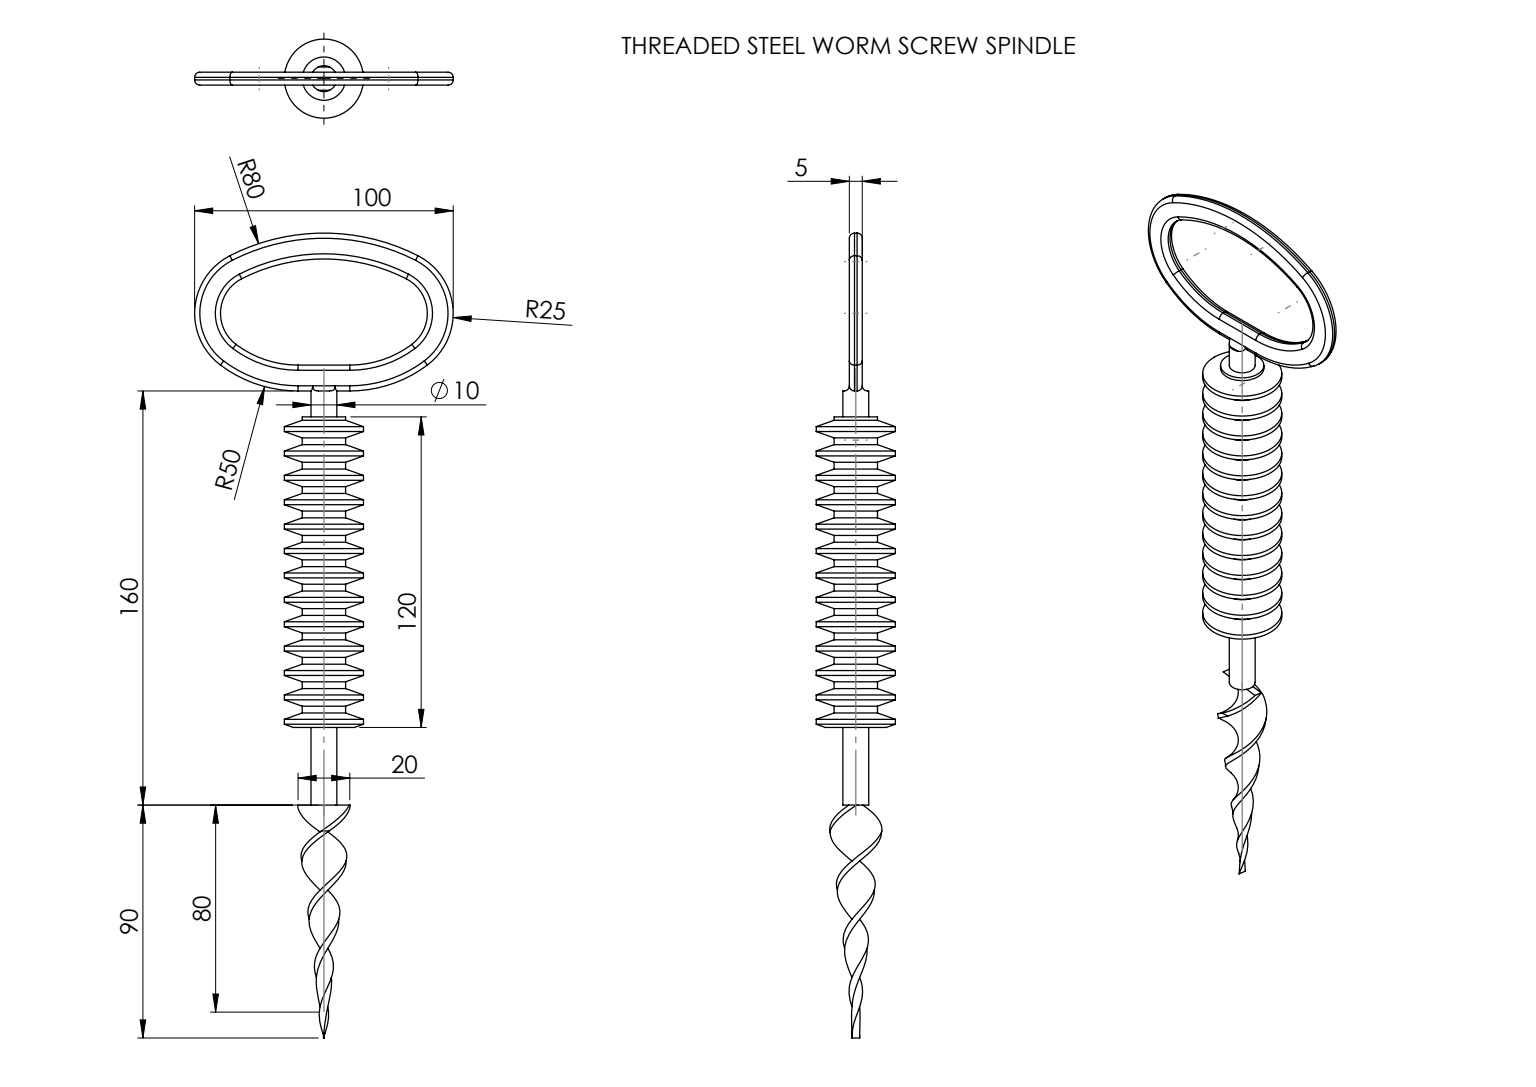
ISO-10303-21;
HEADER;
FILE_DESCRIPTION (('STEP AP214'),
    '1' );
FILE_NAME ('Threaded Steel Worm Screw Spindle.step',
    '2026-10-08T14:03:35',
    ( '' ),
    ( '' ),
    'SwSTEP 2.0',
    'SolidWorks 2026',
    '' );
FILE_SCHEMA (( 'AUTOMOTIVE_DESIGN' ));
ENDSEC;

DATA;
#7=AXIS2_PLACEMENT_3D ( 'NONE', #7492, #359, #1391 ) ;
#9=ORIENTED_EDGE ( 'NONE', *, *, #2863, .F. ) ;
#10=CYLINDRICAL_SURFACE ( 'NONE', #6059, 5.000000000000000000 ) ;
#12=DIRECTION ( 'NONE',  ( -1.000000000000000000, 0.000000000000000000, 0.000000000000000000 ) ) ;
#16=CARTESIAN_POINT ( 'NONE',  ( -12.99553232110413248, 67.62342244460847951, -25.99106464220826851 ) ) ;
#19=CARTESIAN_POINT ( 'NONE',  ( 4.330127018922190985, 92.00000000000000000, -2.500000000000000000 ) ) ;
#20=CARTESIAN_POINT ( 'NONE',  ( 10.69381717166375623, 25.55944687211528077, 0.000000000000000000 ) ) ;
#21=ADVANCED_FACE ( 'NONE', ( #11217 ), #12542, .T. ) ;
#26=EDGE_CURVE ( 'NONE', #11146, #5183, #4908, .T. ) ;
#27=EDGE_CURVE ( 'NONE', #5877, #10681, #5933, .T. ) ;
#30=VERTEX_POINT ( 'NONE', #13473 ) ;
#31=CARTESIAN_POINT ( 'NONE',  ( 25.00000000000000355, 120.0000000000000284, -0.5000000000000000000 ) ) ;
#32=CARTESIAN_POINT ( 'NONE',  ( 8.259026987433399469, -87.08508809531834061, -4.189641850005036083 ) ) ;
#36=CARTESIAN_POINT ( 'NONE',  ( -12.99579180576517246, 64.08350967699263379, -3.310582014804570635E-15 ) ) ;
#37=DIRECTION ( 'NONE',  ( -2.797435172181481150E-17, 1.000000000000000000, -1.765856845898762549E-18 ) ) ;
#38=CARTESIAN_POINT ( 'NONE',  ( -4.250272934615508369, -76.81818181818270830, -9.136824450690360422 ) ) ;
#41=B_SPLINE_CURVE_WITH_KNOTS ( 'NONE', 3,
 ( #7096, #11371, #11645, #793, #10657, #9414, #8218, #1840, #4203, #6320, #13730, #12506, #2044, #8486, #3154, #2892, #3943, #7162, #10396, #1973, #13588, #10461, #11447, #12783, #5330, #6125, #4075, #12585, #8357, #859, #3030, #10593, #5066, #6254, #12653, #997, #11713, #7433, #2104, #9347, #5125, #1907, #13657, #4005, #8288, #6388, #5261, #1067, #2965, #7233, #7301, #11516, #11582, #3091, #9550, #6196, #8427, #10523, #931, #13858, #5196, #9484, #13791, #4141, #12715, #7359, #12055, #6584, #8618, #1398, #12856, #9746, #158, #7499, #6454, #13067, #1133, #3221, #9677, #5393, #292, #12926, #10918, #4547, #2170, #6728, #3289, #81, #6655, #1321, #7637, #10717, #10997, #7564, #11781, #2240, #8759, #3423, #4335, #11846, #8825, #2370, #2303, #8688, #6525, #10783, #4276, #9612 ),
 .UNSPECIFIED., .F., .F.,
 ( 4, 2, 2, 2, 2, 2, 2, 2, 2, 2, 2, 2, 2, 2, 2, 2, 2, 2, 2, 2, 2, 2, 2, 2, 2, 2, 2, 2, 2, 2, 2, 2, 2, 2, 2, 2, 2, 2, 2, 2, 2, 2, 2, 2, 2, 2, 2, 2, 2, 2, 2, 2, 2, 4 ),
 ( 1.115175723065530429E-16, 0.0007940898450324740008, 0.001588179690064836329, 0.003176359380129561202, 0.004764539070194286074, 0.006352718760259011381, 0.007940898450323734953, 0.009529078140388459392, 0.01111725783045318383, 0.01270543752051791001, 0.01588179690064744215, 0.01905815628077697083, 0.02223451566090650297, 0.02382269535097126731, 0.02541087504103603512, 0.02858723442116564359, 0.03017541411123044609, 0.03176359380129525206, 0.03493995318142493339, 0.03652813287148980875, 0.03811631256155468411, 0.04129267194168446953, 0.04288085163174937264, 0.04446903132181426188, 0.04764539070194404730, 0.04923357039200896429, 0.05082175008207386740, 0.05399810946220368751, 0.05717446884233351456, 0.05876264853239842462, 0.06035082822246332079, 0.06352718760259316866, 0.06511536729265808565, 0.06670354698272301652, 0.06829172667278794739, 0.06987990636285287827, 0.07305626574298272613, 0.07464444543304765700, 0.07623262512311257399, 0.07782080481317750487, 0.07940898450324243574, 0.08258534388337231136, 0.08417352357343724223, 0.08576170326350217310, 0.08734988295356710397, 0.08893806264363202096, 0.09211442202376185495, 0.09370260171382675807, 0.09529078140389167506, 0.09687896109395660593, 0.09846714078402152293, 0.1000553204740864260, 0.1008494103191188984, 0.1016435001641513708 ),
 .UNSPECIFIED. ) ;
#43=EDGE_CURVE ( 'NONE', #8596, #8398, #2943, .T. ) ;
#46=FACE_OUTER_BOUND ( 'NONE', #6458, .T. ) ;
#49=CARTESIAN_POINT ( 'NONE',  ( 2.406219558548489190E-16, -8.601520358636511432, 1.518905361043589440E-17 ) ) ;
#52=DIRECTION ( 'NONE',  ( -2.797435172181481150E-17, 1.000000000000000000, -1.765856845898762549E-18 ) ) ;
#53=CARTESIAN_POINT ( 'NONE',  ( 1.800977217354326365, -65.63636364725842043, 1.354836293522729163 ) ) ;
#57=CARTESIAN_POINT ( 'NONE',  ( -8.385254915620292238, 24.75422479069652937, -16.77050983124059158 ) ) ;
#58=CARTESIAN_POINT ( 'NONE',  ( -15.29705854078140348, -29.33764382806072746, 30.59411708156278920 ) ) ;
#59=CARTESIAN_POINT ( 'NONE',  ( -2.079471018873752021E-15, 74.33491362204294717, -1.312648161087776599E-16 ) ) ;
#62=EDGE_LOOP ( 'NONE', ( #12490, #5333, #1562, #12326 ) ) ;
#64=CARTESIAN_POINT ( 'NONE',  ( -10.69381717166375800, 53.83378072214353693, -1.499740397452121781E-15 ) ) ;
#70=ORIENTED_EDGE ( 'NONE', *, *, #7148, .F. ) ;
#73=ORIENTED_EDGE ( 'NONE', *, *, #707, .T. ) ;
#78=CARTESIAN_POINT ( 'NONE',  ( 0.3899450390716444614, -79.59552052770862929, -10.11716208056824762 ) ) ;
#79=DIRECTION ( 'NONE',  ( -1.000000000000000000, 0.000000000000000000, 0.000000000000000000 ) ) ;
#80=CARTESIAN_POINT ( 'NONE',  ( 3.915931169992960648, 90.55292468037850995, -3.111431273932147246 ) ) ;
#81=CARTESIAN_POINT ( 'NONE',  ( -7.912770636739809405, -89.29698991853884138, 4.227864033747772865 ) ) ;
#83=EDGE_LOOP ( 'NONE', ( #9533, #5553, #4896, #10180 ) ) ;
#84=ORIENTED_EDGE ( 'NONE', *, *, #10476, .F. ) ;
#93=AXIS2_PLACEMENT_3D ( 'NONE', #1306, #12036, #9868 ) ;
#96=CARTESIAN_POINT ( 'NONE',  ( -2.905947830705728041, -133.0909090909398458, 2.158723819798283206 ) ) ;
#99=EDGE_CURVE ( 'NONE', #9883, #11270, #7176, .T. ) ;
#100=CARTESIAN_POINT ( 'NONE',  ( 1.824130267506742786, -166.5454545852088017, -2.249022964541941061 ) ) ;
#102=CARTESIAN_POINT ( 'NONE',  ( -1.416598489609734557, -78.09090909090909349, -10.12631592825915838 ) ) ;
#103=B_SPLINE_CURVE_WITH_KNOTS ( 'NONE', 3,
 ( #9323, #12223, #13300, #13225 ),
 .UNSPECIFIED., .F., .F.,
 ( 4, 4 ),
 ( 0.000000000000000000, 1.000000000000000000 ),
 .UNSPECIFIED. ) ;
#106=VECTOR ( 'NONE', #4632, 1000.000000000000000 ) ;
#111=CIRCLE ( 'NONE', #7943, 15.29705854078139460 ) ;
#112=ADVANCED_FACE ( 'NONE', ( #12595 ), #4281, .T. ) ;
#114=EDGE_CURVE ( 'NONE', #2716, #3638, #13476, .T. ) ;
#117=AXIS2_PLACEMENT_3D ( 'NONE', #10882, #1230, #12167 ) ;
#118=CARTESIAN_POINT ( 'NONE',  ( 8.385254915620292238, 90.00000000000000000, 8.679704431140114636E-16 ) ) ;
#119=CARTESIAN_POINT ( 'NONE',  ( -15.29705854078139637, 74.33491362204294717, -1.312648161087776599E-16 ) ) ;
#120=CARTESIAN_POINT ( 'NONE',  ( -8.385254915620295790, 3.280056672672170492, 16.77050983124058448 ) ) ;
#125=CARTESIAN_POINT ( 'NONE',  ( -12.99579180576517246, -20.73949187309215247, -1.518279536322449159E-15 ) ) ;
#126=CARTESIAN_POINT ( 'NONE',  ( -8.385254915620294014, 12.70483462268159869, -2.089658196149648066E-15 ) ) ;
#135=ORIENTED_EDGE ( 'NONE', *, *, #9456, .T. ) ;
#143=DIRECTION ( 'NONE',  ( -2.797435172181481150E-17, 1.000000000000000000, -1.765856845898762549E-18 ) ) ;
#145=EDGE_LOOP ( 'NONE', ( #4394, #1634, #10776, #9029 ) ) ;
#146=AXIS2_PLACEMENT_3D ( 'NONE', #3923, #12417, #8205 ) ;
#147=CIRCLE ( 'NONE', #5069, 5.000000000000000000 ) ;
#149=VERTEX_POINT ( 'NONE', #5637 ) ;
#150=CARTESIAN_POINT ( 'NONE',  ( 15.29705854078138927, 55.48535772202409078, 1.773704474924340737E-15 ) ) ;
#151=ORIENTED_EDGE ( 'NONE', *, *, #13444, .T. ) ;
#154=AXIS2_PLACEMENT_3D ( 'NONE', #13891, #2740, #9326 ) ;
#156=DIRECTION ( 'NONE',  ( -2.797435172181481150E-17, 1.000000000000000000, -1.765856845898762549E-18 ) ) ;
#158=CARTESIAN_POINT ( 'NONE',  ( -5.529376117763302290, -98.63915323273988633, -5.578400940830572807 ) ) ;
#159=B_SPLINE_CURVE_WITH_KNOTS ( 'NONE', 3,
 ( #12320, #4952, #9234, #13548 ),
 .UNSPECIFIED., .F., .F.,
 ( 4, 4 ),
 ( 0.000000000000000000, 1.000000000000000000 ),
 .UNSPECIFIED. ) ;
#164=CIRCLE ( 'NONE', #12478, 50.00000000000001421 ) ;
#166=CARTESIAN_POINT ( 'NONE',  ( 31.81818181818183433, 133.3608531424536920, 2.500000000000000000 ) ) ;
#169=CARTESIAN_POINT ( 'NONE',  ( -15.29705854078138927, 19.67281349139174296, -3.473937238186366113E-17 ) ) ;
#173=CARTESIAN_POINT ( 'NONE',  ( -9.456627357064087747, -73.18181818181821541, -3.908318357316046487 ) ) ;
#176=ADVANCED_FACE ( 'NONE', ( #6620 ), #9921, .T. ) ;
#179=ORIENTED_EDGE ( 'NONE', *, *, #7625, .T. ) ;
#180=CARTESIAN_POINT ( 'NONE',  ( -2.517691654963332357E-15, 90.00000000000000000, -1.589271161308885878E-16 ) ) ;
#183=CARTESIAN_POINT ( 'NONE',  ( -12.99579180576516535, 7.534841976936128560, -1.618136388307047266E-15 ) ) ;
#185=CARTESIAN_POINT ( 'NONE',  ( 12.99579180576516713, 73.50828762700209040, 0.000000000000000000 ) ) ;
#188=FACE_OUTER_BOUND ( 'NONE', #11939, .T. ) ;
#190=EDGE_CURVE ( 'NONE', #2348, #11393, #10077, .T. ) ;
#191=DIRECTION ( 'NONE',  ( -2.797435172181481150E-17, 1.000000000000000000, -1.765856845898762549E-18 ) ) ;
#192=ADVANCED_FACE ( 'NONE', ( #6688 ), #1879, .T. ) ;
#193=ADVANCED_FACE ( 'NONE', ( #9782 ), #3762, .T. ) ;
#195=EDGE_LOOP ( 'NONE', ( #3953, #4577 ) ) ;
#198=ADVANCED_FACE ( 'NONE', ( #8588 ), #2424, .T. ) ;
#200=ORIENTED_EDGE ( 'NONE', *, *, #12255, .T. ) ;
#204=FACE_OUTER_BOUND ( 'NONE', #4519, .T. ) ;
#207=EDGE_CURVE ( 'NONE', #13779, #9777, #1115, .T. ) ;
#211=EDGE_CURVE ( 'NONE', #2222, #2825, #5653, .T. ) ;
#213=EDGE_LOOP ( 'NONE', ( #12461, #12603, #11855, #6788 ) ) ;
#215=DIRECTION ( 'NONE',  ( -2.797435172181481150E-17, 1.000000000000000000, -1.765856845898762549E-18 ) ) ;
#217=CARTESIAN_POINT ( 'NONE',  ( -1.868594470333698657E-15, 66.79670324143890525, -1.179534157023628988E-16 ) ) ;
#218=DIRECTION ( 'NONE',  ( -0.000000000000000000, -0.000000000000000000, -1.000000000000000000 ) ) ;
#219=CYLINDRICAL_SURFACE ( 'NONE', #7081, 8.385254915620292238 ) ;
#221=CARTESIAN_POINT ( 'NONE',  ( -15.29705854078139282, -29.33764382806072746, -30.59411708156279630 ) ) ;
#223=EDGE_LOOP ( 'NONE', ( #1388, #322, #1636, #10853 ) ) ;
#226=ORIENTED_EDGE ( 'NONE', *, *, #7270, .T. ) ;
#228=FACE_OUTER_BOUND ( 'NONE', #3050, .T. ) ;
#229=CARTESIAN_POINT ( 'NONE',  ( -0.9875499244693202172, -80.00464164737402939, 10.06307371418729701 ) ) ;
#232=CARTESIAN_POINT ( 'NONE',  ( -25.00000000000000355, 120.0000000000000284, 0.5000000000000000000 ) ) ;
#233=CARTESIAN_POINT ( 'NONE',  ( -15.29705854078139637, 0.8232575913728885642, -1.453755053663958216E-18 ) ) ;
#235=CARTESIAN_POINT ( 'NONE',  ( -2.866821506922881722E-16, 10.24803554138234496, -1.809656371776380929E-17 ) ) ;
#236=CARTESIAN_POINT ( 'NONE',  ( 1.713057075396043238, -163.8787878899150030, 2.641018403436653728 ) ) ;
#237=VECTOR ( 'NONE', #1930, 1000.000000000000000 ) ;
#238=CARTESIAN_POINT ( 'NONE',  ( 15.29705854078138927, 46.06057977201469100, 1.790347283588440388E-15 ) ) ;
#241=FILL_AREA_STYLE ('',( #9833 ) ) ;
#243=CYLINDRICAL_SURFACE ( 'NONE', #12092, 8.385254915620295790 ) ;
#244=CARTESIAN_POINT ( 'NONE',  ( 0.4999999999999966693, 79.99058638175036151, -2.499999999999982236 ) ) ;
#246=ORIENTED_EDGE ( 'NONE', *, *, #1045, .F. ) ;
#247=CIRCLE ( 'NONE', #2028, 15.29705854078138572 ) ;
#248=AXIS2_PLACEMENT_3D ( 'NONE', #3744, #8028, #12308 ) ;
#250=CARTESIAN_POINT ( 'NONE',  ( 36.36363636363638108, 142.2680885707561629, 2.500000000000000000 ) ) ;
#251=ORIENTED_EDGE ( 'NONE', *, *, #10047, .F. ) ;
#252=DIRECTION ( 'NONE',  ( -2.797435172181481150E-17, 1.000000000000000000, -1.765856845898762549E-18 ) ) ;
#255=EDGE_CURVE ( 'NONE', #10763, #2744, #8961, .T. ) ;
#258=AXIS2_PLACEMENT_3D ( 'NONE', #3303, #12076, #6668 ) ;
#259=CARTESIAN_POINT ( 'NONE',  ( -12.99579180576516713, -1.889935973073298525, -1.584850770978847568E-15 ) ) ;
#262=DIRECTION ( 'NONE',  ( -1.000000000000000000, -5.171946152600902986E-17, 0.000000000000000000 ) ) ;
#263=AXIS2_PLACEMENT_3D ( 'NONE', #6259, #865, #11653 ) ;
#264=B_SPLINE_CURVE_WITH_KNOTS ( 'NONE', 3,
 ( #3142, #782, #3995, #11363 ),
 .UNSPECIFIED., .F., .F.,
 ( 4, 4 ),
 ( 0.000000000000000000, 1.000000000000000000 ),
 .UNSPECIFIED. ) ;
#267=LINE ( 'NONE', #5318, #5455 ) ;
#268=CIRCLE ( 'NONE', #8110, 14.99999999999998934 ) ;
#271=EDGE_CURVE ( 'NONE', #8931, #12042, #8495, .T. ) ;
#274=CARTESIAN_POINT ( 'NONE',  ( -12.99553232110413781, 39.34908859458022334, -1.730463420974848368E-15 ) ) ;
#275=EDGE_CURVE ( 'NONE', #4145, #2418, #159, .T. ) ;
#278=CARTESIAN_POINT ( 'NONE',  ( 10.69346802281034492, 11.89973432371241380, 2.619144277183853160E-15 ) ) ;
#282=CARTESIAN_POINT ( 'NONE',  ( -25.00000000000000355, 120.0000000000000284, -0.5000000000000000000 ) ) ;
#283=VERTEX_POINT ( 'NONE', #6077 ) ;
#284=CARTESIAN_POINT ( 'NONE',  ( -15.29705854078138394, 76.22148119144830503, -30.59411708156277854 ) ) ;
#285=ORIENTED_EDGE ( 'NONE', *, *, #8017, .F. ) ;
#286=DIRECTION ( 'NONE',  ( 0.1234677578012386701, 0.000000000000000000, -0.9923485843107424653 ) ) ;
#287=CARTESIAN_POINT ( 'NONE',  ( 5.570495138619319060E-16, -19.91286587805129926, 3.516327053222078456E-17 ) ) ;
#291=CARTESIAN_POINT ( 'NONE',  ( 4.317896099768522511, 91.66241202089436513, -2.521541801375117853 ) ) ;
#292=CARTESIAN_POINT ( 'NONE',  ( -8.281054986618348934, -94.04345070189340561, -1.330912282001587954 ) ) ;
#293=CARTESIAN_POINT ( 'NONE',  ( -15.29705854078139282, 90.00000000000000000, -1.589271161308885878E-16 ) ) ;
#295=CIRCLE ( 'NONE', #9689, 77.99999999999997158 ) ;
#296=EDGE_LOOP ( 'NONE', ( #12676, #4447, #755, #3036 ) ) ;
#297=VERTEX_POINT ( 'NONE', #11394 ) ;
#299=CARTESIAN_POINT ( 'NONE',  ( -7.887411832334696449, -93.14649341443603703, -3.265743713357469602 ) ) ;
#300=CARTESIAN_POINT ( 'NONE',  ( -3.915931169992964200, 90.55292468037848153, 3.111431273932144581 ) ) ;
#302=LINE ( 'NONE', #4555, #8293 ) ;
#304=CARTESIAN_POINT ( 'NONE',  ( -12.99579180576516713, -1.889935973073298525, -1.584850770978847568E-15 ) ) ;
#305=CARTESIAN_POINT ( 'NONE',  ( -12.99579180576516713, 35.80917582696438473, -1.717993240291646161E-15 ) ) ;
#306=CARTESIAN_POINT ( 'NONE',  ( 15.29705854078139460, -8.601520358636511432, 1.890204135573040269E-15 ) ) ;
#307=CARTESIAN_POINT ( 'NONE',  ( 25.00000000000000355, 120.0000000000000284, 0.5000000000000000000 ) ) ;
#308=CARTESIAN_POINT ( 'NONE',  ( -10.11144051725924520, -69.99977036137985920, 0.2534939247371171822 ) ) ;
#310=CARTESIAN_POINT ( 'NONE',  ( -2.517691654963332357E-15, 90.00000000000000000, -1.589271161308885878E-16 ) ) ;
#311=CARTESIAN_POINT ( 'NONE',  ( -15.29705854078139460, -18.02629830864593785, -1.809685653284690613E-15 ) ) ;
#312=DIRECTION ( 'NONE',  ( -2.797435172181481150E-17, 1.000000000000000000, -1.765856845898762549E-18 ) ) ;
#313=VECTOR ( 'NONE', #2315, 1000.000000000000000 ) ;
#318=CARTESIAN_POINT ( 'NONE',  ( -15.29705854078138927, 74.33491362204296138, -30.59411708156278564 ) ) ;
#320=CARTESIAN_POINT ( 'NONE',  ( -4.288313376222440694E-16, 15.32944684068712782, -2.706960864746847057E-17 ) ) ;
#322=ORIENTED_EDGE ( 'NONE', *, *, #4730, .F. ) ;
#323=CARTESIAN_POINT ( 'NONE',  ( 35.45454545454547457, 140.4866414850956744, -0.5000000000000000000 ) ) ;
#326=CARTESIAN_POINT ( 'NONE',  ( -15.29705854078139460, 27.21102387199583461, 30.59411708156277854 ) ) ;
#329=CARTESIAN_POINT ( 'NONE',  ( -25.00000000000000355, 120.0000000000000284, -0.5000000000000000000 ) ) ;
#334=DIRECTION ( 'NONE',  ( -0.000000000000000000, -0.000000000000000000, -1.000000000000000000 ) ) ;
#336=ORIENTED_EDGE ( 'NONE', *, *, #5229, .T. ) ;
#337=FACE_OUTER_BOUND ( 'NONE', #1428, .T. ) ;
#338=ORIENTED_EDGE ( 'NONE', *, *, #5869, .F. ) ;
#341=DIRECTION ( 'NONE',  ( 1.000000000000000000, 0.000000000000000000, 0.000000000000000000 ) ) ;
#346=CARTESIAN_POINT ( 'NONE',  ( 1.119237408740483668E-15, -40.00941361824963849, 7.065089693818137167E-17 ) ) ;
#349=DIRECTION ( 'NONE',  ( -0.1234677578008764876, 2.460994371251751031E-11, 0.9923485843107875404 ) ) ;
#350=AXIS2_PLACEMENT_3D ( 'NONE', #10266, #11321, #5862 ) ;
#354=EDGE_CURVE ( 'NONE', #717, #1714, #10955, .T. ) ;
#356=CARTESIAN_POINT ( 'NONE',  ( 8.385254915620295790, -24.99427717735608212, 1.068716529980328740E-15 ) ) ;
#357=VERTEX_POINT ( 'NONE', #882 ) ;
#359=DIRECTION ( 'NONE',  ( -2.797435172181481150E-17, 1.000000000000000000, -1.765856845898762549E-18 ) ) ;
#366=CARTESIAN_POINT ( 'NONE',  ( 15.29705854078138749, 57.37192529142945574, 3.746698755667522411E-15 ) ) ;
#367=ORIENTED_EDGE ( 'NONE', *, *, #12940, .T. ) ;
#368=EDGE_CURVE ( 'NONE', #4551, #8182, #6045, .T. ) ;
#371=CARTESIAN_POINT ( 'NONE',  ( -7.177581306179082077, -94.18858243930635865, -4.303391048795623064 ) ) ;
#372=DIRECTION ( 'NONE',  ( -1.000000000000000000, 0.000000000000000000, 0.000000000000000000 ) ) ;
#374=( BOUNDED_SURFACE ( )  B_SPLINE_SURFACE ( 3, 3, ( 
 ( #3071, #10573, #976, #9525 ),
 ( #7481, #12037, #5514, #9661 ),
 ( #6639, #11762, #5441, #8537 ),
 ( #7615, #5310, #2217, #8808 ) ),
 .UNSPECIFIED., .F., .F., .F. ) 
 B_SPLINE_SURFACE_WITH_KNOTS ( ( 4, 4 ),
 ( 4, 4 ),
 ( 0.000000000000000000, 1.000000000000000000 ),
 ( 0.000000000000000000, 1.000000000000000000 ),
 .UNSPECIFIED. ) 
 GEOMETRIC_REPRESENTATION_ITEM ( )  RATIONAL_B_SPLINE_SURFACE ( (
 ( 1.000000000000000000, 0.3333333333333334259, 0.3333333333333334259, 1.000000000000000000),
 ( 1.000000000000000000, 0.3333333333333334259, 0.3333333333333334259, 1.000000000000000000),
 ( 1.000000000000000000, 0.3333333333333334259, 0.3333333333333334259, 1.000000000000000000),
 ( 1.000000000000000000, 0.3333333333333334259, 0.3333333333333334259, 1.000000000000000000) ) ) 
 REPRESENTATION_ITEM ( '' )  SURFACE ( )  );
#375=EDGE_CURVE ( 'NONE', #7425, #1069, #7596, .T. ) ;
#380=DIRECTION ( 'NONE',  ( -2.797435172181481150E-17, 1.000000000000000000, -1.765856845898762549E-18 ) ) ;
#382=DIRECTION ( 'NONE',  ( 1.000000000000000000, 0.000000000000000000, 0.000000000000000000 ) ) ;
#383=CARTESIAN_POINT ( 'NONE',  ( 8.385254915620292238, 59.82872437272870769, -16.77050983124058092 ) ) ;
#384=LINE ( 'NONE', #7781, #5223 ) ;
#385=CARTESIAN_POINT ( 'NONE',  ( -2.134167523385911647, -102.5454545454534099, -7.554873526040499776 ) ) ;
#386=CARTESIAN_POINT ( 'NONE',  ( -15.29705854078139282, 46.06057977201469100, -8.133639011647813827E-17 ) ) ;
#387=CARTESIAN_POINT ( 'NONE',  ( 15.29705854078139815, -18.02629830864593785, -30.59411708156277854 ) ) ;
#388=CARTESIAN_POINT ( 'NONE',  ( 7.181435285653160250, -97.41991341991979425, 5.065585088379008560 ) ) ;
#392=EDGE_LOOP ( 'NONE', ( #9098, #8342, #7823, #504 ) ) ;
#394=AXIS2_PLACEMENT_3D ( 'NONE', #10889, #13103, #12895 ) ;
#395=ORIENTED_EDGE ( 'NONE', *, *, #12190, .T. ) ;
#398=CARTESIAN_POINT ( 'NONE',  ( 15.29705854078139815, 0.8232575913728894523, 1.873561326908940224E-15 ) ) ;
#401=DIRECTION ( 'NONE',  ( 1.000000000000000000, 0.000000000000000000, 0.000000000000000000 ) ) ;
#402=CARTESIAN_POINT ( 'NONE',  ( 1.947606478028208261E-13, -70.00000000000000000, 2.411204079342396664E-14 ) ) ;
#405=DIRECTION ( 'NONE',  ( -1.000000000000000000, 0.000000000000000000, 0.000000000000000000 ) ) ;
#407=B_SPLINE_CURVE_WITH_KNOTS ( 'NONE', 3,
 ( #6684, #183, #7665, #5554 ),
 .UNSPECIFIED., .F., .F.,
 ( 4, 4 ),
 ( 0.000000000000000000, 1.000000000000000000 ),
 .UNSPECIFIED. ) ;
#408=FACE_OUTER_BOUND ( 'NONE', #9520, .T. ) ;
#409=LINE ( 'NONE', #6624, #13262 ) ;
#413=CYLINDRICAL_SURFACE ( 'NONE', #5659, 8.385254915620292238 ) ;
#415=EDGE_LOOP ( 'NONE', ( #5034, #4687, #8692, #5104 ) ) ;
#416=CARTESIAN_POINT ( 'NONE',  ( -25.00000000000000355, 120.0000000000000284, -2.500000000000000000 ) ) ;
#417=EDGE_LOOP ( 'NONE', ( #8624, #1326, #7821, #12079 ) ) ;
#423=CARTESIAN_POINT ( 'NONE',  ( -8.385254915620299343, -34.41905512736551032, 16.77050983124059513 ) ) ;
#424=CARTESIAN_POINT ( 'NONE',  ( -11.81226048336476708, -40.00941361824963849, -1.520867253700650540E-15 ) ) ;
#428=CIRCLE ( 'NONE', #8039, 2.000000000000003997 ) ;
#430=VERTEX_POINT ( 'NONE', #6149 ) ;
#431=ORIENTED_EDGE ( 'NONE', *, *, #8075, .F. ) ;
#437=CARTESIAN_POINT ( 'NONE',  ( 2.498436201158980463, -101.8697035856479260, 6.998341292597221930 ) ) ;
#438=CARTESIAN_POINT ( 'NONE',  ( 15.29705854078138927, 17.78624592198638155, -30.59411708156276788 ) ) ;
#440=ORIENTED_EDGE ( 'NONE', *, *, #1952, .T. ) ;
#441=ORIENTED_EDGE ( 'NONE', *, *, #13836, .T. ) ;
#443=CARTESIAN_POINT ( 'NONE',  ( 12.99553232110414669, -26.62435705548577047, 3.182987412051232956E-15 ) ) ;
#444=CARTESIAN_POINT ( 'NONE',  ( 2.563982627555995819, -78.09090909091013089, 9.749794964675599473 ) ) ;
#446=CARTESIAN_POINT ( 'NONE',  ( -0.9875499244693202172, -80.00464164737402939, 10.06307371418729701 ) ) ;
#449=DIRECTION ( 'NONE',  ( -2.797435172181481150E-17, 1.000000000000000000, -1.765856845898762549E-18 ) ) ;
#451=CARTESIAN_POINT ( 'NONE',  ( -2.054569550994074234, -122.9090909090864159, -4.917417506340981959 ) ) ;
#455=DIRECTION ( 'NONE',  ( -0.8907235428302473501, -0.4545454545454531425, -0.000000000000000000 ) ) ;
#459=ORIENTED_EDGE ( 'NONE', *, *, #3702, .T. ) ;
#461=AXIS2_PLACEMENT_3D ( 'NONE', #7793, #1638, #3808 ) ;
#462=CARTESIAN_POINT ( 'NONE',  ( -4.974937185533102380, 90.00000000000000000, 0.5000000000000000000 ) ) ;
#464=CARTESIAN_POINT ( 'NONE',  ( -2.127113563276592512, -126.4347724850053396, 3.943208343314429154 ) ) ;
#471=CARTESIAN_POINT ( 'NONE',  ( -1.823748309627396313, -150.1894710958037251, 0.6860160126068575170 ) ) ;
#474=CARTESIAN_POINT ( 'NONE',  ( 15.29705854078139282, 46.06057977201469100, -30.59411708156277854 ) ) ;
#475=CARTESIAN_POINT ( 'NONE',  ( -2.517691654963332357E-15, 90.00000000000000000, -1.589271161308885878E-16 ) ) ;
#476=CARTESIAN_POINT ( 'NONE',  ( -15.29705854078139105, 8.361467971976981772, -1.476515546007874940E-17 ) ) ;
#477=CARTESIAN_POINT ( 'NONE',  ( 34.00000000000001421, 108.0000000000000142, 0.5000000000000000000 ) ) ;
#481=CARTESIAN_POINT ( 'NONE',  ( -10.69346802281034670, -35.22415542633469698, -1.185170506590736236E-15 ) ) ;
#482=CIRCLE ( 'NONE', #702, 8.385254915620295790 ) ;
#483=CARTESIAN_POINT ( 'NONE',  ( 8.385254915620288685, 15.32944684068712782, 16.77050983124058448 ) ) ;
#484=AXIS2_PLACEMENT_3D ( 'NONE', #235, #2386, #11795 ) ;
#486=CARTESIAN_POINT ( 'NONE',  ( 4.268720428656451737, 91.34229515271626099, 2.603909174561179540 ) ) ;
#487=ORIENTED_EDGE ( 'NONE', *, *, #12528, .F. ) ;
#488=CARTESIAN_POINT ( 'NONE',  ( -4.607646589138113313, -134.6363636363689977, -0.3820433400546732750 ) ) ;
#489=EDGE_LOOP ( 'NONE', ( #11904, #251, #1201, #2372 ) ) ;
#491=AXIS2_PLACEMENT_3D ( 'NONE', #12908, #6506, #11038 ) ;
#494=( BOUNDED_SURFACE ( )  B_SPLINE_SURFACE ( 3, 3, ( 
 ( #12028, #7814, #12101, #1510 ),
 ( #10005, #4668, #11125, #3609 ),
 ( #6845, #5793, #8499, #5617 ),
 ( #306, #10669, #3167, #13002 ) ),
 .UNSPECIFIED., .F., .F., .T. ) 
 B_SPLINE_SURFACE_WITH_KNOTS ( ( 4, 4 ),
 ( 4, 4 ),
 ( 0.000000000000000000, 1.000000000000000000 ),
 ( 0.000000000000000000, 1.000000000000000000 ),
 .UNSPECIFIED. ) 
 GEOMETRIC_REPRESENTATION_ITEM ( )  RATIONAL_B_SPLINE_SURFACE ( (
 ( 1.000000000000000000, 0.3333333333333334259, 0.3333333333333334259, 1.000000000000000000),
 ( 1.000000000000000000, 0.3333333333333334259, 0.3333333333333334259, 1.000000000000000000),
 ( 1.000000000000000000, 0.3333333333333334259, 0.3333333333333334259, 1.000000000000000000),
 ( 1.000000000000000000, 0.3333333333333334259, 0.3333333333333334259, 1.000000000000000000) ) ) 
 REPRESENTATION_ITEM ( '' )  SURFACE ( )  );
#495=CARTESIAN_POINT ( 'NONE',  ( 6.356408395747725315, -164.3636363623434704, 0.5463072363203682613 ) ) ;
#498=CARTESIAN_POINT ( 'NONE',  ( -15.29705854078139105, 8.361467971976955127, -1.902879688753918396E-15 ) ) ;
#500=ADVANCED_FACE ( 'NONE', ( #7521 ), #3866, .T. ) ;
#501=CARTESIAN_POINT ( 'NONE',  ( 15.29705854078138927, 19.67281349139177138, 3.746698755667522411E-15 ) ) ;
#502=CARTESIAN_POINT ( 'NONE',  ( 9.943536536256114999, -71.42980831100965133, 1.832023074086042591 ) ) ;
#503=ADVANCED_FACE ( 'NONE', ( #5628, #46 ), #2266, .T. ) ;
#504=ORIENTED_EDGE ( 'NONE', *, *, #7116, .F. ) ;
#506=DIRECTION ( 'NONE',  ( -0.000000000000000000, -0.000000000000000000, -1.000000000000000000 ) ) ;
#511=AXIS2_PLACEMENT_3D ( 'NONE', #4639, #8923, #13227 ) ;
#513=CARTESIAN_POINT ( 'NONE',  ( 6.374040420648922733, -86.95534703849641289, -6.729367440589365756 ) ) ;
#514=CARTESIAN_POINT ( 'NONE',  ( -12.99553232110414136, 58.19864449459907974, -1.797034655631248355E-15 ) ) ;
#515=ORIENTED_EDGE ( 'NONE', *, *, #7707, .T. ) ;
#518=CARTESIAN_POINT ( 'NONE',  ( 6.257768754720297677E-16, -22.36966495935058319, 3.950162600893091522E-17 ) ) ;
#519=B_SPLINE_SURFACE_WITH_KNOTS ( 'NONE', 3, 3, ( 
 ( #5541, #1213, #3438, #3236 ),
 ( #3372, #6601, #1154, #100 ),
 ( #236, #4497, #2388, #13153 ),
 ( #4353, #8636, #3301, #6541 ),
 ( #1337, #5620, #7580, #11861 ),
 ( #10799, #5478, #13452, #3655 ),
 ( #6953, #655, #9134, #5764 ),
 ( #7867, #2753, #3733, #4922 ),
 ( #12226, #3577, #13527, #5692 ),
 ( #3799, #7024, #12429, #3867 ),
 ( #10045, #12368, #1699, #12149 ),
 ( #11301, #9205, #451, #11167 ),
 ( #4790, #10184, #8150, #4713 ),
 ( #8016, #5841, #5987, #2820 ),
 ( #8086, #12293, #10119, #8924 ),
 ( #9066, #1553, #10252, #11015 ),
 ( #1415, #11241, #9978, #388 ),
 ( #1627, #528, #2683, #4640 ),
 ( #13228, #2541, #6817, #11092 ),
 ( #1486, #8999, #13303, #7941 ),
 ( #2615, #6888, #13384, #5911 ),
 ( #594, #4858, #11641, #5193 ),
 ( #8216, #4199, #2962, #1762 ),
 ( #2039, #12712, #6317, #1970 ) ),
 .UNSPECIFIED., .F., .F., .F.,
 ( 4, 1, 1, 1, 1, 1, 1, 1, 1, 1, 1, 1, 1, 1, 1, 1, 1, 1, 1, 1, 1, 4 ),
 ( 4, 4 ),
 ( -0.1668267180224854429, -0.1624291228870498593, -0.1587644602741868916, -0.1580315277516142758, -0.1536339326161787200, -0.1471422445591071271, -0.1404411472098719693, -0.1360435520744364135, -0.1316459569390008300, -0.1272483618035652464, -0.1228507666681296628, -0.1140555763972585096, -0.1096579812618229399, -0.1052603861263873564, -0.1008627909909517867, -0.09646519585551620313, -0.08976409850628105924, -0.08327241044920946633, -0.07887481531377389665, -0.07814188279120132252, -0.07447722017833831309, -0.07007962504290274341 ),
 ( 0.003200000000000001888, 0.006800000000000002223 ),
 .UNSPECIFIED. ) ;
#522=CARTESIAN_POINT ( 'NONE',  ( -0.2899689842973289244, -81.00000000000004263, 10.01379011345948378 ) ) ;
#523=ORIENTED_EDGE ( 'NONE', *, *, #13758, .T. ) ;
#525=LINE ( 'NONE', #10042, #3224 ) ;
#527=CARTESIAN_POINT ( 'NONE',  ( -4.918402716924988205, -70.00000000000000000, 0.8996192050778424321 ) ) ;
#528=CARTESIAN_POINT ( 'NONE',  ( 9.844122869699651446, -91.60173160172368512, 1.011447867174433579 ) ) ;
#529=DIRECTION ( 'NONE',  ( -2.797435172181481150E-17, 1.000000000000000000, -1.765856845898762549E-18 ) ) ;
#531=FACE_OUTER_BOUND ( 'NONE', #4485, .T. ) ;
#532=ORIENTED_EDGE ( 'NONE', *, *, #6100, .T. ) ;
#538=CARTESIAN_POINT ( 'NONE',  ( 6.100791518294768956, -112.6832912522008030, 0.2938029233185053268 ) ) ;
#539=FACE_OUTER_BOUND ( 'NONE', #7622, .T. ) ;
#541=CARTESIAN_POINT ( 'NONE',  ( -10.69346802281034847, 30.74929022373126841, -1.418169827888134119E-15 ) ) ;
#542=DIRECTION ( 'NONE',  ( -1.000000000000000000, 0.000000000000000000, 0.000000000000000000 ) ) ;
#546=CARTESIAN_POINT ( 'NONE',  ( -0.1618148777053960430, -158.9590251630839646, -1.491571185530413901 ) ) ;
#547=CARTESIAN_POINT ( 'NONE',  ( 4.804060984082277663, 90.20500167315060480, -1.391503737930617213 ) ) ;
#549=CARTESIAN_POINT ( 'NONE',  ( 8.385254915620294014, 22.12961257269105531, -16.77050983124058092 ) ) ;
#553=CARTESIAN_POINT ( 'NONE',  ( -12.99579180576517601, 64.08350967699263379, 25.99158361153033070 ) ) ;
#554=DIRECTION ( 'NONE',  ( -2.797435172181481150E-17, 1.000000000000000000, -1.765856845898762549E-18 ) ) ;
#555=CARTESIAN_POINT ( 'NONE',  ( -13.62402331790689836, -89.44155844156966850, 2.236035847434436619 ) ) ;
#558=AXIS2_PLACEMENT_3D ( 'NONE', #878, #13613, #12600 ) ;
#559=CARTESIAN_POINT ( 'NONE',  ( -9.701113296676140862, -68.99999999999997158, -3.021359762293432283 ) ) ;
#561=DIRECTION ( 'NONE',  ( -1.000000000000000000, 0.000000000000000000, 0.000000000000000000 ) ) ;
#562=B_SPLINE_CURVE_WITH_KNOTS ( 'NONE', 3,
 ( #7847, #8980, #2601, #8064, #5745, #4693, #3713, #8001, #12352, #6877, #8206, #9051, #6036, #1537, #2741, #513, #4846, #3785, #7009, #3636, #1686, #13571, #3924, #11152, #11223, #11290, #2873, #5822, #12276, #12488, #5899, #7927, #7147, #11425, #10101, #1614, #5971, #10026, #4774, #2664, #437, #10172, #13509, #13287, #3851, #12210, #13365, #10239, #643, #9121, #6933, #583, #13437, #4907, #9185, #8134, #12418, #2807, #7079, #10311, #11357, #1749, #712, #4976, #9255, #4123, #10374, #4184, #8340, #2088, #8538, #1820, #10575, #9592, #10504, #12564, #7418, #8405, #1932, #9327, #3007, #13642, #2947, #5244, #7214, #5046, #1886, #11496, #6369, #977, #11564, #4255, #6237, #1051, #6175, #11695, #12840, #10443, #1955, #3988, #9466, #13713, #8270, #12634, #9531, #13841, #843, #4059 ),
 .UNSPECIFIED., .F., .F.,
 ( 4, 2, 2, 2, 2, 2, 2, 2, 2, 2, 2, 2, 2, 2, 2, 2, 2, 2, 2, 2, 2, 2, 2, 2, 2, 2, 2, 2, 2, 2, 2, 2, 2, 2, 2, 2, 2, 2, 2, 2, 2, 2, 2, 2, 2, 2, 2, 2, 2, 2, 2, 2, 2, 4 ),
 ( 8.420559318810145779E-18, 0.0007945603842730117761, 0.001589120768546015095, 0.003178241537091996798, 0.004767362305637979150, 0.006356483074183960635, 0.009534724611275923606, 0.01112384537982191897, 0.01271296614836791260, 0.01430208691691390623, 0.01589120768545989465, 0.01906944922255190966, 0.02065856999109790329, 0.02224769075964389692, 0.02383681152818988708, 0.02542593229673587724, 0.02860417383382784021, 0.03019329460237380608, 0.03178241537091977542, 0.03337153613946574476, 0.03496065690801170717, 0.03813889844510363891, 0.03972801921364962213, 0.04131713998219560535, 0.04449538151928759955, 0.04767362305637958680, 0.04926274382492558390, 0.05085186459347158100, 0.05403010613056356826, 0.05561922689910957923, 0.05720834766765561102, 0.05879746843620162200, 0.06038658920474763991, 0.06356483074183967574, 0.06515395151038569366, 0.06674307227893173933, 0.06992131381602378903, 0.07309955535311585262, 0.07468867612166184278, 0.07627779689020783294, 0.07945603842729982713, 0.08104515919584577566, 0.08263427996439172418, 0.08581252150148363511, 0.08899076303857555992, 0.09057988380712146681, 0.09216900457566738758, 0.09375812534421329447, 0.09534724611275921524, 0.09693636688130513601, 0.09852548764985105678, 0.1001146084183969637, 0.1009091688026699241, 0.1017037291869428844 ),
 .UNSPECIFIED. ) ;
#563=CARTESIAN_POINT ( 'NONE',  ( 13.62402331790597287, -89.44155844157094748, -2.236035847433821555 ) ) ;
#564=CARTESIAN_POINT ( 'NONE',  ( 10.69381717166375090, 6.709890972096426154, 21.38763434332751245 ) ) ;
#565=CARTESIAN_POINT ( 'NONE',  ( -12.99579180576517246, -20.73949187309215247, -1.518279536322449159E-15 ) ) ;
#570=ORIENTED_EDGE ( 'NONE', *, *, #12778, .T. ) ;
#571=EDGE_CURVE ( 'NONE', #1705, #2048, #9846, .T. ) ;
#572=CARTESIAN_POINT ( 'NONE',  ( 10.69346802281034670, 30.74929022373126841, 0.000000000000000000 ) ) ;
#575=VERTEX_POINT ( 'NONE', #2474 ) ;
#580=AXIS2_PLACEMENT_3D ( 'NONE', #9356, #5931, #7955 ) ;
#582=DIRECTION ( 'NONE',  ( -1.000000000000000000, -0.000000000000000000, -0.000000000000000000 ) ) ;
#583=CARTESIAN_POINT ( 'NONE',  ( -5.285683233297803874, -111.9165838417090271, 3.246843445714708398 ) ) ;
#584=CARTESIAN_POINT ( 'NONE',  ( 10.69346802281034670, 49.59884612375012125, 1.251549203118916541E-15 ) ) ;
#585=AXIS2_PLACEMENT_3D ( 'NONE', #8584, #7391, #10614 ) ;
#588=CARTESIAN_POINT ( 'NONE',  ( 0.9402774206043281735, -80.12121212121192571, 9.996606859377758170 ) ) ;
#589=ORIENTED_EDGE ( 'NONE', *, *, #13115, .F. ) ;
#590=CARTESIAN_POINT ( 'NONE',  ( 0.2039588443089787317, -79.18543989864099331, 10.12004280280962831 ) ) ;
#594=CARTESIAN_POINT ( 'NONE',  ( -7.328281204033265439, -76.12121212249812174, -4.753922619039316011 ) ) ;
#601=ORIENTED_EDGE ( 'NONE', *, *, #5658, .F. ) ;
#603=CARTESIAN_POINT ( 'NONE',  ( -1.619020611652117081, -125.5321122364420603, 4.300443607797105550 ) ) ;
#606=CARTESIAN_POINT ( 'NONE',  ( -1.604942417060130136E-15, 57.37192529142945574, -1.013106070382630377E-16 ) ) ;
#610=FACE_OUTER_BOUND ( 'NONE', #6249, .T. ) ;
#611=CARTESIAN_POINT ( 'NONE',  ( 4.942648287111185645, 90.01344868170882307, -0.7664870281642336414 ) ) ;
#612=DIRECTION ( 'NONE',  ( -2.797435172181481150E-17, 1.000000000000000000, -1.765856845898762549E-18 ) ) ;
#616=LINE ( 'NONE', #8236, #7848 ) ;
#619=CARTESIAN_POINT ( 'NONE',  ( 4.231485814931493117, 91.18833760977217651, 2.665113332093635101 ) ) ;
#620=ORIENTED_EDGE ( 'NONE', *, *, #5753, .T. ) ;
#621=CARTESIAN_POINT ( 'NONE',  ( -3.373786045844842096, -82.89610389617892849, 3.887588323745183150 ) ) ;
#622=ORIENTED_EDGE ( 'NONE', *, *, #7115, .F. ) ;
#627=CARTESIAN_POINT ( 'NONE',  ( -5.581994045268341864, -105.1818181818167091, 11.80851735648757739 ) ) ;
#631=ADVANCED_FACE ( 'NONE', ( #539 ), #4652, .T. ) ;
#632=EDGE_CURVE ( 'NONE', #3638, #2716, #12550, .T. ) ;
#633=CARTESIAN_POINT ( 'NONE',  ( 8.385254915620294014, 90.00000000000000000, 8.679704431140118580E-16 ) ) ;
#634=CYLINDRICAL_SURFACE ( 'NONE', #4434, 15.29705854078138749 ) ;
#636=EDGE_CURVE ( 'NONE', #4358, #10177, #6755, .T. ) ;
#641=CARTESIAN_POINT ( 'NONE',  ( -8.862685976966703905, -71.63821982307230485, -4.927609701037551027 ) ) ;
#643=CARTESIAN_POINT ( 'NONE',  ( -3.419709198711867071, -108.3206314215273665, 5.719072246552273420 ) ) ;
#644=CARTESIAN_POINT ( 'NONE',  ( -15.29705854078138927, 17.78624592198638155, -3.776441015662857042E-15 ) ) ;
#645=CIRCLE ( 'NONE', #8252, 15.29705854078139993 ) ;
#647=ORIENTED_EDGE ( 'NONE', *, *, #9006, .T. ) ;
#649=DIRECTION ( 'NONE',  ( -1.000000000000000000, -0.000000000000000000, -0.000000000000000000 ) ) ;
#651=CARTESIAN_POINT ( 'NONE',  ( 9.991007172155546456, -71.90909090909001122, 2.111483349789144981 ) ) ;
#653=DIRECTION ( 'NONE',  ( -1.000000000000000000, 0.000000000000000000, 0.000000000000000000 ) ) ;
#654=DIRECTION ( 'NONE',  ( 0.000000000000000000, 0.000000000000000000, 1.000000000000000000 ) ) ;
#655=CARTESIAN_POINT ( 'NONE',  ( -1.109824446838103551, -148.3982683980276533, 1.619194360872903804 ) ) ;
#657=CARTESIAN_POINT ( 'NONE',  ( -8.385254915620292238, 22.12961257269105531, -3.907772785857374249E-17 ) ) ;
#660=EDGE_CURVE ( 'NONE', #1806, #12845, #2964, .T. ) ;
#663=ORIENTED_EDGE ( 'NONE', *, *, #3817, .F. ) ;
#664=CARTESIAN_POINT ( 'NONE',  ( 1.843109844542686560, -151.2149270183035128, -0.2962055024153073535 ) ) ;
#666=CARTESIAN_POINT ( 'NONE',  ( 6.132836266241635137, -110.2447350134475101, -1.893865185603917922 ) ) ;
#667=DIRECTION ( 'NONE',  ( -0.000000000000000000, -0.000000000000000000, -1.000000000000000000 ) ) ;
#670=CARTESIAN_POINT ( 'NONE',  ( 1.369039070337584096, -125.1255798145694200, -4.439507930958486170 ) ) ;
#672=CARTESIAN_POINT ( 'NONE',  ( 10.00000000000000000, 98.00000000000000000, -0.5000000000000000000 ) ) ;
#673=CARTESIAN_POINT ( 'NONE',  ( -2.517691654963332357E-15, 90.00000000000000000, -1.589271161308885878E-16 ) ) ;
#675=AXIS2_PLACEMENT_3D ( 'NONE', #13174, #7668, #12891 ) ;
#678=CARTESIAN_POINT ( 'NONE',  ( 8.385254915620290461, 62.45333659073423860, 2.053795118489800004E-15 ) ) ;
#679=ORIENTED_EDGE ( 'NONE', *, *, #10110, .F. ) ;
#680=CARTESIAN_POINT ( 'NONE',  ( -1.651792843486753513E-16, 5.904668890677672088, -1.042679998336861873E-17 ) ) ;
#683=CARTESIAN_POINT ( 'NONE',  ( -2.937342332082010898, -95.36363636365091168, -3.570487953801811276 ) ) ;
#684=AXIS2_PLACEMENT_3D ( 'NONE', #416, #1511, #3396 ) ;
#688=ORIENTED_EDGE ( 'NONE', *, *, #2950, .T. ) ;
#689=FACE_BOUND ( 'NONE', #195, .T. ) ;
#691=CARTESIAN_POINT ( 'NONE',  ( 1.315456961488612908, -124.8181818181797098, -4.422452657364230433 ) ) ;
#692=AXIS2_PLACEMENT_3D ( 'NONE', #9743, #2236, #1063 ) ;
#693=FACE_OUTER_BOUND ( 'NONE', #13636, .T. ) ;
#694=CARTESIAN_POINT ( 'NONE',  ( 25.00000000000000355, 120.0000000000000284, -0.5000000000000000000 ) ) ;
#695=AXIS2_PLACEMENT_3D ( 'NONE', #13824, #5226, #4237 ) ;
#696=FACE_OUTER_BOUND ( 'NONE', #7553, .T. ) ;
#699=CARTESIAN_POINT ( 'NONE',  ( -4.471182088707197799, 90.98125128669738615, 2.240943909473569917 ) ) ;
#700=EDGE_LOOP ( 'NONE', ( #13623, #151, #5803, #4865 ) ) ;
#701=EDGE_CURVE ( 'NONE', #1478, #9187, #6462, .T. ) ;
#702=AXIS2_PLACEMENT_3D ( 'NONE', #7338, #908, #8404 ) ;
#703=CARTESIAN_POINT ( 'NONE',  ( -7.331936968928880916, -85.59420029784318729, 5.937794338404503769 ) ) ;
#705=AXIS2_PLACEMENT_3D ( 'NONE', #8682, #11776, #4329 ) ;
#707=EDGE_CURVE ( 'NONE', #2716, #6241, #8627, .T. ) ;
#710=DIRECTION ( 'NONE',  ( -0.000000000000000000, -0.000000000000000000, -1.000000000000000000 ) ) ;
#712=CARTESIAN_POINT ( 'NONE',  ( -4.569026568008291989, -119.8678717589752836, -2.546033243568991633 ) ) ;
#713=CARTESIAN_POINT ( 'NONE',  ( -4.330127018922195425, 92.00000000000000000, 2.500000000000000000 ) ) ;
#714=VECTOR ( 'NONE', #10865, 1000.000000000000000 ) ;
#715=AXIS2_PLACEMENT_3D ( 'NONE', #7101, #4647, #7031 ) ;
#717=VERTEX_POINT ( 'NONE', #1204 ) ;
#721=CARTESIAN_POINT ( 'NONE',  ( 0.1760972876109651863, -80.66666666666658614, 10.02690338805414072 ) ) ;
#722=EDGE_LOOP ( 'NONE', ( #11943, #9603, #12720, #1677 ) ) ;
#724=LINE ( 'NONE', #2959, #8363 ) ;
#726=AXIS2_PLACEMENT_3D ( 'NONE', #1717, #10409, #13405 ) ;
#729=DIRECTION ( 'NONE',  ( -2.797435172181481150E-17, 1.000000000000000000, -1.765856845898762549E-18 ) ) ;
#732=EDGE_LOOP ( 'NONE', ( #6280, #5930, #13577, #2245 ) ) ;
#738=CARTESIAN_POINT ( 'NONE',  ( -6.341686887230054914, -95.24900142918743029, -5.248039533272778279 ) ) ;
#739=CARTESIAN_POINT ( 'NONE',  ( -33.99999999999999289, 108.0000000000000142, 2.500000000000000000 ) ) ;
#741=ORIENTED_EDGE ( 'NONE', *, *, #7517, .T. ) ;
#743=CARTESIAN_POINT ( 'NONE',  ( -1.570139719938473233, -148.1629368621884169, 1.428393430366113881 ) ) ;
#745=CARTESIAN_POINT ( 'NONE',  ( -0.6059849261898251349, -166.5454546808362863, 5.665245053931520225 ) ) ;
#746=DIRECTION ( 'NONE',  ( -2.797435172181481150E-17, 1.000000000000000000, -1.765856845898762549E-18 ) ) ;
#748=DIRECTION ( 'NONE',  ( -1.000000000000000000, 0.000000000000000000, 0.000000000000000000 ) ) ;
#751=DIRECTION ( 'NONE',  ( -0.000000000000000000, -0.000000000000000000, -1.000000000000000000 ) ) ;
#753=CARTESIAN_POINT ( 'NONE',  ( 3.784192700541107346, -60.99999999999997158, 1.982393907671070599 ) ) ;
#754=VECTOR ( 'NONE', #380, 1000.000000000000000 ) ;
#755=ORIENTED_EDGE ( 'NONE', *, *, #6867, .F. ) ;
#757=DIRECTION ( 'NONE',  ( -2.797435172181481150E-17, 1.000000000000000000, -1.765856845898762549E-18 ) ) ;
#761=CARTESIAN_POINT ( 'NONE',  ( -8.385254915620286909, 34.17900274070598243, -16.77050983124057737 ) ) ;
#762=CARTESIAN_POINT ( 'NONE',  ( -25.00000000000000355, 120.0000000000000284, -0.5000000000000000000 ) ) ;
#763=DIRECTION ( 'NONE',  ( 1.000000000000000000, 0.000000000000000000, 0.000000000000000000 ) ) ;
#765=CARTESIAN_POINT ( 'NONE',  ( -4.974937185533102380, 90.00000000000000000, 0.5000000000000000000 ) ) ;
#770=DIRECTION ( 'NONE',  ( -2.797435172181481150E-17, 1.000000000000000000, -1.765856845898762549E-18 ) ) ;
#773=CARTESIAN_POINT ( 'NONE',  ( 10.69381717166375623, -2.714886977913000266, 1.320497585966558038E-15 ) ) ;
#776=EDGE_CURVE ( 'NONE', #12557, #8762, #302, .T. ) ;
#782=CARTESIAN_POINT ( 'NONE',  ( -12.99579180576516890, -11.31471392308272605, -1.551565153650648068E-15 ) ) ;
#783=ORIENTED_EDGE ( 'NONE', *, *, #6529, .T. ) ;
#784=CARTESIAN_POINT ( 'NONE',  ( 7.500230552170977560, -73.18181818181670906, 6.960552780978377818 ) ) ;
#790=DIRECTION ( 'NONE',  ( 1.000000000000000000, 0.000000000000000000, 0.000000000000000000 ) ) ;
#793=CARTESIAN_POINT ( 'NONE',  ( 0.09329349605429697323, -158.9451967104999142, -1.495111656224116015 ) ) ;
#798=ORIENTED_EDGE ( 'NONE', *, *, #1974, .F. ) ;
#802=EDGE_CURVE ( 'NONE', #149, #11499, #5829, .T. ) ;
#803=CARTESIAN_POINT ( 'NONE',  ( -2.332330206345282431, -138.2006080288368253, -2.072564583226628621 ) ) ;
#805=VECTOR ( 'NONE', #1497, 1000.000000000000000 ) ;
#807=CARTESIAN_POINT ( 'NONE',  ( 1.982309627628414228, -99.59031080125953395, 7.452550939933153984 ) ) ;
#808=CARTESIAN_POINT ( 'NONE',  ( 0.04956920569949166411, -160.9696969715462274, -0.4964001826764073422 ) ) ;
#810=CIRCLE ( 'NONE', #8403, 14.99999999999998934 ) ;
#816=EDGE_CURVE ( 'NONE', #2083, #7574, #4917, .T. ) ;
#828=CARTESIAN_POINT ( 'NONE',  ( -2.733214919987291491, -81.93939393967723106, 9.473759075773607208 ) ) ;
#830=CARTESIAN_POINT ( 'NONE',  ( 3.915768125671617028, -76.35064935075745041, 2.796074470131364453 ) ) ;
#831=DIRECTION ( 'NONE',  ( -1.000000000000000000, 0.000000000000000000, 0.000000000000000000 ) ) ;
#833=FACE_OUTER_BOUND ( 'NONE', #4970, .T. ) ;
#834=CARTESIAN_POINT ( 'NONE',  ( 12.99553232110413781, 77.04820039461787928, 0.000000000000000000 ) ) ;
#837=CARTESIAN_POINT ( 'NONE',  ( -8.277783874104137851, -87.06151417676248627, 4.224168635135138850 ) ) ;
#839=CYLINDRICAL_SURFACE ( 'NONE', #9881, 2.000000000000000000 ) ;
#842=CARTESIAN_POINT ( 'NONE',  ( -12.99579180576516002, -1.889935973073298747, -25.99158361153033070 ) ) ;
#843=CARTESIAN_POINT ( 'NONE',  ( -0.1741440327402171140, -159.7354236601310618, 1.510075946869572139 ) ) ;
#845=( BOUNDED_SURFACE ( )  B_SPLINE_SURFACE ( 3, 3, ( 
 ( #6944, #9195, #8914, #2607 ),
 ( #3860, #13219, #11084, #12361 ),
 ( #2814, #8141, #1476, #443 ),
 ( #5979, #5756, #12423, #4701 ) ),
 .UNSPECIFIED., .F., .F., .T. ) 
 B_SPLINE_SURFACE_WITH_KNOTS ( ( 4, 4 ),
 ( 4, 4 ),
 ( 0.000000000000000000, 1.000000000000000000 ),
 ( 0.000000000000000000, 1.000000000000000000 ),
 .UNSPECIFIED. ) 
 GEOMETRIC_REPRESENTATION_ITEM ( )  RATIONAL_B_SPLINE_SURFACE ( (
 ( 1.000000000000000000, 0.3333333333333334259, 0.3333333333333334259, 1.000000000000000000),
 ( 1.000000000000000000, 0.3333333333333334259, 0.3333333333333334259, 1.000000000000000000),
 ( 1.000000000000000000, 0.3333333333333334259, 0.3333333333333334259, 1.000000000000000000),
 ( 1.000000000000000000, 0.3333333333333334259, 0.3333333333333334259, 1.000000000000000000) ) ) 
 REPRESENTATION_ITEM ( '' )  SURFACE ( )  );
#849=VERTEX_POINT ( 'NONE', #10319 ) ;
#850=ADVANCED_FACE ( 'NONE', ( #13445 ), #9785, .F. ) ;
#853=CARTESIAN_POINT ( 'NONE',  ( -8.385254915620299343, 78.67828027274755698, -2.258796916435532892E-15 ) ) ;
#854=ORIENTED_EDGE ( 'NONE', *, *, #10805, .F. ) ;
#859=CARTESIAN_POINT ( 'NONE',  ( -2.642019774883006988, -134.5079500460111319, 2.362135513950679666 ) ) ;
#860=DIRECTION ( 'NONE',  ( -0.1234677578012386562, -1.701584941912606716E-18, 0.9923485843107423543 ) ) ;
#861=ORIENTED_EDGE ( 'NONE', *, *, #13453, .F. ) ;
#862=EDGE_LOOP ( 'NONE', ( #10905, #5451, #901, #8011 ) ) ;
#865=DIRECTION ( 'NONE',  ( -2.797435172181481150E-17, 1.000000000000000000, -1.765856845898762549E-18 ) ) ;
#869=CARTESIAN_POINT ( 'NONE',  ( 10.00000000000000000, 92.00000000000000000, 2.500000000000000000 ) ) ;
#870=CARTESIAN_POINT ( 'NONE',  ( 5.038813069536555389, -96.69644570957702001, 6.323701593888624295 ) ) ;
#873=CARTESIAN_POINT ( 'NONE',  ( 41.99999999999999289, 120.0000000000000284, -2.500000000000000000 ) ) ;
#876=CIRCLE ( 'NONE', #4681, 5.000000000000000000 ) ;
#878=CARTESIAN_POINT ( 'NONE',  ( 25.00000000000000355, 120.0000000000000284, 0.5000000000000000000 ) ) ;
#879=CARTESIAN_POINT ( 'NONE',  ( -15.29705854078139993, 90.00000000000000000, -1.589271161308885878E-16 ) ) ;
#880=ORIENTED_EDGE ( 'NONE', *, *, #11978, .F. ) ;
#882=CARTESIAN_POINT ( 'NONE',  ( 9.736331930512850619, -69.99978782402618549, 2.722951059031191612 ) ) ;
#883=CARTESIAN_POINT ( 'NONE',  ( -12.88103206736694695, -118.2727272727293979, -6.757986543075753083 ) ) ;
#884=ORIENTED_EDGE ( 'NONE', *, *, #7402, .F. ) ;
#885=DIRECTION ( 'NONE',  ( -1.000000000000000000, 0.000000000000000000, 0.000000000000000000 ) ) ;
#886=AXIS2_PLACEMENT_3D ( 'NONE', #6133, #5201, #13598 ) ;
#887=VERTEX_POINT ( 'NONE', #11637 ) ;
#889=CYLINDRICAL_SURFACE ( 'NONE', #8820, 15.29705854078139105 ) ;
#890=CARTESIAN_POINT ( 'NONE',  ( 2.401759516345856493, -79.03030303050532268, 10.21173794894131248 ) ) ;
#891=CARTESIAN_POINT ( 'NONE',  ( 2.224981447619138297, -153.6493506492904544, -4.266231359692138625 ) ) ;
#894=CARTESIAN_POINT ( 'NONE',  ( 15.29705854078138394, 47.94714734142005597, 30.59411708156277854 ) ) ;
#897=CARTESIAN_POINT ( 'NONE',  ( 15.29705854078138749, 76.22148119144830503, 1.740418857596140842E-15 ) ) ;
#901=ORIENTED_EDGE ( 'NONE', *, *, #12822, .T. ) ;
#902=CARTESIAN_POINT ( 'NONE',  ( -10.00000000000000711, 92.00000000000000000, 0.5000000000000000000 ) ) ;
#908=DIRECTION ( 'NONE',  ( -2.797435172181481150E-17, 1.000000000000000000, -1.765856845898762549E-18 ) ) ;
#911=AXIS2_PLACEMENT_3D ( 'NONE', #11264, #11326, #1722 ) ;
#912=ORIENTED_EDGE ( 'NONE', *, *, #660, .F. ) ;
#920=ORIENTED_EDGE ( 'NONE', *, *, #9124, .T. ) ;
#921=CARTESIAN_POINT ( 'NONE',  ( 12.99553232110413958, 77.04820039461787928, -25.99106464220826851 ) ) ;
#923=DIRECTION ( 'NONE',  ( -2.797435172181481150E-17, 1.000000000000000000, -1.765856845898762549E-18 ) ) ;
#931=CARTESIAN_POINT ( 'NONE',  ( 3.452401867291364557, -108.4018358419776007, -5.656396446225017804 ) ) ;
#933=ORIENTED_EDGE ( 'NONE', *, *, #12978, .T. ) ;
#935=ADVANCED_FACE ( 'NONE', ( #4068 ), #5189, .T. ) ;
#936=B_SPLINE_CURVE_WITH_KNOTS ( 'NONE', 3,
 ( #8249, #1793, #6082, #4827 ),
 .UNSPECIFIED., .F., .F.,
 ( 4, 4 ),
 ( 0.000000000000000000, 1.000000000000000000 ),
 .UNSPECIFIED. ) ;
#937=ORIENTED_EDGE ( 'NONE', *, *, #12975, .F. ) ;
#938=EDGE_LOOP ( 'NONE', ( #5796, #12498, #1323, #6671 ) ) ;
#940=ORIENTED_EDGE ( 'NONE', *, *, #7461, .F. ) ;
#941=DIRECTION ( 'NONE',  ( -0.000000000000000000, -0.000000000000000000, -1.000000000000000000 ) ) ;
#942=CARTESIAN_POINT ( 'NONE',  ( 0.3822922200478666155, -101.0602069644519361, 7.519122157920856253 ) ) ;
#944=CARTESIAN_POINT ( 'NONE',  ( 12.99579180576516890, 64.08350967699263379, 1.492731922528324790E-15 ) ) ;
#947=DIRECTION ( 'NONE',  ( 1.000000000000000000, 0.000000000000000000, 0.000000000000000000 ) ) ;
#949=ADVANCED_FACE ( 'NONE', ( #7224 ), #12480, .T. ) ;
#950=EDGE_CURVE ( 'NONE', #6854, #11418, #8882, .T. ) ;
#951=DIRECTION ( 'NONE',  ( -2.797435172181481150E-17, 1.000000000000000000, -1.765856845898762549E-18 ) ) ;
#952=DIRECTION ( 'NONE',  ( 0.000000000000000000, 0.000000000000000000, 1.000000000000000000 ) ) ;
#954=CARTESIAN_POINT ( 'NONE',  ( -12.85867081388705202, -161.0909090911694932, -2.071848600304991628 ) ) ;
#955=ADVANCED_FACE ( 'NONE', ( #6648 ), #3283, .T. ) ;
#957=LINE ( 'NONE', #5218, #13120 ) ;
#959=DIRECTION ( 'NONE',  ( 0.000000000000000000, 0.000000000000000000, 1.000000000000000000 ) ) ;
#960=FACE_OUTER_BOUND ( 'NONE', #5437, .T. ) ;
#962=CARTESIAN_POINT ( 'NONE',  ( -3.894934744997970100, -89.44155844158483148, 2.935215040339494763 ) ) ;
#964=CARTESIAN_POINT ( 'NONE',  ( 10.69346802281034670, 49.59884612375012125, 2.619144277183853949E-15 ) ) ;
#967=CARTESIAN_POINT ( 'NONE',  ( -4.804060984082282104, 90.20500167315060480, 1.391503737930616991 ) ) ;
#968=CIRCLE ( 'NONE', #8787, 8.385254915620292238 ) ;
#969=EDGE_CURVE ( 'NONE', #3210, #1805, #10968, .T. ) ;
#974=CARTESIAN_POINT ( 'NONE',  ( -12.99579180576516180, -11.31471392308272428, -25.99158361153033425 ) ) ;
#976=CARTESIAN_POINT ( 'NONE',  ( 15.29705854078138394, 55.48535772202409788, 30.59411708156277854 ) ) ;
#977=CARTESIAN_POINT ( 'NONE',  ( 1.489377283214609049, -147.9547819581979979, 1.534577776538655680 ) ) ;
#978=AXIS2_PLACEMENT_3D ( 'NONE', #10454, #11440, #9408 ) ;
#980=CARTESIAN_POINT ( 'NONE',  ( 15.29705854078138927, 47.94714734142005597, 1.790347283588440782E-15 ) ) ;
#982=ORIENTED_EDGE ( 'NONE', *, *, #1139, .T. ) ;
#983=EDGE_LOOP ( 'NONE', ( #6992, #11956, #8964, #6518 ) ) ;
#984=EDGE_CURVE ( 'NONE', #10478, #10108, #1576, .T. ) ;
#987=CARTESIAN_POINT ( 'NONE',  ( 10.69346802281034670, 77.87317997377837742, 1.216646543541944040E-15 ) ) ;
#989=CARTESIAN_POINT ( 'NONE',  ( 15.29705854078139282, 8.361467971976981772, 1.856918518244840178E-15 ) ) ;
#990=CIRCLE ( 'NONE', #4811, 8.385254915620297567 ) ;
#991=CARTESIAN_POINT ( 'NONE',  ( -0.3728392436186487857, -81.93939393937360194, 10.00978956348542326 ) ) ;
#993=CARTESIAN_POINT ( 'NONE',  ( 10.69381717166375267, 63.25855867215299355, 0.000000000000000000 ) ) ;
#996=CARTESIAN_POINT ( 'NONE',  ( 10.69346802281034847, 68.44840202376897764, -21.38693604562068984 ) ) ;
#997=CARTESIAN_POINT ( 'NONE',  ( -0.5124393331798130502, -128.8492006177044118, 4.163771180444989284 ) ) ;
#1005=CYLINDRICAL_SURFACE ( 'NONE', #9526, 15.29705854078139993 ) ;
#1006=CARTESIAN_POINT ( 'NONE',  ( -0.8060388441294140671, -102.1876712484548335, 7.345991765615691449 ) ) ;
#1008=DIRECTION ( 'NONE',  ( -1.000000000000000000, 0.000000000000000000, 0.000000000000000000 ) ) ;
#1010=AXIS2_PLACEMENT_3D ( 'NONE', #3254, #3057, #10751 ) ;
#1014=AXIS2_PLACEMENT_3D ( 'NONE', #10951, #11113, #1354 ) ;
#1015=CARTESIAN_POINT ( 'NONE',  ( 12.99553232110413781, 67.62342244460847951, 0.000000000000000000 ) ) ;
#1020=CARTESIAN_POINT ( 'NONE',  ( -20.16774360697312218, -62.63636366012922707, 2.887214123323314841 ) ) ;
#1027=AXIS2_PLACEMENT_3D ( 'NONE', #3290, #11714, #10718 ) ;
#1028=CYLINDRICAL_SURFACE ( 'NONE', #11070, 8.385254915620292238 ) ;
#1029=B_SPLINE_CURVE_WITH_KNOTS ( 'NONE', 3,
 ( #12936, #2255, #8632, #233 ),
 .UNSPECIFIED., .F., .F.,
 ( 4, 4 ),
 ( 0.000000000000000000, 1.000000000000000000 ),
 .UNSPECIFIED. ) ;
#1031=CARTESIAN_POINT ( 'NONE',  ( -12.66071438417701778, -140.5584415584565079, -5.506376209458912818 ) ) ;
#1035=CARTESIAN_POINT ( 'NONE',  ( -15.29705854078138927, -36.87585420866476227, -1.743114418628290232E-15 ) ) ;
#1038=AXIS2_PLACEMENT_3D ( 'NONE', #10347, #9293, #11462 ) ;
#1039=EDGE_LOOP ( 'NONE', ( #4656, #2047, #6993, #8729 ) ) ;
#1040=CIRCLE ( 'NONE', #12469, 24.99999999999998934 ) ;
#1041=EDGE_CURVE ( 'NONE', #11894, #11396, #10088, .T. ) ;
#1044=FACE_OUTER_BOUND ( 'NONE', #8362, .T. ) ;
#1045=EDGE_CURVE ( 'NONE', #1633, #1929, #12847, .T. ) ;
#1046=CARTESIAN_POINT ( 'NONE',  ( 12.99553232110412893, 67.62342244460847951, 25.99106464220826851 ) ) ;
#1047=CARTESIAN_POINT ( 'NONE',  ( -10.69346802281034847, 30.74929022373126841, -2.692987470725032262E-15 ) ) ;
#1048=ADVANCED_FACE ( 'NONE', ( #10908 ), #10, .T. ) ;
#1051=CARTESIAN_POINT ( 'NONE',  ( 0.8615837080506374424, -151.0610343063302139, 1.652123164482231843 ) ) ;
#1052=CIRCLE ( 'NONE', #5516, 24.99999999999998934 ) ;
#1054=ORIENTED_EDGE ( 'NONE', *, *, #10887, .F. ) ;
#1063=DIRECTION ( 'NONE',  ( -1.000000000000000000, -5.171946152600901754E-17, 0.000000000000000000 ) ) ;
#1064=EDGE_CURVE ( 'NONE', #7475, #1472, #12093, .T. ) ;
#1067=CARTESIAN_POINT ( 'NONE',  ( 5.223624298350400430, -118.2088257147582340, 1.581264552922174049 ) ) ;
#1069=VERTEX_POINT ( 'NONE', #9950 ) ;
#1070=B_SPLINE_CURVE_WITH_KNOTS ( 'NONE', 3,
 ( #4019, #11528, #11726, #1079 ),
 .UNSPECIFIED., .F., .F.,
 ( 4, 4 ),
 ( 0.000000000000000000, 0.002999984648040830010 ),
 .UNSPECIFIED. ) ;
#1071=EDGE_LOOP ( 'NONE', ( #5655, #1958, #7489, #10006 ) ) ;
#1076=CARTESIAN_POINT ( 'NONE',  ( 4.325223352540145783, -97.40615224493882351, 6.735768676233161223 ) ) ;
#1078=CARTESIAN_POINT ( 'NONE',  ( -1.024176664971890860, -142.5800865798597670, -2.358741788134935735 ) ) ;
#1079=CARTESIAN_POINT ( 'NONE',  ( 9.736331930512850619, -69.99978782402618549, 2.722951059031191612 ) ) ;
#1080=CARTESIAN_POINT ( 'NONE',  ( -0.08455446438426061917, -80.00111630769902149, -10.00862910738027622 ) ) ;
#1083=CARTESIAN_POINT ( 'NONE',  ( -9.888538082662732265, -70.78787878787531440, -1.806551902650875840 ) ) ;
#1086=VECTOR ( 'NONE', #12985, 1000.000000000000000 ) ;
#1088=CARTESIAN_POINT ( 'NONE',  ( 12.99579180576516713, 73.50828762700209040, 1.478592833246211056E-15 ) ) ;
#1089=ORIENTED_EDGE ( 'NONE', *, *, #632, .F. ) ;
#1091=CARTESIAN_POINT ( 'NONE',  ( -10.69381717166375800, -12.13966492792242846, -1.266741076154724095E-15 ) ) ;
#1094=DIRECTION ( 'NONE',  ( -2.797435172181481150E-17, 1.000000000000000000, -1.765856845898762549E-18 ) ) ;
#1095=CARTESIAN_POINT ( 'NONE',  ( 8.385254915620290461, 3.280056672672171381, 16.77050983124058803 ) ) ;
#1099=CARTESIAN_POINT ( 'NONE',  ( 8.385254915620294014, 24.75422479069652582, 9.996449125125100638E-16 ) ) ;
#1101=CARTESIAN_POINT ( 'NONE',  ( -12.99553232110414136, 77.04820039461787928, -1.863605890287647356E-15 ) ) ;
#1105=ORIENTED_EDGE ( 'NONE', *, *, #9011, .T. ) ;
#1114=B_SPLINE_CURVE_WITH_KNOTS ( 'NONE', 3,
 ( #9543, #8352, #1834, #4988 ),
 .UNSPECIFIED., .F., .F.,
 ( 4, 4 ),
 ( 0.000000000000000000, 1.000000000000000000 ),
 .UNSPECIFIED. ) ;
#1115=CIRCLE ( 'NONE', #6929, 8.385254915620292238 ) ;
#1116=CARTESIAN_POINT ( 'NONE',  ( -15.29705854078138749, 10.24803554138234496, -1.909542505269288522E-15 ) ) ;
#1120=EDGE_CURVE ( 'NONE', #9797, #887, #7165, .T. ) ;
#1122=EDGE_CURVE ( 'NONE', #7574, #1929, #10739, .T. ) ;
#1124=CIRCLE ( 'NONE', #8726, 15.29705854078139637 ) ;
#1125=AXIS2_PLACEMENT_3D ( 'NONE', #11875, #4574, #6551 ) ;
#1126=CARTESIAN_POINT ( 'NONE',  ( 10.00000000000000000, 92.00000000000000000, -0.5000000000000000000 ) ) ;
#1127=ORIENTED_EDGE ( 'NONE', *, *, #11633, .T. ) ;
#1128=CARTESIAN_POINT ( 'NONE',  ( 10.00000000000000000, 92.00000000000000000, -0.5000000000000000000 ) ) ;
#1129=CARTESIAN_POINT ( 'NONE',  ( -10.00000000000000711, 99.99999999999994316, 0.5000000000000000000 ) ) ;
#1133=CARTESIAN_POINT ( 'NONE',  ( -7.323500324365400438, -96.14321736266329310, -3.508298222391299959 ) ) ;
#1135=EDGE_LOOP ( 'NONE', ( #10525, #11632, #5422, #13706 ) ) ;
#1136=ADVANCED_FACE ( 'NONE', ( #7729 ), #4429, .F. ) ;
#1139=EDGE_CURVE ( 'NONE', #8182, #10177, #6498, .T. ) ;
#1141=EDGE_CURVE ( 'NONE', #2083, #1633, #9870, .T. ) ;
#1143=CYLINDRICAL_SURFACE ( 'NONE', #11409, 15.29705854078139815 ) ;
#1146=VERTEX_POINT ( 'NONE', #12161 ) ;
#1148=CARTESIAN_POINT ( 'NONE',  ( 15.29705854078138927, 38.52236939141059935, -30.59411708156276788 ) ) ;
#1149=CARTESIAN_POINT ( 'NONE',  ( 1.436028440950094742, -80.32363832966076700, -10.00441251861082748 ) ) ;
#1152=CIRCLE ( 'NONE', #8747, 8.385254915620290461 ) ;
#1154=CARTESIAN_POINT ( 'NONE',  ( 0.6059849270565064172, -166.5454544424325718, -5.665245052758470123 ) ) ;
#1155=CARTESIAN_POINT ( 'NONE',  ( -9.991007172155491389, -71.90909090909036649, -2.111483349789142760 ) ) ;
#1159=CIRCLE ( 'NONE', #3378, 15.29705854078139282 ) ;
#1160=CARTESIAN_POINT ( 'NONE',  ( -15.29705854078139637, 74.33491362204294717, -3.876297867647458896E-15 ) ) ;
#1161=EDGE_CURVE ( 'NONE', #3518, #4148, #7840, .T. ) ;
#1166=ORIENTED_EDGE ( 'NONE', *, *, #9006, .F. ) ;
#1170=CIRCLE ( 'NONE', #2960, 50.00000000000001421 ) ;
#1171=CARTESIAN_POINT ( 'NONE',  ( -10.69381717166375623, -2.714886977913000710, -1.300026693482923793E-15 ) ) ;
#1172=CARTESIAN_POINT ( 'NONE',  ( 12.99579180576517246, 26.38439787695498495, -25.99158361153033070 ) ) ;
#1176=VERTEX_POINT ( 'NONE', #1427 ) ;
#1179=CARTESIAN_POINT ( 'NONE',  ( -10.00000000000000711, 139.9999999999999716, -0.5000000000000000000 ) ) ;
#1181=DIRECTION ( 'NONE',  ( 0.000000000000000000, 1.000000000000000000, 0.000000000000000000 ) ) ;
#1183=DIRECTION ( 'NONE',  ( -1.000000000000000000, 0.000000000000000000, 0.000000000000000000 ) ) ;
#1185=ORIENTED_EDGE ( 'NONE', *, *, #4539, .F. ) ;
#1186=CIRCLE ( 'NONE', #2980, 5.000000000000000000 ) ;
#1189=ORIENTED_EDGE ( 'NONE', *, *, #6708, .T. ) ;
#1190=DIRECTION ( 'NONE',  ( -1.000000000000000000, 0.000000000000000000, 0.000000000000000000 ) ) ;
#1191=EDGE_CURVE ( 'NONE', #4658, #10763, #8941, .T. ) ;
#1194=CARTESIAN_POINT ( 'NONE',  ( -7.273479275674047173, -73.48250329347293075, -7.060675431679237057 ) ) ;
#1197=CARTESIAN_POINT ( 'NONE',  ( -15.29705854078139637, 64.91013567203349055, -1.146220074446778111E-16 ) ) ;
#1199=ORIENTED_EDGE ( 'NONE', *, *, #3503, .F. ) ;
#1201=ORIENTED_EDGE ( 'NONE', *, *, #6512, .T. ) ;
#1202=AXIS2_PLACEMENT_3D ( 'NONE', #6544, #2391, #9908 ) ;
#1204=CARTESIAN_POINT ( 'NONE',  ( -33.99999999999999289, 108.0000000000000142, 0.5000000000000000000 ) ) ;
#1205=ORIENTED_EDGE ( 'NONE', *, *, #8589, .T. ) ;
#1208=CIRCLE ( 'NONE', #93, 42.00000000000001421 ) ;
#1209=CARTESIAN_POINT ( 'NONE',  ( -12.99553232110414136, 58.19864449459907974, -3.303875580016498200E-15 ) ) ;
#1210=ADVANCED_FACE ( 'NONE', ( #8649 ), #5552, .T. ) ;
#1212=CARTESIAN_POINT ( 'NONE',  ( -12.99579180576516713, 45.23395377697384134, -1.751278857619846450E-15 ) ) ;
#1213=CARTESIAN_POINT ( 'NONE',  ( 1.066429238991517314, -168.0000000000001421, -0.4719413927851733859 ) ) ;
#1215=CARTESIAN_POINT ( 'NONE',  ( -9.601587402597671073, -70.78787878788241983, -2.975959431766524776 ) ) ;
#1217=EDGE_CURVE ( 'NONE', #1501, #10825, #13244, .T. ) ;
#1220=ORIENTED_EDGE ( 'NONE', *, *, #4700, .F. ) ;
#1225=DIRECTION ( 'NONE',  ( -1.000000000000000000, 0.000000000000000000, 0.000000000000000000 ) ) ;
#1227=AXIS2_PLACEMENT_3D ( 'NONE', #6619, #9995, #5635 ) ;
#1229=VERTEX_POINT ( 'NONE', #11110 ) ;
#1230=DIRECTION ( 'NONE',  ( -0.8907235428302473501, 0.4545454545454531425, 0.000000000000000000 ) ) ;
#1231=CARTESIAN_POINT ( 'NONE',  ( 8.385254915620294014, 3.280056672672171381, 2.053795118489800793E-15 ) ) ;
#1232=EDGE_CURVE ( 'NONE', #4529, #4849, #6504, .T. ) ;
#1233=VECTOR ( 'NONE', #7883, 1000.000000000000114 ) ;
#1234=B_SPLINE_CURVE_WITH_KNOTS ( 'NONE', 3,
 ( #10165, #572, #4533, #8815 ),
 .UNSPECIFIED., .F., .F.,
 ( 4, 4 ),
 ( 0.000000000000000000, 1.000000000000000000 ),
 .UNSPECIFIED. ) ;
#1237=CYLINDRICAL_SURFACE ( 'NONE', #11778, 8.385254915620292238 ) ;
#1240=CARTESIAN_POINT ( 'NONE',  ( 12.99579180576515647, 16.95961992694555676, 25.99158361153032359 ) ) ;
#1242=DIRECTION ( 'NONE',  ( -2.797435172181481150E-17, 1.000000000000000000, -1.765856845898762549E-18 ) ) ;
#1245=ORIENTED_EDGE ( 'NONE', *, *, #1141, .F. ) ;
#1249=PRODUCT_DEFINITION_FORMATION_WITH_SPECIFIED_SOURCE ( 'ANY', '', #10016, .NOT_KNOWN. ) ;
#1251=DIRECTION ( 'NONE',  ( -2.797435172181481150E-17, 1.000000000000000000, -1.765856845898762549E-18 ) ) ;
#1253=CARTESIAN_POINT ( 'NONE',  ( 12.99553232110413958, 11.07475474455194053, 3.182987412051231773E-15 ) ) ;
#1255=ORIENTED_EDGE ( 'NONE', *, *, #7784, .F. ) ;
#1256=ORIENTED_EDGE ( 'NONE', *, *, #354, .F. ) ;
#1260=CARTESIAN_POINT ( 'NONE',  ( -1.964926745380544348, -77.94210580202374672, -9.914063068206223406 ) ) ;
#1261=CARTESIAN_POINT ( 'NONE',  ( 2.974540731479519701E-17, -1.063309978032472847, 1.877653204021102445E-18 ) ) ;
#1262=CARTESIAN_POINT ( 'NONE',  ( 4.130090007162176668, 90.90347248489021581, -2.819710018450384048 ) ) ;
#1265=ORIENTED_EDGE ( 'NONE', *, *, #114, .T. ) ;
#1267=CARTESIAN_POINT ( 'NONE',  ( -4.317896099768527840, 91.66241202089433671, 2.521541801375117853 ) ) ;
#1270=DIRECTION ( 'NONE',  ( 0.000000000000000000, 0.000000000000000000, 1.000000000000000000 ) ) ;
#1274=LINE ( 'NONE', #7718, #3945 ) ;
#1277=( BOUNDED_SURFACE ( )  B_SPLINE_SURFACE ( 3, 3, ( 
 ( #10028, #438, #8065, #644 ),
 ( #3786, #8982, #13288, #1539 ),
 ( #3637, #4909, #7011, #5823 ),
 ( #11291, #9186, #7928, #12211 ) ),
 .UNSPECIFIED., .F., .F., .F. ) 
 B_SPLINE_SURFACE_WITH_KNOTS ( ( 4, 4 ),
 ( 4, 4 ),
 ( 0.000000000000000000, 1.000000000000000000 ),
 ( 0.000000000000000000, 1.000000000000000000 ),
 .UNSPECIFIED. ) 
 GEOMETRIC_REPRESENTATION_ITEM ( )  RATIONAL_B_SPLINE_SURFACE ( (
 ( 1.000000000000000000, 0.3333333333333334259, 0.3333333333333334259, 1.000000000000000000),
 ( 1.000000000000000000, 0.3333333333333334259, 0.3333333333333334259, 1.000000000000000000),
 ( 1.000000000000000000, 0.3333333333333334259, 0.3333333333333334259, 1.000000000000000000),
 ( 1.000000000000000000, 0.3333333333333334259, 0.3333333333333334259, 1.000000000000000000) ) ) 
 REPRESENTATION_ITEM ( '' )  SURFACE ( )  );
#1281=CARTESIAN_POINT ( 'NONE',  ( -12.99579180576517068, 73.50828762700209040, -3.329728542850656599E-15 ) ) ;
#1284=EDGE_CURVE ( 'NONE', #4658, #12645, #13017, .T. ) ;
#1286=CARTESIAN_POINT ( 'NONE',  ( 10.00000000000000000, 98.00000000000000000, 0.5000000000000000000 ) ) ;
#1293=CARTESIAN_POINT ( 'NONE',  ( -10.69381717166375978, 25.55944687211528787, 21.38763434332751245 ) ) ;
#1295=CARTESIAN_POINT ( 'NONE',  ( -8.385254915620292238, -22.36966495935058319, 3.950162600893091522E-17 ) ) ;
#1296=CARTESIAN_POINT ( 'NONE',  ( 35.20000000000002416, 106.4000000000000199, 2.500000000000000000 ) ) ;
#1297=CARTESIAN_POINT ( 'NONE',  ( 12.99579180576517601, -30.16426982310158067, 3.183050967463144563E-15 ) ) ;
#1299=DIRECTION ( 'NONE',  ( -1.000000000000000000, -5.171946152600901754E-17, 0.000000000000000000 ) ) ;
#1302=AXIS2_PLACEMENT_3D ( 'NONE', #287, #3633, #1682 ) ;
#1303=ADVANCED_FACE ( 'NONE', ( #3952 ), #8974, .T. ) ;
#1306=CARTESIAN_POINT ( 'NONE',  ( -10.00000000000000711, 139.9999999999999716, 2.500000000000000000 ) ) ;
#1307=CARTESIAN_POINT ( 'NONE',  ( 15.29705854078138927, 90.00000000000000000, 1.714422261702872766E-15 ) ) ;
#1308=CARTESIAN_POINT ( 'NONE',  ( 8.385254915620294014, -15.56949922734665570, 1.052073721316228694E-15 ) ) ;
#1309=CARTESIAN_POINT ( 'NONE',  ( 7.679260624019852705E-16, -27.45107625865536605, 4.847467093863555185E-17 ) ) ;
#1312=ADVANCED_FACE ( 'NONE', ( #11256 ), #4731, .T. ) ;
#1315=VERTEX_POINT ( 'NONE', #8228 ) ;
#1316=DIRECTION ( 'NONE',  ( -2.797435172181481150E-17, 1.000000000000000000, -1.765856845898762549E-18 ) ) ;
#1317=CARTESIAN_POINT ( 'NONE',  ( 48.00000000000000000, 120.0000000000000284, -0.5000000000000000000 ) ) ;
#1320=CARTESIAN_POINT ( 'NONE',  ( 3.629742700906665842, 90.29727615934677942, -3.441963681523289686 ) ) ;
#1321=CARTESIAN_POINT ( 'NONE',  ( -7.363455934862510155, -88.30281729203618113, 5.335658674741773133 ) ) ;
#1323=ORIENTED_EDGE ( 'NONE', *, *, #10531, .T. ) ;
#1324=CIRCLE ( 'NONE', #6265, 2.000000000000003997 ) ;
#1326=ORIENTED_EDGE ( 'NONE', *, *, #12213, .F. ) ;
#1331=DIRECTION ( 'NONE',  ( 2.797435172181480534E-17, -1.000000000000000000, 1.765856845898762164E-18 ) ) ;
#1333=CARTESIAN_POINT ( 'NONE',  ( 10.69381717166374912, 34.98422482212468054, 21.38763434332751245 ) ) ;
#1334=CARTESIAN_POINT ( 'NONE',  ( 12.99579180576517068, 7.534841976936129448, -25.99158361153032359 ) ) ;
#1337=CARTESIAN_POINT ( 'NONE',  ( -0.5048931899935213963, -158.0606060608750170, -1.721373026808497686 ) ) ;
#1339=DIRECTION ( 'NONE',  ( -1.000000000000000000, 0.000000000000000000, 0.000000000000000000 ) ) ;
#1346=CARTESIAN_POINT ( 'NONE',  ( -10.69381717166375090, 72.68333662216240043, -21.38763434332750890 ) ) ;
#1350=DIRECTION ( 'NONE',  ( 1.000000000000000000, 2.797435172181480534E-17, -0.000000000000000000 ) ) ;
#1354=DIRECTION ( 'NONE',  ( -1.000000000000000000, 0.000000000000000000, 0.000000000000000000 ) ) ;
#1356=LINE ( 'NONE', #4508, #9291 ) ;
#1358=CARTESIAN_POINT ( 'NONE',  ( 12.99579180576516535, 45.23395377697384134, 1.521010101092551666E-15 ) ) ;
#1360=ADVANCED_FACE ( 'NONE', ( #4804 ), #4937, .T. ) ;
#1362=CARTESIAN_POINT ( 'NONE',  ( -1.077638310512993291E-15, 38.52236939141059935, -6.802498971006334016E-17 ) ) ;
#1363=CARTESIAN_POINT ( 'NONE',  ( -12.99553232110413958, 67.62342244460847951, -1.830320272959447658E-15 ) ) ;
#1365=SHAPE_REPRESENTATION ( 'Threaded Steel Worm Screw Spindle', ( #8193 ), #11552 ) ;
#1369=CARTESIAN_POINT ( 'NONE',  ( 8.385254915620292238, 15.32944684068712782, 2.053795118489800004E-15 ) ) ;
#1371=DIRECTION ( 'NONE',  ( -0.000000000000000000, -0.000000000000000000, -1.000000000000000000 ) ) ;
#1373=EDGE_LOOP ( 'NONE', ( #9014, #4066, #10422, #13661 ) ) ;
#1379=ADVANCED_FACE ( 'NONE', ( #6065 ), #9145, .T. ) ;
#1382=DIRECTION ( 'NONE',  ( -2.797435172181481150E-17, 1.000000000000000000, -1.765856845898762549E-18 ) ) ;
#1383=CARTESIAN_POINT ( 'NONE',  ( 4.789632241632986620, -77.94522257074953586, 8.921723374081109270 ) ) ;
#1386=EDGE_CURVE ( 'NONE', #12240, #1176, #4981, .T. ) ;
#1388=ORIENTED_EDGE ( 'NONE', *, *, #4419, .F. ) ;
#1391=DIRECTION ( 'NONE',  ( -1.000000000000000000, 0.000000000000000000, 0.000000000000000000 ) ) ;
#1394=ADVANCED_FACE ( 'NONE', ( #6182 ), #3012, .T. ) ;
#1398=CARTESIAN_POINT ( 'NONE',  ( -3.521118371085406373, -100.8219657368393030, -6.686088967780647430 ) ) ;
#1403=ORIENTED_EDGE ( 'NONE', *, *, #9175, .T. ) ;
#1404=AXIS2_PLACEMENT_3D ( 'NONE', #13762, #9455, #1944 ) ;
#1408=DIRECTION ( 'NONE',  ( -0.8000000000000008216, 0.5999999999999988676, 0.000000000000000000 ) ) ;
#1409=CARTESIAN_POINT ( 'NONE',  ( 0.000000000000000000, 0.000000000000000000, 0.000000000000000000 ) ) ;
#1410=CARTESIAN_POINT ( 'NONE',  ( 12.99553232110413781, 58.19864449459907974, 1.506840924385250240E-15 ) ) ;
#1411=DIRECTION ( 'NONE',  ( -1.000000000000000000, 0.000000000000000000, 0.000000000000000000 ) ) ;
#1412=AXIS2_PLACEMENT_3D ( 'NONE', #9958, #4403, #11982 ) ;
#1414=CARTESIAN_POINT ( 'NONE',  ( 8.385254915620297567, -15.56949922734665748, -16.77050983124058803 ) ) ;
#1415=CARTESIAN_POINT ( 'NONE',  ( 4.278103086407295308, -97.41991341990937769, 7.774081346648461732 ) ) ;
#1416=CARTESIAN_POINT ( 'NONE',  ( -10.00000000000000711, 139.9999999999999716, 2.500000000000000000 ) ) ;
#1417=CARTESIAN_POINT ( 'NONE',  ( 15.29705854078138927, -18.02629830864593785, 30.59411708156278564 ) ) ;
#1418=DIRECTION ( 'NONE',  ( -0.000000000000000000, -0.000000000000000000, -1.000000000000000000 ) ) ;
#1419=VERTEX_POINT ( 'NONE', #12031 ) ;
#1421=VERTEX_POINT ( 'NONE', #6775 ) ;
#1424=CARTESIAN_POINT ( 'NONE',  ( 10.00000000000000000, 90.00000000000000000, 0.5000000000000000000 ) ) ;
#1425=DIRECTION ( 'NONE',  ( -0.000000000000000000, -0.000000000000000000, -1.000000000000000000 ) ) ;
#1426=DIRECTION ( 'NONE',  ( -0.000000000000000000, -0.000000000000000000, -1.000000000000000000 ) ) ;
#1427=CARTESIAN_POINT ( 'NONE',  ( 15.29705854078138749, 47.94714734142005597, 1.790347283588440388E-15 ) ) ;
#1428=EDGE_LOOP ( 'NONE', ( #10008, #3383, #8004, #1403 ) ) ;
#1431=ORIENTED_EDGE ( 'NONE', *, *, #3497, .F. ) ;
#1432=DIRECTION ( 'NONE',  ( -1.000000000000000000, 0.000000000000000000, 0.000000000000000000 ) ) ;
#1433=CARTESIAN_POINT ( 'NONE',  ( 12.99579180576516357, 16.95961992694555676, 0.000000000000000000 ) ) ;
#1437=CARTESIAN_POINT ( 'NONE',  ( -4.259889090956146873, -78.36053271697988976, -9.185913463276904167 ) ) ;
#1438=CARTESIAN_POINT ( 'NONE',  ( 15.29705854078139460, -29.33764382806072746, 30.59411708156279985 ) ) ;
#1439=CARTESIAN_POINT ( 'NONE',  ( -8.385254915620295790, -34.41905512736551032, 6.077912412602530076E-17 ) ) ;
#1440=DIRECTION ( 'NONE',  ( -1.000000000000000000, 0.000000000000000000, 0.000000000000000000 ) ) ;
#1442=ORIENTED_EDGE ( 'NONE', *, *, #8928, .F. ) ;
#1444=EDGE_CURVE ( 'NONE', #2799, #3806, #8730, .T. ) ;
#1445=AXIS2_PLACEMENT_3D ( 'NONE', #4826, #13624, #10423 ) ;
#1447=CARTESIAN_POINT ( 'NONE',  ( -2.237684797877293663E-15, 79.99058638175036151, -1.412519245696701158E-16 ) ) ;
#1448=EDGE_LOOP ( 'NONE', ( #11783, #1558, #7098, #2655 ) ) ;
#1449=( BOUNDED_SURFACE ( )  B_SPLINE_SURFACE ( 3, 3, ( 
 ( #10572, #12754, #9589, #5369 ),
 ( #13838, #9463, #8464, #7414 ),
 ( #7543, #6503, #1046, #6234 ),
 ( #8337, #8402, #9660, #11691 ) ),
 .UNSPECIFIED., .F., .F., .T. ) 
 B_SPLINE_SURFACE_WITH_KNOTS ( ( 4, 4 ),
 ( 4, 4 ),
 ( 0.000000000000000000, 1.000000000000000000 ),
 ( 0.000000000000000000, 1.000000000000000000 ),
 .UNSPECIFIED. ) 
 GEOMETRIC_REPRESENTATION_ITEM ( )  RATIONAL_B_SPLINE_SURFACE ( (
 ( 1.000000000000000000, 0.3333333333333334259, 0.3333333333333334259, 1.000000000000000000),
 ( 1.000000000000000000, 0.3333333333333334259, 0.3333333333333334259, 1.000000000000000000),
 ( 1.000000000000000000, 0.3333333333333334259, 0.3333333333333334259, 1.000000000000000000),
 ( 1.000000000000000000, 0.3333333333333334259, 0.3333333333333334259, 1.000000000000000000) ) ) 
 REPRESENTATION_ITEM ( '' )  SURFACE ( )  );
#1452=CARTESIAN_POINT ( 'NONE',  ( 10.11144057928414242, -69.99977036137985920, -0.2534939170199681513 ) ) ;
#1454=ORIENTED_EDGE ( 'NONE', *, *, #5490, .F. ) ;
#1456=ORIENTED_EDGE ( 'NONE', *, *, #4730, .T. ) ;
#1457=EDGE_CURVE ( 'NONE', #2229, #11958, #5249, .T. ) ;
#1459=EDGE_LOOP ( 'NONE', ( #3631, #4186, #3330, #12674 ) ) ;
#1460=VERTEX_POINT ( 'NONE', #11700 ) ;
#1466=DIRECTION ( 'NONE',  ( -0.000000000000000000, -0.000000000000000000, -1.000000000000000000 ) ) ;
#1472=VERTEX_POINT ( 'NONE', #9159 ) ;
#1476=CARTESIAN_POINT ( 'NONE',  ( 12.99553232110413958, -26.62435705548576692, 25.99106464220828983 ) ) ;
#1477=CARTESIAN_POINT ( 'NONE',  ( 8.152362820469006621, -73.18181818182262077, 5.943141306424061021 ) ) ;
#1478=VERTEX_POINT ( 'NONE', #1591 ) ;
#1479=CARTESIAN_POINT ( 'NONE',  ( 8.385254915620292238, 90.00000000000000000, 8.679704431140114636E-16 ) ) ;
#1484=CARTESIAN_POINT ( 'NONE',  ( -15.29705854078139282, 46.06057977201469100, -2.036022158066717581E-15 ) ) ;
#1485=FACE_OUTER_BOUND ( 'NONE', #145, .T. ) ;
#1486=CARTESIAN_POINT ( 'NONE',  ( 3.913402758210908772, -81.93939393942487470, -9.205743832022209361 ) ) ;
#1487=DIRECTION ( 'NONE',  ( -1.000000000000000000, 0.000000000000000000, 0.000000000000000000 ) ) ;
#1489=CARTESIAN_POINT ( 'NONE',  ( 8.385254915620294014, 78.67828027274755698, 8.868043070384791430E-16 ) ) ;
#1490=ORIENTED_EDGE ( 'NONE', *, *, #11940, .F. ) ;
#1491=ORIENTED_EDGE ( 'NONE', *, *, #11278, .F. ) ;
#1493=CARTESIAN_POINT ( 'NONE',  ( 1.661059338047568001, -148.6780715075996966, -1.248219484669665924 ) ) ;
#1495=CARTESIAN_POINT ( 'NONE',  ( -6.036583442707799563, -95.60204248688987150, -5.530378780570661235 ) ) ;
#1496=CARTESIAN_POINT ( 'NONE',  ( 2.008006476061143353, -80.00378950643523979, 9.910921260988354575 ) ) ;
#1497=DIRECTION ( 'NONE',  ( -1.000000000000000000, -2.797435172181480534E-17, 0.000000000000000000 ) ) ;
#1501=VERTEX_POINT ( 'NONE', #1787 ) ;
#1509=CARTESIAN_POINT ( 'NONE',  ( -39.99999999999999289, 100.0000000000000000, 2.500000000000000000 ) ) ;
#1510=CARTESIAN_POINT ( 'NONE',  ( -8.385254915620297567, -6.144721277337256815, -2.041332847496538735E-15 ) ) ;
#1511=DIRECTION ( 'NONE',  ( 0.000000000000000000, 0.000000000000000000, 1.000000000000000000 ) ) ;
#1512=CARTESIAN_POINT ( 'NONE',  ( 8.385254915620290461, 53.02855864072483882, 9.722760835075755586E-16 ) ) ;
#1514=ORIENTED_EDGE ( 'NONE', *, *, #11143, .F. ) ;
#1515=CARTESIAN_POINT ( 'NONE',  ( 4.208314830452973609, -157.8181818182845007, 0.6624707635749896850 ) ) ;
#1517=CARTESIAN_POINT ( 'NONE',  ( -2.517691654963332357E-15, 90.00000000000000000, -1.589271161308885878E-16 ) ) ;
#1520=FACE_OUTER_BOUND ( 'NONE', #11031, .T. ) ;
#1522=CARTESIAN_POINT ( 'NONE',  ( -8.385254915620297567, -34.41905512736551032, -9.053393109928500416E-16 ) ) ;
#1523=ADVANCED_FACE ( 'NONE', ( #7899 ), #11140, .F. ) ;
#1526=B_SPLINE_CURVE_WITH_KNOTS ( 'NONE', 3,
 ( #1439, #481, #5716, #8954 ),
 .UNSPECIFIED., .F., .F.,
 ( 4, 4 ),
 ( 0.000000000000000000, 1.000000000000000000 ),
 .UNSPECIFIED. ) ;
#1527=AXIS2_PLACEMENT_3D ( 'NONE', #13455, #4995, #3801 ) ;
#1529=AXIS2_PLACEMENT_3D ( 'NONE', #5524, #10912, #4542 ) ;
#1531=LINE ( 'NONE', #5671, #12811 ) ;
#1533=CARTESIAN_POINT ( 'NONE',  ( 12.99553232110413781, 77.04820039461787928, 3.182987412051231773E-15 ) ) ;
#1537=CARTESIAN_POINT ( 'NONE',  ( 5.492103586168583185, -85.98458891577695340, -7.620002978679659478 ) ) ;
#1539=CARTESIAN_POINT ( 'NONE',  ( -12.99579180576516535, 16.95961992694555676, -3.214849374574138845E-15 ) ) ;
#1542=EDGE_LOOP ( 'NONE', ( #8607, #8080, #6527, #11183 ) ) ;
#1543=EDGE_CURVE ( 'NONE', #2454, #8513, #7588, .T. ) ;
#1546=CARTESIAN_POINT ( 'NONE',  ( 8.385254915620294014, -24.99427717735608212, 1.068716529980328543E-15 ) ) ;
#1549=CARTESIAN_POINT ( 'NONE',  ( 7.273479296210343392, -73.48250327241889579, 7.060675410516041417 ) ) ;
#1550=DIRECTION ( 'NONE',  ( -2.797435172181481150E-17, 1.000000000000000000, -1.765856845898762549E-18 ) ) ;
#1553=CARTESIAN_POINT ( 'NONE',  ( -0.4173931308523584627, -102.5454545454544615, 7.668730708677045982 ) ) ;
#1555=AXIS2_PLACEMENT_3D ( 'NONE', #329, #13101, #3459 ) ;
#1558=ORIENTED_EDGE ( 'NONE', *, *, #9619, .F. ) ;
#1559=AXIS2_PLACEMENT_3D ( 'NONE', #3456, #10956, #8717 ) ;
#1562=ORIENTED_EDGE ( 'NONE', *, *, #3110, .T. ) ;
#1565=CARTESIAN_POINT ( 'NONE',  ( 6.060518735590991746, -109.8459309627911864, -2.257746733285272089 ) ) ;
#1566=DIRECTION ( 'NONE',  ( 1.000000000000000000, 0.000000000000000000, 0.000000000000000000 ) ) ;
#1567=CARTESIAN_POINT ( 'NONE',  ( -15.29705854078138927, 29.09759144140119957, -5.138218104596347907E-17 ) ) ;
#1570=EDGE_LOOP ( 'NONE', ( #12242, #620, #13076, #12492 ) ) ;
#1571=ORIENTED_EDGE ( 'NONE', *, *, #3141, .T. ) ;
#1572=FACE_OUTER_BOUND ( 'NONE', #13487, .T. ) ;
#1575=AXIS2_PLACEMENT_3D ( 'NONE', #9277, #13660, #13796 ) ;
#1576=CIRCLE ( 'NONE', #9419, 8.385254915620294014 ) ;
#1577=DIRECTION ( 'NONE',  ( 0.000000000000000000, 0.000000000000000000, 1.000000000000000000 ) ) ;
#1583=VECTOR ( 'NONE', #8845, 1000.000000000000000 ) ;
#1586=AXIS2_PLACEMENT_3D ( 'NONE', #13102, #4376, #9715 ) ;
#1588=AXIS2_PLACEMENT_3D ( 'NONE', #13019, #2479, #12948 ) ;
#1589=CARTESIAN_POINT ( 'NONE',  ( 3.288118420601234604, 90.13403546913524167, 3.770150660886109950 ) ) ;
#1590=ORIENTED_EDGE ( 'NONE', *, *, #1191, .T. ) ;
#1591=CARTESIAN_POINT ( 'NONE',  ( 31.81818181818183433, 133.3608531424536920, 0.5000000000000000000 ) ) ;
#1597=CARTESIAN_POINT ( 'NONE',  ( 0.7140975576127237545, -124.8181818181821825, -13.04184819563892539 ) ) ;
#1599=AXIS2_PLACEMENT_3D ( 'NONE', #518, #12281, #372 ) ;
#1600=CARTESIAN_POINT ( 'NONE',  ( -1.552166912326615374E-15, 55.48535772202409078, -9.797919878057798703E-17 ) ) ;
#1601=CARTESIAN_POINT ( 'NONE',  ( -25.00000000000000355, 120.0000000000000284, 0.5000000000000000000 ) ) ;
#1603=CARTESIAN_POINT ( 'NONE',  ( -12.97449437267217931, -39.59556244224027211, 25.94898874534434796 ) ) ;
#1609=CARTESIAN_POINT ( 'NONE',  ( 15.29705854078139105, -36.87585420866476227, 1.980000072520086583E-15 ) ) ;
#1613=CARTESIAN_POINT ( 'NONE',  ( -2.517691654963332357E-15, 90.00000000000000000, -1.589271161308885878E-16 ) ) ;
#1614=CARTESIAN_POINT ( 'NONE',  ( 4.934221198804287667, -99.30322515911785786, 5.966777793213275061 ) ) ;
#1615=CARTESIAN_POINT ( 'NONE',  ( 8.385254915620295790, 50.40394642271930081, -16.77050983124058803 ) ) ;
#1618=CARTESIAN_POINT ( 'NONE',  ( -10.69346802281034847, -6.949821576306442594, -1.285027358575335329E-15 ) ) ;
#1620=CARTESIAN_POINT ( 'NONE',  ( 0.9052951019204806826, -80.99999999999998579, 10.12030223674823581 ) ) ;
#1622=FACE_OUTER_BOUND ( 'NONE', #13090, .T. ) ;
#1626=CARTESIAN_POINT ( 'NONE',  ( -10.69346802281034670, -16.37459952631584059, -2.593420296013165014E-15 ) ) ;
#1627=CARTESIAN_POINT ( 'NONE',  ( 9.841394828004627726, -91.60173160174092288, 2.396245945945958411 ) ) ;
#1629=CARTESIAN_POINT ( 'NONE',  ( -15.29705854078138927, 19.67281349139174296, -3.473937238186366113E-17 ) ) ;
#1630=AXIS2_PLACEMENT_3D ( 'NONE', #59, #7473, #10758 ) ;
#1631=DIRECTION ( 'NONE',  ( -1.000000000000000000, 0.000000000000000000, 0.000000000000000000 ) ) ;
#1633=VERTEX_POINT ( 'NONE', #2696 ) ;
#1634=ORIENTED_EDGE ( 'NONE', *, *, #12978, .F. ) ;
#1635=DIRECTION ( 'NONE',  ( -2.797435172181481150E-17, 1.000000000000000000, -1.765856845898762549E-18 ) ) ;
#1636=ORIENTED_EDGE ( 'NONE', *, *, #13462, .T. ) ;
#1637=CARTESIAN_POINT ( 'NONE',  ( 4.216390066750006937, -117.2395442519084128, 3.627621796832325884 ) ) ;
#1638=DIRECTION ( 'NONE',  ( -2.797435172181481150E-17, 1.000000000000000000, -1.765856845898762549E-18 ) ) ;
#1644=ORIENTED_EDGE ( 'NONE', *, *, #6867, .T. ) ;
#1646=ORIENTED_EDGE ( 'NONE', *, *, #2049, .T. ) ;
#1648=ADVANCED_FACE ( 'NONE', ( #9217 ), #8226, .T. ) ;
#1649=CARTESIAN_POINT ( 'NONE',  ( 3.709034887389476509, -132.4786972693144662, -0.6210620215803320798 ) ) ;
#1650=CARTESIAN_POINT ( 'NONE',  ( 4.330127018922190985, 91.86461561432780343, -2.500000000000000000 ) ) ;
#1654=EDGE_CURVE ( 'NONE', #2621, #3550, #8315, .T. ) ;
#1655=CARTESIAN_POINT ( 'NONE',  ( 15.29705854078139105, 19.67281349139174296, 1.840275709580740132E-15 ) ) ;
#1668=CARTESIAN_POINT ( 'NONE',  ( -10.82118823930625418, -118.2727272727264420, -9.720764081409949853 ) ) ;
#1671=CARTESIAN_POINT ( 'NONE',  ( -10.69381717166375623, -21.56444287793185666, -1.233455458826524398E-15 ) ) ;
#1674=CARTESIAN_POINT ( 'NONE',  ( 9.115242562766566081, -73.26725376456661820, 4.373789808026823600 ) ) ;
#1675=CIRCLE ( 'NONE', #2788, 8.385254915620292238 ) ;
#1676=ORIENTED_EDGE ( 'NONE', *, *, #1120, .F. ) ;
#1677=ORIENTED_EDGE ( 'NONE', *, *, #2791, .T. ) ;
#1678=CARTESIAN_POINT ( 'NONE',  ( -1.210348956774063511, -80.16702553641545137, 10.05366391452042230 ) ) ;
#1679=EDGE_LOOP ( 'NONE', ( #10985, #3054, #7344, #7916 ) ) ;
#1681=CIRCLE ( 'NONE', #1227, 8.385254915620290461 ) ;
#1682=DIRECTION ( 'NONE',  ( -1.000000000000000000, 0.000000000000000000, 0.000000000000000000 ) ) ;
#1686=CARTESIAN_POINT ( 'NONE',  ( 7.892147093659925616, -89.25378073177839156, -4.277061995178171649 ) ) ;
#1687=FACE_OUTER_BOUND ( 'NONE', #8643, .T. ) ;
#1692=CARTESIAN_POINT ( 'NONE',  ( 25.00000000000000355, 120.0000000000000284, -0.5000000000000000000 ) ) ;
#1693=CARTESIAN_POINT ( 'NONE',  ( 6.726204760714201925, -75.54545454545360883, 7.481082188384250209 ) ) ;
#1695=CARTESIAN_POINT ( 'NONE',  ( 2.255225228351934952, -77.73185732064989395, 9.851628683897507344 ) ) ;
#1696=( NAMED_UNIT ( * ) PLANE_ANGLE_UNIT ( ) SI_UNIT ( $, .RADIAN. ) );
#1699=CARTESIAN_POINT ( 'NONE',  ( 1.423465862495751466, -128.7272727272806492, -3.918423281948167691 ) ) ;
#1701=CARTESIAN_POINT ( 'NONE',  ( 15.29705854078138749, 76.22148119144830503, 1.740418857596140842E-15 ) ) ;
#1703=CARTESIAN_POINT ( 'NONE',  ( 1.958204620527036497E-15, -70.00000000000000000, 1.236099792129133461E-16 ) ) ;
#1705=VERTEX_POINT ( 'NONE', #7772 ) ;
#1706=EDGE_CURVE ( 'NONE', #3550, #2621, #11671, .T. ) ;
#1709=ORIENTED_EDGE ( 'NONE', *, *, #11756, .F. ) ;
#1710=CARTESIAN_POINT ( 'NONE',  ( -5.391851710260636921, -96.31036116225249089, -6.045474291746966600 ) ) ;
#1712=DIRECTION ( 'NONE',  ( -2.797435172181481150E-17, 1.000000000000000000, -1.765856845898762549E-18 ) ) ;
#1714=VERTEX_POINT ( 'NONE', #8912 ) ;
#1716=CARTESIAN_POINT ( 'NONE',  ( 0.1852016367012860043, -160.0000000000003126, -1.488522876466233713 ) ) ;
#1717=CARTESIAN_POINT ( 'NONE',  ( 4.355466475183198247E-16, -15.56949922734665570, 2.749350679782564022E-17 ) ) ;
#1718=DIRECTION ( 'NONE',  ( -2.797435172181481150E-17, 1.000000000000000000, -1.765856845898762549E-18 ) ) ;
#1722=DIRECTION ( 'NONE',  ( 0.000000000000000000, 0.000000000000000000, 1.000000000000000000 ) ) ;
#1725=ADVANCED_FACE ( 'NONE', ( #12062 ), #3294, .T. ) ;
#1727=VERTEX_POINT ( 'NONE', #13780 ) ;
#1733=PLANE ( 'NONE',  #1445 ) ;
#1734=CARTESIAN_POINT ( 'NONE',  ( 35.20000000000001705, 106.4000000000000199, -2.500000000000000000 ) ) ;
#1738=CARTESIAN_POINT ( 'NONE',  ( 12.99553232110413425, 20.49953269456136695, 25.99106464220827917 ) ) ;
#1739=CARTESIAN_POINT ( 'NONE',  ( -4.330127018922195425, 92.00000000000000000, 2.500000000000000000 ) ) ;
#1741=EDGE_CURVE ( 'NONE', #283, #13516, #1152, .T. ) ;
#1743=CARTESIAN_POINT ( 'NONE',  ( -6.938012361950032236, -85.09891028704761595, 6.468549380687601769 ) ) ;
#1745=VERTEX_POINT ( 'NONE', #13053 ) ;
#1748=CARTESIAN_POINT ( 'NONE',  ( -1.815818965600183303E-15, 64.91013567203349055, -1.146220074446778111E-16 ) ) ;
#1749=CARTESIAN_POINT ( 'NONE',  ( -4.752793807721118924, -119.4346283814399499, -2.305654517533438419 ) ) ;
#1757=CARTESIAN_POINT ( 'NONE',  ( 10.03938689678732032, -69.87878787879145648, 0.2267434780641480463 ) ) ;
#1759=CARTESIAN_POINT ( 'NONE',  ( 4.961404791891397714, 89.99999999999998579, 0.6346456166747422856 ) ) ;
#1762=CARTESIAN_POINT ( 'NONE',  ( -8.355983821213438745, -73.45454545935436386, -17.50953411596619702 ) ) ;
#1764=DIRECTION ( 'NONE',  ( -2.797435172181481150E-17, 1.000000000000000000, -1.765856845898762549E-18 ) ) ;
#1768=CIRCLE ( 'NONE', #12538, 8.385254915620294014 ) ;
#1779=DIRECTION ( 'NONE',  ( -2.797435172181481150E-17, 1.000000000000000000, -1.765856845898762549E-18 ) ) ;
#1780=CARTESIAN_POINT ( 'NONE',  ( 12.99553232110414491, 1.649976794542512559, 1.591673766201862918E-15 ) ) ;
#1787=CARTESIAN_POINT ( 'NONE',  ( 36.36363636363638108, 142.2680885707561629, 0.5000000000000000000 ) ) ;
#1788=AXIS2_PLACEMENT_3D ( 'NONE', #11891, #1242, #9791 ) ;
#1789=ORIENTED_EDGE ( 'NONE', *, *, #1139, .F. ) ;
#1792=DIRECTION ( 'NONE',  ( -2.797435172181481150E-17, 1.000000000000000000, -1.765856845898762549E-18 ) ) ;
#1793=CARTESIAN_POINT ( 'NONE',  ( 10.69346802281034314, 59.02362407375952102, 0.000000000000000000 ) ) ;
#1795=CARTESIAN_POINT ( 'NONE',  ( 3.469499284126810856, -73.45454542565497036, 20.14723442872987746 ) ) ;
#1796=ADVANCED_FACE ( 'NONE', ( #6924 ), #8146, .T. ) ;
#1797=CARTESIAN_POINT ( 'NONE',  ( -15.29705854078139282, 36.63580182200523438, -3.809726632991057923E-15 ) ) ;
#1798=VECTOR ( 'NONE', #9395, 1000.000000000000000 ) ;
#1799=CARTESIAN_POINT ( 'NONE',  ( 8.385254915620288685, 5.904668890677672088, 16.77050983124058448 ) ) ;
#1800=DIRECTION ( 'NONE',  ( 0.000000000000000000, 0.000000000000000000, 1.000000000000000000 ) ) ;
#1801=CIRCLE ( 'NONE', #484, 15.29705854078138749 ) ;
#1805=VERTEX_POINT ( 'NONE', #2434 ) ;
#1806=VERTEX_POINT ( 'NONE', #11144 ) ;
#1807=AXIS2_PLACEMENT_3D ( 'NONE', #12317, #10067, #2910 ) ;
#1813=PLANE ( 'NONE',  #2040 ) ;
#1814=EDGE_CURVE ( 'NONE', #2160, #10681, #6742, .T. ) ;
#1815=CARTESIAN_POINT ( 'NONE',  ( 12.99553232110414491, 29.92431064457076673, -25.99106464220827561 ) ) ;
#1817=CARTESIAN_POINT ( 'NONE',  ( -10.69346802281034670, 59.02362407375952102, -1.518026679872732817E-15 ) ) ;
#1818=EDGE_CURVE ( 'NONE', #6908, #9709, #1234, .T. ) ;
#1820=CARTESIAN_POINT ( 'NONE',  ( -0.009804802457270511001, -127.8804227454992457, -4.311392792372593874 ) ) ;
#1821=DIRECTION ( 'NONE',  ( 0.1234677578012386701, 0.000000000000000000, -0.9923485843107424653 ) ) ;
#1822=( BOUNDED_SURFACE ( )  B_SPLINE_SURFACE ( 3, 3, ( 
 ( #4284, #9559, #11790, #11524 ),
 ( #11593, #8435, #13868, #4215 ),
 ( #5137, #6465, #12793, #10667 ),
 ( #10729, #1148, #1982, #13669 ) ),
 .UNSPECIFIED., .F., .F., .T. ) 
 B_SPLINE_SURFACE_WITH_KNOTS ( ( 4, 4 ),
 ( 4, 4 ),
 ( 0.000000000000000000, 1.000000000000000000 ),
 ( 0.000000000000000000, 1.000000000000000000 ),
 .UNSPECIFIED. ) 
 GEOMETRIC_REPRESENTATION_ITEM ( )  RATIONAL_B_SPLINE_SURFACE ( (
 ( 1.000000000000000000, 0.3333333333333334259, 0.3333333333333334259, 1.000000000000000000),
 ( 1.000000000000000000, 0.3333333333333334259, 0.3333333333333334259, 1.000000000000000000),
 ( 1.000000000000000000, 0.3333333333333334259, 0.3333333333333334259, 1.000000000000000000),
 ( 1.000000000000000000, 0.3333333333333334259, 0.3333333333333334259, 1.000000000000000000) ) ) 
 REPRESENTATION_ITEM ( '' )  SURFACE ( )  );
#1825=ORIENTED_EDGE ( 'NONE', *, *, #6988, .T. ) ;
#1826=ORIENTED_EDGE ( 'NONE', *, *, #375, .F. ) ;
#1828=ORIENTED_EDGE ( 'NONE', *, *, #5654, .T. ) ;
#1830=EDGE_CURVE ( 'NONE', #2958, #4633, #7853, .T. ) ;
#1832=CARTESIAN_POINT ( 'NONE',  ( -14.13596196814456718, -39.17949320881311337, -28.27192393628914502 ) ) ;
#1834=CARTESIAN_POINT ( 'NONE',  ( 12.99553232110413958, 11.07475474455194053, 0.000000000000000000 ) ) ;
#1838=ADVANCED_FACE ( 'NONE', ( #11285 ), #9653, .T. ) ;
#1840=CARTESIAN_POINT ( 'NONE',  ( -0.1372443476013192609, -156.3093790477994958, -1.553728524142399037 ) ) ;
#1841=FACE_OUTER_BOUND ( 'NONE', #213, .T. ) ;
#1846=CARTESIAN_POINT ( 'NONE',  ( -15.29705854078138927, 38.52236939141059935, 30.59411708156276433 ) ) ;
#1847=ORIENTED_EDGE ( 'NONE', *, *, #4187, .T. ) ;
#1849=CARTESIAN_POINT ( 'NONE',  ( -4.684139815134829021, -116.4556953340202909, -3.176431292803267414 ) ) ;
#1854=CARTESIAN_POINT ( 'NONE',  ( 15.29705854078138394, 29.09759144140119957, 30.59411708156277854 ) ) ;
#1856=DIRECTION ( 'NONE',  ( -0.000000000000000000, -0.000000000000000000, -1.000000000000000000 ) ) ;
#1863=ORIENTED_EDGE ( 'NONE', *, *, #8017, .T. ) ;
#1864=CARTESIAN_POINT ( 'NONE',  ( -8.385254915620295790, -12.94488700934118341, 16.77050983124058448 ) ) ;
#1871=CARTESIAN_POINT ( 'NONE',  ( 3.606245374316391583, -157.8181818183015821, -2.267989313183790934 ) ) ;
#1872=VECTOR ( 'NONE', #5601, 1000.000000000000000 ) ;
#1874=CARTESIAN_POINT ( 'NONE',  ( 10.00000000000000000, 92.00000000000000000, 2.500000000000000000 ) ) ;
#1875=CARTESIAN_POINT ( 'NONE',  ( -10.00000000000000711, 139.9999999999999716, 2.500000000000000000 ) ) ;
#1876=CARTESIAN_POINT ( 'NONE',  ( -4.942648287111191863, 90.01344868170882307, 0.7664870281642331973 ) ) ;
#1879=( BOUNDED_SURFACE ( )  B_SPLINE_SURFACE ( 3, 3, ( 
 ( #5558, #326, #9711, #4582 ),
 ( #10883, #3255, #10684, #7529 ),
 ( #12019, #1293, #4509, #7466 ),
 ( #7735, #11810, #13100, #8867 ) ),
 .UNSPECIFIED., .F., .F., .T. ) 
 B_SPLINE_SURFACE_WITH_KNOTS ( ( 4, 4 ),
 ( 4, 4 ),
 ( 0.000000000000000000, 1.000000000000000000 ),
 ( 0.000000000000000000, 1.000000000000000000 ),
 .UNSPECIFIED. ) 
 GEOMETRIC_REPRESENTATION_ITEM ( )  RATIONAL_B_SPLINE_SURFACE ( (
 ( 1.000000000000000000, 0.3333333333333334259, 0.3333333333333334259, 1.000000000000000000),
 ( 1.000000000000000000, 0.3333333333333334259, 0.3333333333333334259, 1.000000000000000000),
 ( 1.000000000000000000, 0.3333333333333334259, 0.3333333333333334259, 1.000000000000000000),
 ( 1.000000000000000000, 0.3333333333333334259, 0.3333333333333334259, 1.000000000000000000) ) ) 
 REPRESENTATION_ITEM ( '' )  SURFACE ( )  );
#1880=CARTESIAN_POINT ( 'NONE',  ( -6.798205150802573371, -84.93498744380758581, 6.637038377984636917 ) ) ;
#1885=FACE_OUTER_BOUND ( 'NONE', #3585, .T. ) ;
#1886=CARTESIAN_POINT ( 'NONE',  ( 2.435310979999304237, -143.3834574191564002, 0.8240421561592208288 ) ) ;
#1887=DIRECTION ( 'NONE',  ( -0.8000000000000008216, 0.5999999999999988676, 0.000000000000000000 ) ) ;
#1889=EDGE_CURVE ( 'NONE', #12845, #7874, #12943, .T. ) ;
#1890=VERTEX_POINT ( 'NONE', #462 ) ;
#1894=CIRCLE ( 'NONE', #9727, 8.385254915620295790 ) ;
#1901=ORIENTED_EDGE ( 'NONE', *, *, #2761, .F. ) ;
#1903=CARTESIAN_POINT ( 'NONE',  ( -9.846850911399156914, -91.60173160168641004, 0.3733502116265231541 ) ) ;
#1904=CARTESIAN_POINT ( 'NONE',  ( -8.385254915620292238, 43.60378069071538221, 16.77050983124057382 ) ) ;
#1905=( BOUNDED_SURFACE ( )  B_SPLINE_SURFACE ( 3, 3, ( 
 ( #3089, #10521, #5195, #13790 ),
 ( #6319, #996, #9549, #12781 ),
 ( #10656, #9611, #16, #12854 ),
 ( #3220, #6802, #10781, #2301 ) ),
 .UNSPECIFIED., .F., .F., .T. ) 
 B_SPLINE_SURFACE_WITH_KNOTS ( ( 4, 4 ),
 ( 4, 4 ),
 ( 0.000000000000000000, 1.000000000000000000 ),
 ( 0.000000000000000000, 1.000000000000000000 ),
 .UNSPECIFIED. ) 
 GEOMETRIC_REPRESENTATION_ITEM ( )  RATIONAL_B_SPLINE_SURFACE ( (
 ( 1.000000000000000000, 0.3333333333333334259, 0.3333333333333334259, 1.000000000000000000),
 ( 1.000000000000000000, 0.3333333333333334259, 0.3333333333333334259, 1.000000000000000000),
 ( 1.000000000000000000, 0.3333333333333334259, 0.3333333333333334259, 1.000000000000000000),
 ( 1.000000000000000000, 0.3333333333333334259, 0.3333333333333334259, 1.000000000000000000) ) ) 
 REPRESENTATION_ITEM ( '' )  SURFACE ( )  );
#1907=CARTESIAN_POINT ( 'NONE',  ( 2.678949786664373445, -123.4179834144425740, 4.050618884325445812 ) ) ;
#1909=CIRCLE ( 'NONE', #11972, 48.00000000000001421 ) ;
#1910=ORIENTED_EDGE ( 'NONE', *, *, #9040, .T. ) ;
#1911=ORIENTED_EDGE ( 'NONE', *, *, #6137, .T. ) ;
#1914=EDGE_CURVE ( 'NONE', #8462, #8344, #10106, .T. ) ;
#1918=CARTESIAN_POINT ( 'NONE',  ( 3.127593042865025375, -81.56118865055866252, -9.358713454693210920 ) ) ;
#1919=CARTESIAN_POINT ( 'NONE',  ( 0.3237100442286745539, -158.0606060622567668, 0.5247744424694577026 ) ) ;
#1923=CYLINDRICAL_SURFACE ( 'NONE', #1038, 8.385254915620292238 ) ;
#1924=CYLINDRICAL_SURFACE ( 'NONE', #7839, 15.29705854078139105 ) ;
#1927=CIRCLE ( 'NONE', #6627, 5.000000000000000000 ) ;
#1929=VERTEX_POINT ( 'NONE', #9140 ) ;
#1930=DIRECTION ( 'NONE',  ( -2.797435172181481150E-17, 1.000000000000000000, -1.765856845898762549E-18 ) ) ;
#1932=CARTESIAN_POINT ( 'NONE',  ( 2.710744138662893210, -134.9675367765264582, -2.173820228074841321 ) ) ;
#1933=CARTESIAN_POINT ( 'NONE',  ( -3.867425345466811493, -111.7272727272759454, 3.383301718857328666 ) ) ;
#1934=AXIS2_PLACEMENT_3D ( 'NONE', #9679, #7434, #6389 ) ;
#1936=ORIENTED_EDGE ( 'NONE', *, *, #5084, .F. ) ;
#1938=ORIENTED_EDGE ( 'NONE', *, *, #6260, .F. ) ;
#1941=CARTESIAN_POINT ( 'NONE',  ( 8.012933684613601670, -76.12121211522740793, 3.597289648239124116 ) ) ;
#1942=CARTESIAN_POINT ( 'NONE',  ( 2.503528417663046124, -105.1818181818193096, -12.81920766435407089 ) ) ;
#1943=CARTESIAN_POINT ( 'NONE',  ( -8.385254915620299343, 50.40394642271930081, 16.77050983124058803 ) ) ;
#1944=DIRECTION ( 'NONE',  ( -0.5999999999999966471, 0.8000000000000024869, 0.000000000000000000 ) ) ;
#1948=EDGE_CURVE ( 'NONE', #2799, #11270, #12812, .T. ) ;
#1949=ORIENTED_EDGE ( 'NONE', *, *, #816, .F. ) ;
#1950=CARTESIAN_POINT ( 'NONE',  ( 12.99579180576517778, -20.73949187309215247, -25.99158361153034136 ) ) ;
#1952=EDGE_CURVE ( 'NONE', #849, #717, #5857, .T. ) ;
#1955=CARTESIAN_POINT ( 'NONE',  ( 0.3217016761801410052, -154.7285720644513844, 1.606987287732108527 ) ) ;
#1956=CARTESIAN_POINT ( 'NONE',  ( 12.99553232110413958, 48.77386654458962312, 1.520979731354686344E-15 ) ) ;
#1957=ORIENTED_EDGE ( 'NONE', *, *, #5433, .T. ) ;
#1958=ORIENTED_EDGE ( 'NONE', *, *, #3431, .T. ) ;
#1959=EDGE_LOOP ( 'NONE', ( #2546, #8274, #1644, #8029 ) ) ;
#1963=CARTESIAN_POINT ( 'NONE',  ( 8.385254915620294014, 78.67828027274755698, 9.540301975042864801E-16 ) ) ;
#1964=EDGE_LOOP ( 'NONE', ( #10298, #4928, #5699, #8290 ) ) ;
#1967=CARTESIAN_POINT ( 'NONE',  ( 32.72727272727274084, 135.1423002281142089, 0.5000000000000000000 ) ) ;
#1970=CARTESIAN_POINT ( 'NONE',  ( -10.82460162405759263, -71.99999999999995737, -2.658570984655005631 ) ) ;
#1972=FACE_OUTER_BOUND ( 'NONE', #6824, .T. ) ;
#1973=CARTESIAN_POINT ( 'NONE',  ( -1.819570364555604502, -146.4201944892890879, -1.378504945579682062 ) ) ;
#1974=EDGE_CURVE ( 'NONE', #887, #3550, #3586, .T. ) ;
#1975=FACE_OUTER_BOUND ( 'NONE', #9275, .T. ) ;
#1980=CIRCLE ( 'NONE', #6906, 8.385254915620294014 ) ;
#1982=CARTESIAN_POINT ( 'NONE',  ( -15.29705854078138216, 38.52236939141059935, -30.59411708156276788 ) ) ;
#1983=CARTESIAN_POINT ( 'NONE',  ( -5.313449998973543309, -115.2025049533512799, -2.323891416253867082 ) ) ;
#1985=CARTESIAN_POINT ( 'NONE',  ( -0.7701066202684672124, -168.0000000000000568, -1.909695209560596796 ) ) ;
#1987=EDGE_CURVE ( 'NONE', #10906, #7855, #6496, .T. ) ;
#1988=DIRECTION ( 'NONE',  ( -0.000000000000000000, -0.000000000000000000, -1.000000000000000000 ) ) ;
#1989=CARTESIAN_POINT ( 'NONE',  ( -12.99553232110413781, 1.649976794542511671, -25.99106464220828627 ) ) ;
#1993=CARTESIAN_POINT ( 'NONE',  ( -8.385254915620294014, 59.82872437272870769, -1.056489625149731375E-16 ) ) ;
#1994=EDGE_CURVE ( 'NONE', #13048, #8282, #10954, .T. ) ;
#1995=CARTESIAN_POINT ( 'NONE',  ( 11.81226048336477064, -40.00941361824963849, 0.000000000000000000 ) ) ;
#1996=CARTESIAN_POINT ( 'NONE',  ( -15.29705854078139282, 90.00000000000000000, -1.589271161308885878E-16 ) ) ;
#1998=CARTESIAN_POINT ( 'NONE',  ( -0.01432886326384079194, -82.89610389603521412, -5.147384767215601009 ) ) ;
#2000=FACE_OUTER_BOUND ( 'NONE', #12656, .T. ) ;
#2003=LINE ( 'NONE', #6284, #3458 ) ;
#2007=ADVANCED_FACE ( 'NONE', ( #10967 ), #8662, .F. ) ;
#2008=CARTESIAN_POINT ( 'NONE',  ( -4.560784247219692666, -95.36363636362557372, -0.7586904865638435247 ) ) ;
#2009=EDGE_CURVE ( 'NONE', #9777, #13779, #6942, .T. ) ;
#2010=CARTESIAN_POINT ( 'NONE',  ( -2.517691654963332357E-15, 90.00000000000000000, -1.589271161308885878E-16 ) ) ;
#2011=CARTESIAN_POINT ( 'NONE',  ( -4.769534092270762748, 90.26591089801031842, 1.504791211541889329 ) ) ;
#2013=ORIENTED_EDGE ( 'NONE', *, *, #7115, .T. ) ;
#2016=CARTESIAN_POINT ( 'NONE',  ( -15.29705854078139282, -10.48808792804187284, -3.755586217998579266E-15 ) ) ;
#2020=CARTESIAN_POINT ( 'NONE',  ( 15.29705854078138927, 29.09759144140119957, 1.823632900916640480E-15 ) ) ;
#2021=CARTESIAN_POINT ( 'NONE',  ( -8.385254915620292238, -3.520109059331755663, -2.049896454535566708E-15 ) ) ;
#2022=DIRECTION ( 'NONE',  ( -1.000000000000000000, 0.000000000000000000, 0.000000000000000000 ) ) ;
#2027=DIRECTION ( 'NONE',  ( -0.000000000000000000, -0.000000000000000000, -1.000000000000000000 ) ) ;
#2028=AXIS2_PLACEMENT_3D ( 'NONE', #1362, #5641, #7963 ) ;
#2030=ORIENTED_EDGE ( 'NONE', *, *, #10110, .T. ) ;
#2031=CARTESIAN_POINT ( 'NONE',  ( -2.771542151761396955, 90.01585036846415733, -4.174539845741943367 ) ) ;
#2039=CARTESIAN_POINT ( 'NONE',  ( -9.412634226148453465, -72.00000000000004263, -5.970118669234189213 ) ) ;
#2040=AXIS2_PLACEMENT_3D ( 'NONE', #8201, #4116, #12482 ) ;
#2044=CARTESIAN_POINT ( 'NONE',  ( -0.6071592415733604309, -152.6372033014571343, -1.642897721265916822 ) ) ;
#2047=ORIENTED_EDGE ( 'NONE', *, *, #9173, .T. ) ;
#2048=VERTEX_POINT ( 'NONE', #4517 ) ;
#2049=EDGE_CURVE ( 'NONE', #11046, #11768, #7829, .T. ) ;
#2050=CARTESIAN_POINT ( 'NONE',  ( -0.5594493140154206401, -142.1330619314459796, -2.638491898088323850 ) ) ;
#2051=VECTOR ( 'NONE', #7783, 1000.000000000000000 ) ;
#2053=DIRECTION ( 'NONE',  ( -2.797435172181481150E-17, 1.000000000000000000, -1.765856845898762549E-18 ) ) ;
#2054=CARTESIAN_POINT ( 'NONE',  ( -3.914066993105319359, -117.7082033709801578, -3.866271586310865871 ) ) ;
#2056=DIRECTION ( 'NONE',  ( 1.000000000000000000, 0.000000000000000000, 0.000000000000000000 ) ) ;
#2058=DIRECTION ( 'NONE',  ( -2.797435172181481150E-17, 1.000000000000000000, -1.765856845898762549E-18 ) ) ;
#2068=ADVANCED_FACE ( 'NONE', ( #337 ), #4594, .T. ) ;
#2073=DIRECTION ( 'NONE',  ( -2.797435172181481150E-17, 1.000000000000000000, -1.765856845898762549E-18 ) ) ;
#2074=CARTESIAN_POINT ( 'NONE',  ( 2.518175769240307726, -124.8181818181797240, 12.81633841918553607 ) ) ;
#2077=DIRECTION ( 'NONE',  ( -1.000000000000000000, 0.000000000000000000, 0.000000000000000000 ) ) ;
#2078=DIRECTION ( 'NONE',  ( -2.797435172181481150E-17, 1.000000000000000000, -1.765856845898762549E-18 ) ) ;
#2079=DIRECTION ( 'NONE',  ( -2.797435172181479917E-17, 1.000000000000000000, -1.765856845898779112E-18 ) ) ;
#2082=EDGE_CURVE ( 'NONE', #6129, #4849, #10611, .T. ) ;
#2083=VERTEX_POINT ( 'NONE', #6275 ) ;
#2084=CARTESIAN_POINT ( 'NONE',  ( -8.385254915620292238, 43.60378069071538221, -2.162292655033656152E-15 ) ) ;
#2086=CARTESIAN_POINT ( 'NONE',  ( -12.99553232110413425, 29.92431064457076673, -25.99106464220827917 ) ) ;
#2087=CARTESIAN_POINT ( 'NONE',  ( -3.164093685572913817, -79.18419798644474383, -9.628149054438361887 ) ) ;
#2088=CARTESIAN_POINT ( 'NONE',  ( -1.070382723972096883, -126.0551519452116622, -4.385908996712817753 ) ) ;
#2098=CARTESIAN_POINT ( 'NONE',  ( 15.29705854078139282, 90.00000000000000000, 1.714422261702873160E-15 ) ) ;
#2099=CIRCLE ( 'NONE', #9723, 14.99999999999998934 ) ;
#2100=DIRECTION ( 'NONE',  ( -2.797435172181481150E-17, 1.000000000000000000, -1.765856845898762549E-18 ) ) ;
#2101=CARTESIAN_POINT ( 'NONE',  ( 8.385254915620290461, 62.45333659073423860, 9.189312520034297072E-16 ) ) ;
#2104=CARTESIAN_POINT ( 'NONE',  ( 1.032204844967210100, -126.1190415558569526, 4.386694312918715255 ) ) ;
#2105=CARTESIAN_POINT ( 'NONE',  ( -25.00000000000000355, 120.0000000000000284, 0.5000000000000000000 ) ) ;
#2106=ORIENTED_EDGE ( 'NONE', *, *, #13434, .F. ) ;
#2108=VERTEX_POINT ( 'NONE', #12877 ) ;
#2110=CARTESIAN_POINT ( 'NONE',  ( 10.69346802281034492, 40.17406817374066463, 2.619144277183853160E-15 ) ) ;
#2113=CARTESIAN_POINT ( 'NONE',  ( -3.926155785508803397, -105.6048756127474633, 5.752462641596377324 ) ) ;
#2114=CARTESIAN_POINT ( 'NONE',  ( -2.889799813501109593, -137.4545454546409360, -1.105612428328569763 ) ) ;
#2118=CARTESIAN_POINT ( 'NONE',  ( -3.711366765501976861, -78.09090909091068511, -9.373274001092186225 ) ) ;
#2120=DIRECTION ( 'NONE',  ( -5.551115123125776539E-17, 1.000000000000000000, 3.944304526105059027E-31 ) ) ;
#2125=CARTESIAN_POINT ( 'NONE',  ( -3.915768125667399957, -76.35064935077906512, -2.796074470126640676 ) ) ;
#2126=AXIS2_PLACEMENT_3D ( 'NONE', #12074, #3656, #1339 ) ;
#2128=DIRECTION ( 'NONE',  ( -2.797435172181481150E-17, 1.000000000000000000, -1.765856845898762549E-18 ) ) ;
#2133=CARTESIAN_POINT ( 'NONE',  ( 15.29705854078138927, 0.8232575913729167638, 30.59411708156278564 ) ) ;
#2134=CARTESIAN_POINT ( 'NONE',  ( 57.42880470118691250, -62.63636363331826118, 5.311255545704360870 ) ) ;
#2137=CARTESIAN_POINT ( 'NONE',  ( 15.29705854078139105, 27.21102387199583816, 1.823632900916640874E-15 ) ) ;
#2139=AXIS2_PLACEMENT_3D ( 'NONE', #4273, #7562, #7497 ) ;
#2141=DIRECTION ( 'NONE',  ( 1.000000000000000000, 0.000000000000000000, 0.000000000000000000 ) ) ;
#2148=ORIENTED_EDGE ( 'NONE', *, *, #5469, .F. ) ;
#2149=CARTESIAN_POINT ( 'NONE',  ( -2.517691654963332357E-15, 90.00000000000000000, -1.589271161308885878E-16 ) ) ;
#2150=EDGE_CURVE ( 'NONE', #7666, #1714, #11208, .T. ) ;
#2152=CARTESIAN_POINT ( 'NONE',  ( -9.723082549030324984, -72.03366437468082495, -2.708544034036612924 ) ) ;
#2154=CIRCLE ( 'NONE', #8881, 16.99999999999998934 ) ;
#2159=B_SPLINE_SURFACE_WITH_KNOTS ( 'NONE', 3, 3, ( 
 ( #10359, #10082, #495, #4758, #3692, #3836, #9033, #6916, #7128, #12544, #1597, #1668, #13346, #627, #6017, #7981, #563, #12259, #8121, #5953, #11403, #2646, #11203, #8186 ),
 ( #8047, #12404, #10224, #4888, #2792, #6085, #12330, #2720, #7058, #11340, #691, #4960, #12742, #3119, #3059, #8454, #8520, #7469, #5356, #11478, #6422, #53, #5162, #6158 ),
 ( #10427, #13696, #5224, #2923, #1871, #891, #9451, #9511, #4040, #9646, #6226, #3190, #12615, #13823, #11546, #2008, #962, #4170, #830, #7397, #11747, #10560, #8323, #7197 ),
 ( #8590, #5096, #9379, #11678, #7328, #10620, #2991, #1031, #4309, #7262, #2074, #6351, #6287, #1942, #13757, #10489, #11611, #4106, #5295, #12680, #9576, #13887, #2134, #4236 ) ),
 .UNSPECIFIED., .F., .F., .F.,
 ( 4, 4 ),
 ( 4, 1, 1, 1, 1, 1, 1, 1, 1, 1, 1, 1, 1, 1, 1, 1, 1, 1, 1, 1, 1, 4 ),
 ( -0.002000000000000000475, 0.02200000000000000566 ),
 ( -0.009000000000000030545, -0.004090909090909119854, -2.775557561562891043E-17, 0.0008181818181817908375, 0.005727272727272700661, 0.01250649350649347610, 0.02045454545454543360, 0.02536363636363634516, 0.03027272727272725672, 0.03518181818181816828, 0.04009090909090907984, 0.04990909090909089602, 0.05481818181818180757, 0.05972727272727271913, 0.06463636363636363069, 0.06954545454545453531, 0.07749350649350648934, 0.08427272727272726305, 0.08918181818181818155, 0.08999999999999998279, 0.09409090909090908617, 0.09900000000000000466 ),
 .UNSPECIFIED. ) ;
#2160=VERTEX_POINT ( 'NONE', #2265 ) ;
#2168=DIRECTION ( 'NONE',  ( 2.797435172181479917E-17, -1.000000000000000000, 1.765856845898779112E-18 ) ) ;
#2170=CARTESIAN_POINT ( 'NONE',  ( -8.481997772293230042, -90.97423660740879825, 2.267516047978543448 ) ) ;
#2179=CARTESIAN_POINT ( 'NONE',  ( 10.69381717166375623, -2.714886977913000266, 2.619229793989003951E-15 ) ) ;
#2180=CARTESIAN_POINT ( 'NONE',  ( 8.385254915620292238, 5.904668890677672088, 1.018788103988028800E-15 ) ) ;
#2183=CARTESIAN_POINT ( 'NONE',  ( -1.652786589945713258, -148.3982683983876711, -1.815848636689608053 ) ) ;
#2184=DIRECTION ( 'NONE',  ( 0.4545454545454531425, -0.8907235428302472391, 0.000000000000000000 ) ) ;
#2185=DIRECTION ( 'NONE',  ( -2.797435172181481150E-17, 1.000000000000000000, -1.765856845898762549E-18 ) ) ;
#2186=CARTESIAN_POINT ( 'NONE',  ( -9.849330193486526497, -69.00000000000014211, -1.830547125266440034 ) ) ;
#2189=AXIS2_PLACEMENT_3D ( 'NONE', #12295, #455, #9208 ) ;
#2195=CARTESIAN_POINT ( 'NONE',  ( 10.00000000000000711, 139.9999999999999716, -2.500000000000000000 ) ) ;
#2196=EDGE_LOOP ( 'NONE', ( #5799, #7876, #226, #10586 ) ) ;
#2198=DIRECTION ( 'NONE',  ( -1.000000000000000000, 0.000000000000000000, 0.000000000000000000 ) ) ;
#2199=CIRCLE ( 'NONE', #11610, 16.99999999999998934 ) ;
#2200=CARTESIAN_POINT ( 'NONE',  ( 10.69346802281034847, 2.474956373702985601, 2.619144277183853949E-15 ) ) ;
#2201=DIRECTION ( 'NONE',  ( -2.797435172181481150E-17, 1.000000000000000000, -1.765856845898762549E-18 ) ) ;
#2202=CIRCLE ( 'NONE', #2886, 15.29705854078139460 ) ;
#2204=CARTESIAN_POINT ( 'NONE',  ( 8.385254915620294014, 12.70483462268159869, 1.017890798515799537E-15 ) ) ;
#2207=LINE ( 'NONE', #2282, #8267 ) ;
#2211=EDGE_CURVE ( 'NONE', #5518, #3968, #1124, .T. ) ;
#2214=PRODUCT_DEFINITION ( 'UNKNOWN', '', #1249, #3623 ) ;
#2217=CARTESIAN_POINT ( 'NONE',  ( 8.385254915620285132, 53.02855864072483882, 16.77050983124058092 ) ) ;
#2218=CARTESIAN_POINT ( 'NONE',  ( -10.00000000000000533, 92.00000000000000000, 4.500000000000000888 ) ) ;
#2221=CARTESIAN_POINT ( 'NONE',  ( -12.99553232110413958, 11.07475474455194053, -1.630606568990249473E-15 ) ) ;
#2222=VERTEX_POINT ( 'NONE', #10806 ) ;
#2223=EDGE_CURVE ( 'NONE', #10278, #7425, #10526, .T. ) ;
#2224=AXIS2_PLACEMENT_3D ( 'NONE', #4585, #12096, #7737 ) ;
#2226=EDGE_CURVE ( 'NONE', #297, #5518, #12965, .T. ) ;
#2229=VERTEX_POINT ( 'NONE', #1424 ) ;
#2236=DIRECTION ( 'NONE',  ( -2.797435172181481150E-17, 1.000000000000000000, -1.765856845898762549E-18 ) ) ;
#2238=DIRECTION ( 'NONE',  ( -1.000000000000000000, -0.000000000000000000, 0.000000000000000000 ) ) ;
#2239=AXIS2_PLACEMENT_3D ( 'NONE', #8754, #7697, #11909 ) ;
#2240=CARTESIAN_POINT ( 'NONE',  ( -3.789659181785903552, -84.41043748841794070, 8.773495529534001136 ) ) ;
#2243=VECTOR ( 'NONE', #6352, 1000.000000000000000 ) ;
#2245=ORIENTED_EDGE ( 'NONE', *, *, #12955, .F. ) ;
#2251=DIRECTION ( 'NONE',  ( -2.797435172181481150E-17, 1.000000000000000000, -1.765856845898762549E-18 ) ) ;
#2252=CARTESIAN_POINT ( 'NONE',  ( 12.99553232110413958, 58.19864449459908684, -25.99106464220826851 ) ) ;
#2254=CIRCLE ( 'NONE', #8525, 8.385254915620294014 ) ;
#2255=CARTESIAN_POINT ( 'NONE',  ( -10.69346802281034847, 2.474956373702985157, -1.318312975903535027E-15 ) ) ;
#2258=CARTESIAN_POINT ( 'NONE',  ( -9.736331930512843513, -69.99978782402621391, -2.722951059031194276 ) ) ;
#2259=CARTESIAN_POINT ( 'NONE',  ( -8.152362820468885829, -73.18181818181821541, -5.943141306424241321 ) ) ;
#2261=DIRECTION ( 'NONE',  ( -1.000000000000000000, 0.000000000000000000, 0.000000000000000000 ) ) ;
#2263=( BOUNDED_SURFACE ( )  B_SPLINE_SURFACE ( 3, 3, ( 
 ( #11952, #58, #1438, #2343 ),
 ( #6626, #12099, #10890, #1297 ),
 ( #5563, #9853, #4513, #2413 ),
 ( #5643, #13183, #9925, #3528 ) ),
 .UNSPECIFIED., .F., .F., .F. ) 
 B_SPLINE_SURFACE_WITH_KNOTS ( ( 4, 4 ),
 ( 4, 4 ),
 ( 0.000000000000000000, 1.000000000000000000 ),
 ( 0.000000000000000000, 1.000000000000000000 ),
 .UNSPECIFIED. ) 
 GEOMETRIC_REPRESENTATION_ITEM ( )  RATIONAL_B_SPLINE_SURFACE ( (
 ( 1.000000000000000000, 0.3333333333333334259, 0.3333333333333334259, 1.000000000000000000),
 ( 1.000000000000000000, 0.3333333333333334259, 0.3333333333333334259, 1.000000000000000000),
 ( 1.000000000000000000, 0.3333333333333334259, 0.3333333333333334259, 1.000000000000000000),
 ( 1.000000000000000000, 0.3333333333333334259, 0.3333333333333334259, 1.000000000000000000) ) ) 
 REPRESENTATION_ITEM ( '' )  SURFACE ( )  );
#2265=CARTESIAN_POINT ( 'NONE',  ( -39.99999999999999289, 120.0000000000000284, -0.5000000000000000000 ) ) ;
#2266=PLANE ( 'NONE',  #6271 ) ;
#2274=CARTESIAN_POINT ( 'NONE',  ( 15.29705854078139105, 55.48535772202409078, 1.773704474924341131E-15 ) ) ;
#2282=CARTESIAN_POINT ( 'NONE',  ( 34.00000000000001421, 108.0000000000000142, 2.500000000000000000 ) ) ;
#2287=CARTESIAN_POINT ( 'NONE',  ( -8.385254915620292238, 62.45333659073423860, -1.102836519679677113E-16 ) ) ;
#2288=CARTESIAN_POINT ( 'NONE',  ( -15.29705854078138749, 17.78624592198638155, -3.140796412417860432E-17 ) ) ;
#2289=AXIS2_PLACEMENT_3D ( 'NONE', #8458, #2078, #12747 ) ;
#2292=ORIENTED_EDGE ( 'NONE', *, *, #5390, .T. ) ;
#2293=ORIENTED_EDGE ( 'NONE', *, *, #368, .F. ) ;
#2296=ORIENTED_EDGE ( 'NONE', *, *, #7999, .T. ) ;
#2297=CARTESIAN_POINT ( 'NONE',  ( 15.29705854078138572, 66.79670324143890525, 1.757061666260240493E-15 ) ) ;
#2301=CARTESIAN_POINT ( 'NONE',  ( -15.29705854078138927, 66.79670324143890525, -3.866317875498727004E-15 ) ) ;
#2302=ADVANCED_FACE ( 'NONE', ( #4424 ), #243, .T. ) ;
#2303=CARTESIAN_POINT ( 'NONE',  ( 0.2804847452500967009, -81.23845599192084421, 9.920157271374822727 ) ) ;
#2315=DIRECTION ( 'NONE',  ( -1.000000000000000000, -0.000000000000000000, -0.000000000000000000 ) ) ;
#2323=CARTESIAN_POINT ( 'NONE',  ( 10.69346802281034847, -16.37459952631584059, 2.619144277183853555E-15 ) ) ;
#2326=ORIENTED_EDGE ( 'NONE', *, *, #99, .T. ) ;
#2327=EDGE_CURVE ( 'NONE', #10377, #430, #12102, .T. ) ;
#2328=CARTESIAN_POINT ( 'NONE',  ( 15.29705854078139282, 74.33491362204294717, 1.740418857596141631E-15 ) ) ;
#2330=TOROIDAL_SURFACE ( 'NONE', #3683, 48.00000000000001421, 2.000000000000000000 ) ;
#2332=CARTESIAN_POINT ( 'NONE',  ( -3.554095123023855901E-16, 12.70483462268159869, -2.243491919447391838E-17 ) ) ;
#2334=AXIS2_PLACEMENT_3D ( 'NONE', #3455, #2405, #1432 ) ;
#2340=CARTESIAN_POINT ( 'NONE',  ( 10.69381717166375445, 34.98422482212468054, 0.000000000000000000 ) ) ;
#2341=CARTESIAN_POINT ( 'NONE',  ( 12.99579180576516890, 26.38439787695498495, 1.549288279656779528E-15 ) ) ;
#2343=CARTESIAN_POINT ( 'NONE',  ( 15.29705854078140348, -29.33764382806072746, 3.746698755667525567E-15 ) ) ;
#2344=DIRECTION ( 'NONE',  ( -2.797435172181481150E-17, 1.000000000000000000, -1.765856845898762549E-18 ) ) ;
#2348=VERTEX_POINT ( 'NONE', #6917 ) ;
#2354=CARTESIAN_POINT ( 'NONE',  ( -8.385254915620294014, 24.75422479069652582, -4.371241731156832241E-17 ) ) ;
#2355=CARTESIAN_POINT ( 'NONE',  ( -10.69346802281034670, 40.17406817374066463, -1.451455445216333422E-15 ) ) ;
#2357=AXIS2_PLACEMENT_3D ( 'NONE', #5848, #5697, #8020 ) ;
#2359=CARTESIAN_POINT ( 'NONE',  ( -8.385254915620294014, 12.70483462268159869, -1.071767397633848135E-15 ) ) ;
#2364=DIRECTION ( 'NONE',  ( 1.000000000000000000, -0.000000000000000000, 0.000000000000000000 ) ) ;
#2366=CARTESIAN_POINT ( 'NONE',  ( -15.29705854078139815, 74.33491362204296138, 30.59411708156277854 ) ) ;
#2369=CARTESIAN_POINT ( 'NONE',  ( -15.29705854078139282, -8.601520358636511432, 1.518905361043589440E-17 ) ) ;
#2370=CARTESIAN_POINT ( 'NONE',  ( -0.1460947463170765848, -81.55043853261756226, 9.868234360004247918 ) ) ;
#2372=ORIENTED_EDGE ( 'NONE', *, *, #1041, .T. ) ;
#2375=VECTOR ( 'NONE', #4322, 1000.000000000000000 ) ;
#2379=EDGE_CURVE ( 'NONE', #6129, #6854, #11433, .T. ) ;
#2383=CARTESIAN_POINT ( 'NONE',  ( 15.29705854078138394, 36.63580182200524149, 30.59411708156277854 ) ) ;
#2386=DIRECTION ( 'NONE',  ( -2.797435172181481150E-17, 1.000000000000000000, -1.765856845898762549E-18 ) ) ;
#2387=ADVANCED_FACE ( 'NONE', ( #693 ), #10580, .T. ) ;
#2388=CARTESIAN_POINT ( 'NONE',  ( 0.5095487862222187747, -163.8787879204104456, 3.239446891907019399 ) ) ;
#2389=CARTESIAN_POINT ( 'NONE',  ( 1.485233070515279641, -81.00000000000027001, -9.907277990170701543 ) ) ;
#2391=DIRECTION ( 'NONE',  ( -2.797435172181481150E-17, 1.000000000000000000, -1.765856845898762549E-18 ) ) ;
#2393=ORIENTED_EDGE ( 'NONE', *, *, #13566, .T. ) ;
#2403=CARTESIAN_POINT ( 'NONE',  ( -0.1852016367016632581, -70.00000000000000000, 1.488522876466137790 ) ) ;
#2404=ORIENTED_EDGE ( 'NONE', *, *, #11143, .T. ) ;
#2405=DIRECTION ( 'NONE',  ( -2.797435172181481150E-17, 1.000000000000000000, -1.765856845898762549E-18 ) ) ;
#2406=CARTESIAN_POINT ( 'NONE',  ( 12.99553232110413781, 1.649976794542512337, 25.99106464220828627 ) ) ;
#2407=CARTESIAN_POINT ( 'NONE',  ( -12.99579180576516002, 45.23395377697383424, -25.99158361153033070 ) ) ;
#2410=EDGE_CURVE ( 'NONE', #5381, #1478, #3818, .T. ) ;
#2411=DIRECTION ( 'NONE',  ( -2.797435172181481150E-17, 1.000000000000000000, -1.765856845898762549E-18 ) ) ;
#2413=CARTESIAN_POINT ( 'NONE',  ( 10.69381717166376333, -30.98922082794128130, 2.619229793989005134E-15 ) ) ;
#2415=DIRECTION ( 'NONE',  ( -2.797435172181481150E-17, 1.000000000000000000, -1.765856845898762549E-18 ) ) ;
#2416=CARTESIAN_POINT ( 'NONE',  ( 10.69381717166374912, 16.13466892210585257, 21.38763434332750890 ) ) ;
#2417=ORIENTED_EDGE ( 'NONE', *, *, #10047, .T. ) ;
#2418=VERTEX_POINT ( 'NONE', #10360 ) ;
#2420=EDGE_CURVE ( 'NONE', #6795, #3901, #11215, .T. ) ;
#2422=CARTESIAN_POINT ( 'NONE',  ( 40.00000000000000711, 100.0000000000000000, -0.5000000000000000000 ) ) ;
#2424=( BOUNDED_SURFACE ( )  B_SPLINE_SURFACE ( 3, 3, ( 
 ( #2274, #4374, #8654, #4435 ),
 ( #12953, #3320, #6557, #10815 ),
 ( #12462, #6990, #11126, #3611 ),
 ( #1512, #10279, #10215, #13481 ) ),
 .UNSPECIFIED., .F., .F., .T. ) 
 B_SPLINE_SURFACE_WITH_KNOTS ( ( 4, 4 ),
 ( 4, 4 ),
 ( 0.000000000000000000, 1.000000000000000000 ),
 ( 0.000000000000000000, 1.000000000000000000 ),
 .UNSPECIFIED. ) 
 GEOMETRIC_REPRESENTATION_ITEM ( )  RATIONAL_B_SPLINE_SURFACE ( (
 ( 1.000000000000000000, 0.3333333333333334259, 0.3333333333333334259, 1.000000000000000000),
 ( 1.000000000000000000, 0.3333333333333334259, 0.3333333333333334259, 1.000000000000000000),
 ( 1.000000000000000000, 0.3333333333333334259, 0.3333333333333334259, 1.000000000000000000),
 ( 1.000000000000000000, 0.3333333333333334259, 0.3333333333333334259, 1.000000000000000000) ) ) 
 REPRESENTATION_ITEM ( '' )  SURFACE ( )  );
#2426=ADVANCED_FACE ( 'NONE', ( #4107 ), #2711, .T. ) ;
#2428=DIRECTION ( 'NONE',  ( 1.000000000000000000, 3.558407130208836623E-15, 0.000000000000000000 ) ) ;
#2430=CARTESIAN_POINT ( 'NONE',  ( -14.13596196814457429, -39.17949320881311337, -1.592785305112443692E-15 ) ) ;
#2434=CARTESIAN_POINT ( 'NONE',  ( -15.29705854078138927, 66.79670324143890525, -1.179534157023628988E-16 ) ) ;
#2438=DIRECTION ( 'NONE',  ( -2.797435172181481150E-17, 1.000000000000000000, -1.765856845898762549E-18 ) ) ;
#2439=ORIENTED_EDGE ( 'NONE', *, *, #7534, .F. ) ;
#2442=DIRECTION ( 'NONE',  ( -1.000000000000000000, 0.000000000000000000, 0.000000000000000000 ) ) ;
#2443=CARTESIAN_POINT ( 'NONE',  ( -15.29705854078139282, 36.63580182200523438, -6.469358145237827718E-17 ) ) ;
#2444=FACE_OUTER_BOUND ( 'NONE', #1135, .T. ) ;
#2446=CARTESIAN_POINT ( 'NONE',  ( 12.99579180576517601, -30.16426982310158067, 1.682131806534656762E-15 ) ) ;
#2449=CIRCLE ( 'NONE', #1555, 24.99999999999998934 ) ;
#2454=VERTEX_POINT ( 'NONE', #12616 ) ;
#2462=AXIS2_PLACEMENT_3D ( 'NONE', #7430, #7633, #6581 ) ;
#2463=CARTESIAN_POINT ( 'NONE',  ( 5.272971512688771512, -111.2727272727264136, -4.182478603667378891 ) ) ;
#2465=CARTESIAN_POINT ( 'NONE',  ( -15.29705854078138927, -18.02629830864593785, -30.59411708156278564 ) ) ;
#2466=DIRECTION ( 'NONE',  ( -1.000000000000000000, 0.000000000000000000, 0.000000000000000000 ) ) ;
#2472=ORIENTED_EDGE ( 'NONE', *, *, #9583, .T. ) ;
#2473=DIRECTION ( 'NONE',  ( 0.000000000000000000, 0.000000000000000000, 1.000000000000000000 ) ) ;
#2474=CARTESIAN_POINT ( 'NONE',  ( -32.72727272727271952, 135.1423002281142089, 2.500000000000000000 ) ) ;
#2479=DIRECTION ( 'NONE',  ( -2.797435172181481150E-17, 1.000000000000000000, -1.765856845898762549E-18 ) ) ;
#2480=VERTEX_POINT ( 'NONE', #7264 ) ;
#2486=DIRECTION ( 'NONE',  ( -1.000000000000000000, 0.000000000000000000, 0.000000000000000000 ) ) ;
#2489=FACE_OUTER_BOUND ( 'NONE', #3296, .T. ) ;
#2491=CARTESIAN_POINT ( 'NONE',  ( -2.517691654963332357E-15, 90.00000000000000000, -1.589271161308885878E-16 ) ) ;
#2500=ORIENTED_EDGE ( 'NONE', *, *, #9043, .F. ) ;
#2503=ADVANCED_FACE ( 'NONE', ( #9512 ), #4042, .T. ) ;
#2504=VERTEX_POINT ( 'NONE', #6289 ) ;
#2507=CARTESIAN_POINT ( 'NONE',  ( 15.29705854078138927, 55.48535772202409078, 1.773704474924340737E-15 ) ) ;
#2509=FACE_OUTER_BOUND ( 'NONE', #7236, .T. ) ;
#2511=CARTESIAN_POINT ( 'NONE',  ( 10.04421448860481370, -71.03329039087918773, 1.233851556784668180 ) ) ;
#2512=EDGE_LOOP ( 'NONE', ( #7083, #10952, #13546, #7362 ) ) ;
#2516=EDGE_CURVE ( 'NONE', #10661, #7842, #3578, .T. ) ;
#2517=CARTESIAN_POINT ( 'NONE',  ( -12.99553232110414491, -26.62435705548577047, -3.153769166990986831E-15 ) ) ;
#2527=VECTOR ( 'NONE', #12897, 1000.000000000000000 ) ;
#2528=EDGE_CURVE ( 'NONE', #10214, #5183, #8455, .T. ) ;
#2529=VERTEX_POINT ( 'NONE', #10622 ) ;
#2530=B_SPLINE_CURVE_WITH_KNOTS ( 'NONE', 3,
 ( #10089, #2430, #10161, #424 ),
 .UNSPECIFIED., .F., .F.,
 ( 4, 4 ),
 ( 0.000000000000000000, 1.000000000000000000 ),
 .UNSPECIFIED. ) ;
#2532=CARTESIAN_POINT ( 'NONE',  ( 5.312266725920431476, -76.81818181818330515, 8.563072071057876045 ) ) ;
#2534=CARTESIAN_POINT ( 'NONE',  ( 4.658052367537127481, 90.49197326372723182, 1.819943918220761514 ) ) ;
#2535=( LENGTH_UNIT ( ) NAMED_UNIT ( * ) SI_UNIT ( .MILLI., .METRE. ) );
#2536=DIRECTION ( 'NONE',  ( 0.000000000000000000, 0.000000000000000000, 1.000000000000000000 ) ) ;
#2537=CARTESIAN_POINT ( 'NONE',  ( 15.29705854078139460, -18.02629830864596627, 1.906846944237139921E-15 ) ) ;
#2541=CARTESIAN_POINT ( 'NONE',  ( 7.616846500228380279, -85.78354978356603056, -7.024694013235112777 ) ) ;
#2546=ORIENTED_EDGE ( 'NONE', *, *, #3616, .F. ) ;
#2548=CARTESIAN_POINT ( 'NONE',  ( -0.09498690616969264477, -159.7394095615612173, 1.519620673727829052 ) ) ;
#2551=DIRECTION ( 'NONE',  ( -2.797435172181481150E-17, 1.000000000000000000, -1.765856845898762549E-18 ) ) ;
#2554=B_SPLINE_CURVE_WITH_KNOTS ( 'NONE', 3,
 ( #386, #1212, #11013, #13226 ),
 .UNSPECIFIED., .F., .F.,
 ( 4, 4 ),
 ( 0.000000000000000000, 1.000000000000000000 ),
 .UNSPECIFIED. ) ;
#2555=DIRECTION ( 'NONE',  ( 0.000000000000000000, 0.000000000000000000, 1.000000000000000000 ) ) ;
#2562=CARTESIAN_POINT ( 'NONE',  ( 10.69381717166375445, 16.13466892210585613, 0.000000000000000000 ) ) ;
#2563=AXIS2_PLACEMENT_3D ( 'NONE', #9602, #6777, #3400 ) ;
#2567=CARTESIAN_POINT ( 'NONE',  ( -5.503342039658565452E-16, 19.67281349139174296, -3.473937238186366113E-17 ) ) ;
#2578=DIRECTION ( 'NONE',  ( -1.000000000000000000, 0.000000000000000000, 0.000000000000000000 ) ) ;
#2579=CARTESIAN_POINT ( 'NONE',  ( -15.29705854078138927, 57.37192529142945574, -1.013106070382630377E-16 ) ) ;
#2583=CARTESIAN_POINT ( 'NONE',  ( -15.29705854078139105, -38.76242177807012723, -1.736451602112920500E-15 ) ) ;
#2585=EDGE_LOOP ( 'NONE', ( #3562, #9665, #9197, #7304 ) ) ;
#2587=ORIENTED_EDGE ( 'NONE', *, *, #10621, .F. ) ;
#2588=CARTESIAN_POINT ( 'NONE',  ( 15.29705854078139815, -27.45107625865536960, -30.59411708156277854 ) ) ;
#2589=CIRCLE ( 'NONE', #5962, 79.99999999999997158 ) ;
#2596=CARTESIAN_POINT ( 'NONE',  ( -10.00000000000000000, 92.00000000000000000, -2.500000000000000000 ) ) ;
#2597=EDGE_CURVE ( 'NONE', #2835, #10317, #7263, .T. ) ;
#2599=EDGE_CURVE ( 'NONE', #3638, #13463, #409, .T. ) ;
#2601=CARTESIAN_POINT ( 'NONE',  ( -1.581702400640785156, -80.31021565580134336, -9.984810461684977767 ) ) ;
#2602=CARTESIAN_POINT ( 'NONE',  ( -10.69346802281034670, 59.02362407375952102, -1.518026679872732817E-15 ) ) ;
#2604=ORIENTED_EDGE ( 'NONE', *, *, #7546, .F. ) ;
#2607=CARTESIAN_POINT ( 'NONE',  ( 8.385254915620295790, -24.99427717735608212, 2.053795118489800793E-15 ) ) ;
#2608=CARTESIAN_POINT ( 'NONE',  ( 9.849330193486522944, -69.00000000000002842, 1.830547125266435149 ) ) ;
#2610=CARTESIAN_POINT ( 'NONE',  ( -0.3899449583696082411, -79.59552047185403012, 10.11716208309628762 ) ) ;
#2614=CARTESIAN_POINT ( 'NONE',  ( -10.69346802281034492, 11.89973432371241380, -1.351598593231734330E-15 ) ) ;
#2615=CARTESIAN_POINT ( 'NONE',  ( 0.05222919907312795901, -79.03030303025963121, -10.66847369585458516 ) ) ;
#2616=EDGE_CURVE ( 'NONE', #6810, #8462, #13314, .T. ) ;
#2617=CARTESIAN_POINT ( 'NONE',  ( -10.00000000000000000, 90.00000000000000000, 2.500000000000000000 ) ) ;
#2621=VERTEX_POINT ( 'NONE', #3257 ) ;
#2625=CARTESIAN_POINT ( 'NONE',  ( 2.607973140908031784, -104.0364159275374760, -6.664989919102580984 ) ) ;
#2626=CARTESIAN_POINT ( 'NONE',  ( -15.29705854078138927, 29.09759144140119957, -5.138218104596347907E-17 ) ) ;
#2627=DIRECTION ( 'NONE',  ( -2.797435172181481150E-17, 1.000000000000000000, -1.765856845898762549E-18 ) ) ;
#2630=DIRECTION ( 'NONE',  ( -1.000000000000000000, 0.000000000000000000, 0.000000000000000000 ) ) ;
#2632=CARTESIAN_POINT ( 'NONE',  ( -0.5090839304981049640, -157.9207379528257604, -1.416845878072839460 ) ) ;
#2637=CARTESIAN_POINT ( 'NONE',  ( 12.99553232110414491, -7.774801155466914970, 0.000000000000000000 ) ) ;
#2638=ORIENTED_EDGE ( 'NONE', *, *, #6959, .T. ) ;
#2639=DIRECTION ( 'NONE',  ( -2.797435172181481150E-17, 1.000000000000000000, -1.765856845898762549E-18 ) ) ;
#2642=CARTESIAN_POINT ( 'NONE',  ( 2.920448137081741891, -118.2727272727312595, 4.227847206581237138 ) ) ;
#2646=CARTESIAN_POINT ( 'NONE',  ( 5.849706340539694516, -65.63636363268138041, 2.546235460329709710 ) ) ;
#2647=CARTESIAN_POINT ( 'NONE',  ( -10.69381717166375800, 6.709890972096425266, 21.38763434332750890 ) ) ;
#2648=CARTESIAN_POINT ( 'NONE',  ( -15.29705854078140348, -19.91286587805129926, 30.59411708156278564 ) ) ;
#2649=CARTESIAN_POINT ( 'NONE',  ( 10.69346802281034847, -35.22415542633469698, 2.619144277183853555E-15 ) ) ;
#2650=CARTESIAN_POINT ( 'NONE',  ( 14.13596196814457606, -39.17949320881311337, 3.462312115431394170E-15 ) ) ;
#2654=CIRCLE ( 'NONE', #2189, 2.000000000000003997 ) ;
#2655=ORIENTED_EDGE ( 'NONE', *, *, #3503, .T. ) ;
#2660=AXIS2_PLACEMENT_3D ( 'NONE', #10823, #191, #1299 ) ;
#2661=DIRECTION ( 'NONE',  ( -2.797435172181481150E-17, 1.000000000000000000, -1.765856845898762549E-18 ) ) ;
#2664=CARTESIAN_POINT ( 'NONE',  ( 2.866591608029287919, -101.4961736542552160, 6.904028388510872638 ) ) ;
#2665=CARTESIAN_POINT ( 'NONE',  ( -10.69381717166376156, -30.98922082794128130, -2.584341753958642254E-15 ) ) ;
#2667=ADVANCED_FACE ( 'NONE', ( #11950 ), #5426, .T. ) ;
#2668=ORIENTED_EDGE ( 'NONE', *, *, #9951, .F. ) ;
#2669=EDGE_CURVE ( 'NONE', #13011, #3550, #2926, .T. ) ;
#2674=ORIENTED_EDGE ( 'NONE', *, *, #1830, .T. ) ;
#2677=ORIENTED_EDGE ( 'NONE', *, *, #1191, .F. ) ;
#2678=CARTESIAN_POINT ( 'NONE',  ( -15.29705854078139637, 64.91013567203349055, -1.146220074446778111E-16 ) ) ;
#2681=CARTESIAN_POINT ( 'NONE',  ( 5.770059030975414061, -111.2727272727274510, -3.008649887262795808 ) ) ;
#2682=CARTESIAN_POINT ( 'NONE',  ( -10.69381717166375800, 44.40900277213413716, 21.38763434332750535 ) ) ;
#2683=CARTESIAN_POINT ( 'NONE',  ( 9.846850911383061344, -91.60173160173981444, -0.3733502116074404742 ) ) ;
#2686=LINE ( 'NONE', #4717, #6238 ) ;
#2689=ORIENTED_EDGE ( 'NONE', *, *, #8985, .T. ) ;
#2691=EDGE_CURVE ( 'NONE', #1421, #1176, #5843, .T. ) ;
#2693=EDGE_LOOP ( 'NONE', ( #13345, #7689, #6148, #5706 ) ) ;
#2694=CARTESIAN_POINT ( 'NONE',  ( -2.021131906156611535, -99.55200189714852854, -7.478639190186810559 ) ) ;
#2696=CARTESIAN_POINT ( 'NONE',  ( 8.385254915620294014, 12.70483462268159869, 1.002145295323929345E-15 ) ) ;
#2697=EDGE_CURVE ( 'NONE', #2418, #3001, #247, .T. ) ;
#2699=CIRCLE ( 'NONE', #4462, 15.29705854078138927 ) ;
#2703=CARTESIAN_POINT ( 'NONE',  ( 3.598469168196945844, -133.8876842431320142, 0.1837403886752023985 ) ) ;
#2704=AXIS2_PLACEMENT_3D ( 'NONE', #5719, #8878, #7816 ) ;
#2705=VECTOR ( 'NONE', #7761, 1000.000000000000000 ) ;
#2706=CARTESIAN_POINT ( 'NONE',  ( 4.895553837162434974, 90.06565955263931755, -1.025098571782897983 ) ) ;
#2708=DIRECTION ( 'NONE',  ( -1.000000000000000000, -5.171946152600902986E-17, 0.000000000000000000 ) ) ;
#2709=CARTESIAN_POINT ( 'NONE',  ( -0.1852016367018560761, -70.00000000000000000, 1.488522876466114253 ) ) ;
#2710=CARTESIAN_POINT ( 'NONE',  ( -12.99579180576517246, 64.08350967699263379, -1.817850092276246042E-15 ) ) ;
#2711=TOROIDAL_SURFACE ( 'NONE', #695, 42.00000000000001421, 2.000000000000000000 ) ;
#2713=CARTESIAN_POINT ( 'NONE',  ( 4.330127018922190096, 91.83037361138187293, 2.500000000000000000 ) ) ;
#2714=ORIENTED_EDGE ( 'NONE', *, *, #9894, .F. ) ;
#2715=CARTESIAN_POINT ( 'NONE',  ( -3.042673274263591132, -100.2727272727296537, -12.70187379131512628 ) ) ;
#2716=VERTEX_POINT ( 'NONE', #476 ) ;
#2719=AXIS2_PLACEMENT_3D ( 'NONE', #11729, #2058, #12667 ) ;
#2720=CARTESIAN_POINT ( 'NONE',  ( 3.056920711447597139, -140.5584415584316957, 3.800163123442064528 ) ) ;
#2721=AXIS2_PLACEMENT_3D ( 'NONE', #3215, #9884, #286 ) ;
#2723=DIRECTION ( 'NONE',  ( -2.797435172181481150E-17, 1.000000000000000000, -1.765856845898762549E-18 ) ) ;
#2724=CARTESIAN_POINT ( 'NONE',  ( 12.99579180576517423, -20.73949187309215247, 3.183050967463144168E-15 ) ) ;
#2725=CARTESIAN_POINT ( 'NONE',  ( 12.99553232110413425, -36.04913500549519512, 25.99106464220827917 ) ) ;
#2726=CARTESIAN_POINT ( 'NONE',  ( 8.235865160261019113, -74.54711633044367147, 5.866162657818820847 ) ) ;
#2727=B_SPLINE_CURVE_WITH_KNOTS ( 'NONE', 3,
 ( #8863, #8943, #7731, #10812 ),
 .UNSPECIFIED., .F., .F.,
 ( 4, 4 ),
 ( 0.000000000000000000, 1.000000000000000000 ),
 .UNSPECIFIED. ) ;
#2730=( BOUNDED_SURFACE ( )  B_SPLINE_SURFACE ( 3, 3, ( 
 ( #7377, #11386, #11597, #13808 ),
 ( #13743, #3891, #4088, #5082 ),
 ( #1780, #4158, #1989, #9364 ),
 ( #6270, #8440, #12729, #2840 ) ),
 .UNSPECIFIED., .F., .F., .F. ) 
 B_SPLINE_SURFACE_WITH_KNOTS ( ( 4, 4 ),
 ( 4, 4 ),
 ( 0.000000000000000000, 1.000000000000000000 ),
 ( 0.000000000000000000, 1.000000000000000000 ),
 .UNSPECIFIED. ) 
 GEOMETRIC_REPRESENTATION_ITEM ( )  RATIONAL_B_SPLINE_SURFACE ( (
 ( 1.000000000000000000, 0.3333333333333334259, 0.3333333333333334259, 1.000000000000000000),
 ( 1.000000000000000000, 0.3333333333333334259, 0.3333333333333334259, 1.000000000000000000),
 ( 1.000000000000000000, 0.3333333333333334259, 0.3333333333333334259, 1.000000000000000000),
 ( 1.000000000000000000, 0.3333333333333334259, 0.3333333333333334259, 1.000000000000000000) ) ) 
 REPRESENTATION_ITEM ( '' )  SURFACE ( )  );
#2731=AXIS2_PLACEMENT_3D ( 'NONE', #7513, #9360, #1008 ) ;
#2732=B_SPLINE_CURVE_WITH_KNOTS ( 'NONE', 3,
 ( #7890, #6841, #1363, #13180 ),
 .UNSPECIFIED., .F., .F.,
 ( 4, 4 ),
 ( 0.000000000000000000, 1.000000000000000000 ),
 .UNSPECIFIED. ) ;
#2733=CARTESIAN_POINT ( 'NONE',  ( 15.29705854078139637, -27.45107625865536605, 1.949638918210572832E-15 ) ) ;
#2735=ORIENTED_EDGE ( 'NONE', *, *, #2597, .F. ) ;
#2736=CARTESIAN_POINT ( 'NONE',  ( 8.385254915620301119, -34.41905512736551032, -16.77050983124059158 ) ) ;
#2740=DIRECTION ( 'NONE',  ( -1.000000000000000000, 0.000000000000000000, 0.000000000000000000 ) ) ;
#2741=CARTESIAN_POINT ( 'NONE',  ( 5.802558726164779301, -86.30923214627286200, -7.334200378339981619 ) ) ;
#2742=CARTESIAN_POINT ( 'NONE',  ( 10.69346802281033781, 59.02362407375952102, 21.38693604562068984 ) ) ;
#2743=VERTEX_POINT ( 'NONE', #6982 ) ;
#2744=VERTEX_POINT ( 'NONE', #1655 ) ;
#2746=CARTESIAN_POINT ( 'NONE',  ( 2.197875741315407971, -79.21212121212158763, 9.798460318839140371 ) ) ;
#2748=CARTESIAN_POINT ( 'NONE',  ( 9.243399941159408328, -71.03723844962674150, 4.118320456981444444 ) ) ;
#2750=CARTESIAN_POINT ( 'NONE',  ( 2.264596963715684641, -106.9090909090917449, -6.916633125700833773 ) ) ;
#2751=CARTESIAN_POINT ( 'NONE',  ( -10.00000000000000711, 139.9999999999999716, 0.5000000000000000000 ) ) ;
#2753=CARTESIAN_POINT ( 'NONE',  ( 1.024176664970867456, -142.5800865801970758, 2.358741788133955186 ) ) ;
#2757=CARTESIAN_POINT ( 'NONE',  ( -15.29705854078139282, 36.63580182200523438, -6.469358145237827718E-17 ) ) ;
#2758=ADVANCED_FACE ( 'NONE', ( #8171 ), #1924, .T. ) ;
#2759=AXIS2_PLACEMENT_3D ( 'NONE', #2567, #8875, #6844 ) ;
#2760=( LENGTH_UNIT ( ) NAMED_UNIT ( * ) SI_UNIT ( .MILLI., .METRE. ) );
#2761=EDGE_CURVE ( 'NONE', #6483, #7762, #11124, .T. ) ;
#2763=EDGE_LOOP ( 'NONE', ( #2604, #4999, #10793, #5861, #7324, #5018, #13356, #5893, #11172, #9843 ) ) ;
#2767=CARTESIAN_POINT ( 'NONE',  ( -3.600965394138023523, -133.8702908180223119, -0.1741706324120513294 ) ) ;
#2774=CARTESIAN_POINT ( 'NONE',  ( 3.636509701354637691, -131.0710334046880234, -1.453205936098713735 ) ) ;
#2775=DIRECTION ( 'NONE',  ( 2.797435172181480534E-17, -1.000000000000000000, 1.765856845898762164E-18 ) ) ;
#2776=CYLINDRICAL_SURFACE ( 'NONE', #10301, 15.29705854078138927 ) ;
#2777=CARTESIAN_POINT ( 'NONE',  ( -4.974937185533102380, 90.00000000000000000, -0.5000000000000000000 ) ) ;
#2778=AXIS2_PLACEMENT_3D ( 'NONE', #11087, #11300, #653 ) ;
#2779=DIRECTION ( 'NONE',  ( -0.000000000000000000, -0.000000000000000000, -1.000000000000000000 ) ) ;
#2783=CARTESIAN_POINT ( 'NONE',  ( -2.237684797877294057E-15, 79.99058638175036151, -1.412519245696701404E-16 ) ) ;
#2788=AXIS2_PLACEMENT_3D ( 'NONE', #1447, #3468, #4754 ) ;
#2789=DIRECTION ( 'NONE',  ( -1.000000000000000000, 0.000000000000000000, 0.000000000000000000 ) ) ;
#2791=EDGE_CURVE ( 'NONE', #13463, #6241, #1801, .T. ) ;
#2792=CARTESIAN_POINT ( 'NONE',  ( -4.208314830420946784, -157.8181818182383438, -0.6624707635850120013 ) ) ;
#2796=LINE ( 'NONE', #633, #4094 ) ;
#2799=VERTEX_POINT ( 'NONE', #527 ) ;
#2800=DIRECTION ( 'NONE',  ( 0.000000000000000000, 0.000000000000000000, 1.000000000000000000 ) ) ;
#2802=CARTESIAN_POINT ( 'NONE',  ( -12.99579180576517246, -20.73949187309215247, -3.174617675444691075E-15 ) ) ;
#2805=CARTESIAN_POINT ( 'NONE',  ( 12.99579180576516713, -1.889935973073297859, 1.604750804297411238E-15 ) ) ;
#2807=CARTESIAN_POINT ( 'NONE',  ( -5.569711040290264314, -116.8635738538862654, -0.6440865148614328684 ) ) ;
#2808=CARTESIAN_POINT ( 'NONE',  ( 12.99553232110412893, 58.19864449459908684, 25.99106464220827561 ) ) ;
#2809=( BOUNDED_SURFACE ( )  B_SPLINE_SURFACE ( 3, 3, ( 
 ( #11225, #1615, #5900, #10173 ),
 ( #584, #4847, #13438, #5972 ),
 ( #1956, #10444, #8341, #11426 ),
 ( #980, #12635, #4060, #3075 ) ),
 .UNSPECIFIED., .F., .F., .T. ) 
 B_SPLINE_SURFACE_WITH_KNOTS ( ( 4, 4 ),
 ( 4, 4 ),
 ( 0.000000000000000000, 1.000000000000000000 ),
 ( 0.000000000000000000, 1.000000000000000000 ),
 .UNSPECIFIED. ) 
 GEOMETRIC_REPRESENTATION_ITEM ( )  RATIONAL_B_SPLINE_SURFACE ( (
 ( 1.000000000000000000, 0.3333333333333334259, 0.3333333333333334259, 1.000000000000000000),
 ( 1.000000000000000000, 0.3333333333333334259, 0.3333333333333334259, 1.000000000000000000),
 ( 1.000000000000000000, 0.3333333333333334259, 0.3333333333333334259, 1.000000000000000000),
 ( 1.000000000000000000, 0.3333333333333334259, 0.3333333333333334259, 1.000000000000000000) ) ) 
 REPRESENTATION_ITEM ( '' )  SURFACE ( )  );
#2811=CIRCLE ( 'NONE', #585, 14.99999999999999112 ) ;
#2814=CARTESIAN_POINT ( 'NONE',  ( -12.99553232110414491, -26.62435705548577047, -1.497464099677451275E-15 ) ) ;
#2815=CARTESIAN_POINT ( 'NONE',  ( 3.711366765502052356, -78.09090909090807031, 9.373274001092589458 ) ) ;
#2816=EDGE_LOOP ( 'NONE', ( #2293, #4955, #8610, #1789 ) ) ;
#2817=CARTESIAN_POINT ( 'NONE',  ( 3.108119077941494446, -77.10324909055569265, 9.630131019297053285 ) ) ;
#2818=DIRECTION ( 'NONE',  ( 0.000000000000000000, 0.000000000000000000, 1.000000000000000000 ) ) ;
#2819=AXIS2_PLACEMENT_3D ( 'NONE', #4004, #11369, #5988 ) ;
#2820=CARTESIAN_POINT ( 'NONE',  ( -5.272971512688663154, -111.2727272727274368, 4.182478603667165729 ) ) ;
#2821=CYLINDRICAL_SURFACE ( 'NONE', #4150, 8.385254915620292238 ) ;
#2822=CARTESIAN_POINT ( 'NONE',  ( -12.99553232110414314, 20.49953269456136695, -1.663892186318449368E-15 ) ) ;
#2823=CARTESIAN_POINT ( 'NONE',  ( 0.1852016367012860043, -160.0000000000003126, -1.488522876466233713 ) ) ;
#2824=CIRCLE ( 'NONE', #1934, 15.29705854078139105 ) ;
#2825=VERTEX_POINT ( 'NONE', #9976 ) ;
#2826=ADVANCED_FACE ( 'NONE', ( #1485 ), #9577, .T. ) ;
#2828=CARTESIAN_POINT ( 'NONE',  ( 1.787228567177412186, -149.6910924273273906, -0.8766906025594750629 ) ) ;
#2831=CARTESIAN_POINT ( 'NONE',  ( -3.430185293861314655, -134.8221474816296563, -0.6797513324038796378 ) ) ;
#2834=DIRECTION ( 'NONE',  ( -2.797435172181481150E-17, 1.000000000000000000, -1.765856845898762549E-18 ) ) ;
#2835=VERTEX_POINT ( 'NONE', #6952 ) ;
#2839=CARTESIAN_POINT ( 'NONE',  ( -39.99999999999999289, 120.0000000000000284, 0.5000000000000000000 ) ) ;
#2840=CARTESIAN_POINT ( 'NONE',  ( -15.29705854078139637, 0.8232575913729158756, -3.749818214850030626E-15 ) ) ;
#2842=FACE_OUTER_BOUND ( 'NONE', #8879, .T. ) ;
#2846=CARTESIAN_POINT ( 'NONE',  ( 5.138450363093609141, -111.7272727272695079, -0.006098328147151244397 ) ) ;
#2849=EDGE_CURVE ( 'NONE', #2083, #6241, #9947, .T. ) ;
#2853=CARTESIAN_POINT ( 'NONE',  ( -10.00000000000000711, 97.99999999999994316, 0.5000000000000000000 ) ) ;
#2854=DIRECTION ( 'NONE',  ( -2.797435172181481150E-17, 1.000000000000000000, -1.765856845898762549E-18 ) ) ;
#2856=DIRECTION ( 'NONE',  ( 1.000000000000000000, 0.000000000000000000, 0.000000000000000000 ) ) ;
#2861=B_SPLINE_CURVE_WITH_KNOTS ( 'NONE', 3,
 ( #8559, #3295, #11853, #11921, #10725, #7774, #8626, #5611, #300, #6660, #9683, #8835, #10857, #1267, #11786, #5534 ),
 .UNSPECIFIED., .F., .F.,
 ( 4, 2, 2, 2, 2, 2, 2, 4 ),
 ( 0.000000000000000000, 0.0009977135201011855421, 0.001496570280151775494, 0.001995427040202365446, 0.002494283800252954965, 0.002993140560303544917, 0.003491997320354134869, 0.003990854080404723954 ),
 .UNSPECIFIED. ) ;
#2863=EDGE_CURVE ( 'NONE', #8344, #8462, #10568, .T. ) ;
#2864=CARTESIAN_POINT ( 'NONE',  ( -0.9875499244693202172, -80.00464164737402939, 10.06307371418729701 ) ) ;
#2866=TOROIDAL_SURFACE ( 'NONE', #5317, 22.99999999999999289, 2.000000000000000000 ) ;
#2867=ORIENTED_EDGE ( 'NONE', *, *, #3795, .T. ) ;
#2868=CARTESIAN_POINT ( 'NONE',  ( 15.29705854078139460, -10.48808792804187284, -30.59411708156277854 ) ) ;
#2869=CARTESIAN_POINT ( 'NONE',  ( 8.385254915620297567, 31.55439052270045508, -16.77050983124059158 ) ) ;
#2873=CARTESIAN_POINT ( 'NONE',  ( 8.470699010985018873, -93.30712875542430140, 0.4970230768060718840 ) ) ;
#2878=ORIENTED_EDGE ( 'NONE', *, *, #2223, .F. ) ;
#2882=CARTESIAN_POINT ( 'NONE',  ( -15.29705854078139105, -38.76242177807012723, -3.676584163678260711E-15 ) ) ;
#2884=CARTESIAN_POINT ( 'NONE',  ( 8.385254915620292238, 90.00000000000000000, 8.679704431140118580E-16 ) ) ;
#2886=AXIS2_PLACEMENT_3D ( 'NONE', #8842, #4857, #11240 ) ;
#2890=CARTESIAN_POINT ( 'NONE',  ( 15.29705854078139105, 19.67281349139174296, 1.840275709580740132E-15 ) ) ;
#2892=CARTESIAN_POINT ( 'NONE',  ( -1.053348594425001616, -150.0300328178547318, -1.640268818953221963 ) ) ;
#2896=ORIENTED_EDGE ( 'NONE', *, *, #701, .T. ) ;
#2899=DIRECTION ( 'NONE',  ( -2.797435172181481150E-17, 1.000000000000000000, -1.765856845898762549E-18 ) ) ;
#2902=CARTESIAN_POINT ( 'NONE',  ( -1.207220731154811100, -146.6502848478751275, 1.905708617823901108 ) ) ;
#2904=CARTESIAN_POINT ( 'NONE',  ( -1.111302930823951263, -163.8787879467685116, -2.940232647904911012 ) ) ;
#2905=CYLINDRICAL_SURFACE ( 'NONE', #9655, 8.385254915620294014 ) ;
#2906=CARTESIAN_POINT ( 'NONE',  ( 0.000000000000000000, 71.01020514433645303, -0.5000000000000000000 ) ) ;
#2909=AXIS2_PLACEMENT_3D ( 'NONE', #4225, #8240, #13749 ) ;
#2910=DIRECTION ( 'NONE',  ( 1.000000000000000000, 0.000000000000000000, 0.000000000000000000 ) ) ;
#2911=CARTESIAN_POINT ( 'NONE',  ( -8.385254915620297567, 31.55439052270045508, -1.138338632290247530E-15 ) ) ;
#2916=CARTESIAN_POINT ( 'NONE',  ( 4.560784247219194398, -95.36363636362298735, 0.7586904865634463979 ) ) ;
#2918=EDGE_LOOP ( 'NONE', ( #10221, #4399 ) ) ;
#2923=CARTESIAN_POINT ( 'NONE',  ( 4.588105241694418801, -161.0909090907375401, -0.3432044964428315192 ) ) ;
#2924=EDGE_CURVE ( 'NONE', #10679, #7969, #9284, .T. ) ;
#2926=B_SPLINE_CURVE_WITH_KNOTS ( 'NONE', 3,
 ( #13027, #125, #7599, #1295 ),
 .UNSPECIFIED., .F., .F.,
 ( 4, 4 ),
 ( 0.000000000000000000, 1.000000000000000000 ),
 .UNSPECIFIED. ) ;
#2928=CARTESIAN_POINT ( 'NONE',  ( 12.99553232110413958, 48.77386654458962312, 3.182987412051232168E-15 ) ) ;
#2931=AXIS2_PLACEMENT_3D ( 'NONE', #7129, #11405, #6089 ) ;
#2932=CARTESIAN_POINT ( 'NONE',  ( -10.69381717166375623, 16.13466892210585613, -1.366597928139322991E-15 ) ) ;
#2933=VECTOR ( 'NONE', #11026, 1000.000000000000000 ) ;
#2934=CARTESIAN_POINT ( 'NONE',  ( -4.658064847839354705, 90.49194140877688142, 1.819915145876240370 ) ) ;
#2935=EDGE_CURVE ( 'NONE', #10108, #10478, #5401, .T. ) ;
#2936=EDGE_CURVE ( 'NONE', #13011, #11197, #6215, .T. ) ;
#2939=CARTESIAN_POINT ( 'NONE',  ( -5.035065420445773654, -83.15251865640357209, 8.244702687588977952 ) ) ;
#2940=ORIENTED_EDGE ( 'NONE', *, *, #1122, .F. ) ;
#2941=ORIENTED_EDGE ( 'NONE', *, *, #984, .T. ) ;
#2942=CARTESIAN_POINT ( 'NONE',  ( -8.385254915620292238, -22.36966495935058319, -2.016610837207367011E-15 ) ) ;
#2943=B_SPLINE_CURVE_WITH_KNOTS ( 'NONE', 3,
 ( #13250, #1650, #10269, #3674, #3522, #7959, #6979, #5866, #6761, #10138, #547, #11323, #2706, #611, #12094, #4809 ),
 .UNSPECIFIED., .F., .F.,
 ( 4, 2, 2, 2, 2, 2, 2, 4 ),
 ( 0.000000000000000000, 0.0003997740159331187953, 0.0007995480318662375905, 0.001599096063732475181, 0.001998870079665579936, 0.002398644095598684474, 0.002798418111531789012, 0.003198192127464893550 ),
 .UNSPECIFIED. ) ;
#2946=CARTESIAN_POINT ( 'NONE',  ( -15.29705854078138749, -1.063309978032445979, -30.59411708156277854 ) ) ;
#2947=CARTESIAN_POINT ( 'NONE',  ( 2.958050194273104783, -139.3718435583852227, -0.4183503205596436625 ) ) ;
#2948=CARTESIAN_POINT ( 'NONE',  ( 8.385254915620290461, 79.99058638175036151, 8.868043070384787486E-16 ) ) ;
#2950=EDGE_CURVE ( 'NONE', #4148, #5091, #12833, .T. ) ;
#2952=EDGE_LOOP ( 'NONE', ( #2668, #7333, #9668, #861 ) ) ;
#2957=CARTESIAN_POINT ( 'NONE',  ( 12.97449437267217753, -39.59556244224027211, 1.645560741966129631E-15 ) ) ;
#2958=VERTEX_POINT ( 'NONE', #3109 ) ;
#2959=CARTESIAN_POINT ( 'NONE',  ( 15.29705854078138927, 90.00000000000000000, 1.714422261702872766E-15 ) ) ;
#2960=AXIS2_PLACEMENT_3D ( 'NONE', #7185, #1856, #6274 ) ;
#2962=CARTESIAN_POINT ( 'NONE',  ( -5.912741552701379355, -73.45454545179654815, -18.82838426746663174 ) ) ;
#2964=B_SPLINE_CURVE_WITH_KNOTS ( 'NONE', 3,
 ( #1496, #5776, #8434, #13738, #7171, #5075, #11922, #11854, #10859, #229 ),
 .UNSPECIFIED., .F., .F.,
 ( 4, 3, 3, 4 ),
 ( 0.000000000000000000, 0.0007726433382168586489, 0.001886030654550297121, 0.002999417971186700387 ),
 .UNSPECIFIED. ) ;
#2965=CARTESIAN_POINT ( 'NONE',  ( 5.478016874438395689, -117.3626624613967806, 1.011505465123966552 ) ) ;
#2967=EDGE_CURVE ( 'NONE', #6908, #6441, #13285, .T. ) ;
#2969=VERTEX_POINT ( 'NONE', #1995 ) ;
#2971=DIRECTION ( 'NONE',  ( -1.000000000000000000, 0.000000000000000000, 0.000000000000000000 ) ) ;
#2973=CARTESIAN_POINT ( 'NONE',  ( 5.059189827636713765, -83.15590270883112112, -8.262539084012589186 ) ) ;
#2974=CARTESIAN_POINT ( 'NONE',  ( -0.5850150888136983474, -160.9696969704900482, 1.917718896956037700 ) ) ;
#2978=CARTESIAN_POINT ( 'NONE',  ( -15.29705854078139282, 90.00000000000000000, -1.589271161308885878E-16 ) ) ;
#2980=AXIS2_PLACEMENT_3D ( 'NONE', #7985, #5731, #4680 ) ;
#2982=CARTESIAN_POINT ( 'NONE',  ( 12.66071438417660922, -140.5584415584655460, 5.506376209459975080 ) ) ;
#2987=CARTESIAN_POINT ( 'NONE',  ( -4.330127018922201643, 91.72908881866754882, -2.499999999999993783 ) ) ;
#2990=AXIS2_PLACEMENT_3D ( 'NONE', #4490, #1331, #13298 ) ;
#2991=CARTESIAN_POINT ( 'NONE',  ( -3.361332843921210234, -147.1038961038632067, -14.17852599539660297 ) ) ;
#2992=CARTESIAN_POINT ( 'NONE',  ( -10.00000000000000711, 139.9999999999999716, -0.5000000000000000000 ) ) ;
#2993=CARTESIAN_POINT ( 'NONE',  ( 15.29705854078139105, -36.87585420866476227, 3.746698755667522411E-15 ) ) ;
#2994=CARTESIAN_POINT ( 'NONE',  ( -4.338055960494663132, 91.73205429892865936, 2.486400748338238653 ) ) ;
#2995=ORIENTED_EDGE ( 'NONE', *, *, #12917, .F. ) ;
#2997=EDGE_CURVE ( 'NONE', #1745, #13042, #1170, .T. ) ;
#2998=CARTESIAN_POINT ( 'NONE',  ( -8.844020276311006512, -89.05663101222295097, 1.691421750721286088 ) ) ;
#2999=EDGE_CURVE ( 'NONE', #8545, #3001, #11535, .T. ) ;
#3001=VERTEX_POINT ( 'NONE', #5146 ) ;
#3006=CARTESIAN_POINT ( 'NONE',  ( -15.29705854078138927, 57.37192529142945574, -1.013106070382630377E-16 ) ) ;
#3007=CARTESIAN_POINT ( 'NONE',  ( 2.997639754412456892, -137.4006169092532161, -1.171341992379282715 ) ) ;
#3012=CYLINDRICAL_SURFACE ( 'NONE', #8089, 15.29705854078139105 ) ;
#3013=ORIENTED_EDGE ( 'NONE', *, *, #10866, .T. ) ;
#3016=CIRCLE ( 'NONE', #10832, 79.99999999999997158 ) ;
#3017=VERTEX_POINT ( 'NONE', #9501 ) ;
#3018=CARTESIAN_POINT ( 'NONE',  ( -2.504624958784990426E-13, 92.00000000000000000, -4.500000000000000888 ) ) ;
#3022=EDGE_LOOP ( 'NONE', ( #7971, #2587, #11100, #11127 ) ) ;
#3024=CARTESIAN_POINT ( 'NONE',  ( -10.00000000000000000, 90.00000000000000000, 0.5000000000000000000 ) ) ;
#3026=CARTESIAN_POINT ( 'NONE',  ( -8.597717047221227205, -85.78354978359179484, 6.129448613111333266 ) ) ;
#3027=FACE_BOUND ( 'NONE', #9859, .T. ) ;
#3030=CARTESIAN_POINT ( 'NONE',  ( -2.416244575755594148, -133.5561241431034887, 2.746148655430789454 ) ) ;
#3032=TOROIDAL_SURFACE ( 'NONE', #13591, 16.99999999999998934, 2.000000000000000000 ) ;
#3033=EDGE_LOOP ( 'NONE', ( #3076, #9189, #13236, #8479 ) ) ;
#3036=ORIENTED_EDGE ( 'NONE', *, *, #2936, .F. ) ;
#3037=CARTESIAN_POINT ( 'NONE',  ( -0.3297608091563175581, -142.6355133186271757, -2.624337192179055478 ) ) ;
#3041=CARTESIAN_POINT ( 'NONE',  ( 6.326212770466429269, -95.26718119391159689, 5.262869407572682512 ) ) ;
#3043=CARTESIAN_POINT ( 'NONE',  ( 8.385254915620290461, 62.45333659073424570, -16.77050983124057737 ) ) ;
#3047=CARTESIAN_POINT ( 'NONE',  ( 10.00000000000000711, 139.9999999999999716, -2.500000000000000000 ) ) ;
#3048=CARTESIAN_POINT ( 'NONE',  ( 15.29705854078139282, -1.063309978032472403, 1.873561326908939435E-15 ) ) ;
#3049=AXIS2_PLACEMENT_3D ( 'NONE', #1748, #10373, #9184 ) ;
#3050=EDGE_LOOP ( 'NONE', ( #13784, #4749, #5332, #9024 ) ) ;
#3054=ORIENTED_EDGE ( 'NONE', *, *, #7896, .T. ) ;
#3057=DIRECTION ( 'NONE',  ( -2.797435172181481150E-17, 1.000000000000000000, -1.765856845898762549E-18 ) ) ;
#3059=CARTESIAN_POINT ( 'NONE',  ( 0.003226301100676102433, -100.2727272727208856, 4.613888802083836893 ) ) ;
#3060=B_SPLINE_CURVE_WITH_KNOTS ( 'NONE', 3,
 ( #13331, #3681, #12249, #6905 ),
 .UNSPECIFIED., .F., .F.,
 ( 4, 4 ),
 ( 0.000000000000000000, 1.000000000000000000 ),
 .UNSPECIFIED. ) ;
#3062=CARTESIAN_POINT ( 'NONE',  ( 8.385254915620292238, -22.36966495935058319, 2.053795118489800004E-15 ) ) ;
#3064=DIRECTION ( 'NONE',  ( 1.000000000000000000, 0.000000000000000000, 0.000000000000000000 ) ) ;
#3065=AXIS2_PLACEMENT_3D ( 'NONE', #6709, #9799, #7545 ) ;
#3068=CARTESIAN_POINT ( 'NONE',  ( -12.99579180576516890, -11.31471392308272605, -3.182109625360474349E-15 ) ) ;
#3071=CARTESIAN_POINT ( 'NONE',  ( -15.29705854078139460, 55.48535772202409078, -2.069307775394917278E-15 ) ) ;
#3072=CARTESIAN_POINT ( 'NONE',  ( 15.29705854078139460, -1.063309978032445091, -30.59411708156277854 ) ) ;
#3073=DIRECTION ( 'NONE',  ( -2.797435172181481150E-17, 1.000000000000000000, -1.765856845898762549E-18 ) ) ;
#3075=CARTESIAN_POINT ( 'NONE',  ( -15.29705854078139282, 47.94714734142005597, -3.833032258170527700E-15 ) ) ;
#3076=ORIENTED_EDGE ( 'NONE', *, *, #8071, .F. ) ;
#3079=CARTESIAN_POINT ( 'NONE',  ( -2.517691654963332357E-15, 90.00000000000000000, -1.589271161308885878E-16 ) ) ;
#3084=CARTESIAN_POINT ( 'NONE',  ( -6.213657885899291244, -97.41991341993369247, -5.968417174478657827 ) ) ;
#3085=DIRECTION ( 'NONE',  ( 0.000000000000000000, 0.000000000000000000, 1.000000000000000000 ) ) ;
#3087=CARTESIAN_POINT ( 'NONE',  ( -0.6173387890061908800, -69.99999999999998579, 4.961742921553712549 ) ) ;
#3089=CARTESIAN_POINT ( 'NONE',  ( 8.385254915620292238, 69.25350232273815720, 9.631531405059307235E-16 ) ) ;
#3091=CARTESIAN_POINT ( 'NONE',  ( 5.650019569485428050, -113.2088557674236000, -2.224334737347880786 ) ) ;
#3101=CARTESIAN_POINT ( 'NONE',  ( 7.692922818056756817, -86.09451208659135091, -5.376924148044465390 ) ) ;
#3106=DIRECTION ( 'NONE',  ( -1.000000000000000000, 0.000000000000000000, 0.000000000000000000 ) ) ;
#3107=CARTESIAN_POINT ( 'NONE',  ( 10.69346802281034670, 30.74929022373126841, 2.619144277183853555E-15 ) ) ;
#3109=CARTESIAN_POINT ( 'NONE',  ( 15.29705854078139282, -38.76242177807012723, 1.940132561565339224E-15 ) ) ;
#3110=EDGE_CURVE ( 'NONE', #1805, #3210, #5856, .T. ) ;
#3112=CARTESIAN_POINT ( 'NONE',  ( -12.09338464843076189, -169.0000000000000568, 0.006909782850911748778 ) ) ;
#3114=CARTESIAN_POINT ( 'NONE',  ( -2.517691654963332357E-15, 90.00000000000000000, -1.589271161308885878E-16 ) ) ;
#3116=CARTESIAN_POINT ( 'NONE',  ( 12.99579180576516890, -11.31471392308272605, 0.000000000000000000 ) ) ;
#3118=CARTESIAN_POINT ( 'NONE',  ( 1.174765158563475076, -79.03030302990762834, 10.44010582255705444 ) ) ;
#3119=CARTESIAN_POINT ( 'NONE',  ( -2.886819890957894152, -105.1818181818214839, 3.599275682873828153 ) ) ;
#3121=CARTESIAN_POINT ( 'NONE',  ( 8.385254915620294014, 50.40394642271930792, 2.053795118489800793E-15 ) ) ;
#3122=CARTESIAN_POINT ( 'NONE',  ( 15.29705854078139105, -36.87585420866476227, 1.940132561565339224E-15 ) ) ;
#3123=CARTESIAN_POINT ( 'NONE',  ( -12.99579180576516535, 16.95961992694555676, -1.651422005635246569E-15 ) ) ;
#3124=AXIS2_PLACEMENT_3D ( 'NONE', #13005, #2185, #2466 ) ;
#3125=ADVANCED_FACE ( 'NONE', ( #4266 ), #4196, .T. ) ;
#3126=AXIS2_PLACEMENT_3D ( 'NONE', #13264, #2639, #8112 ) ;
#3130=CARTESIAN_POINT ( 'NONE',  ( -8.385254915620292238, 53.02855864072483882, -9.364084330386787485E-17 ) ) ;
#3132=AXIS2_PLACEMENT_3D ( 'NONE', #5561, #4511, #6691 ) ;
#3133=AXIS2_PLACEMENT_3D ( 'NONE', #1126, #2364, #5382 ) ;
#3135=DIRECTION ( 'NONE',  ( 1.000000000000000000, 2.797435172181480534E-17, -0.000000000000000000 ) ) ;
#3136=CYLINDRICAL_SURFACE ( 'NONE', #9483, 8.385254915620292238 ) ;
#3137=DIRECTION ( 'NONE',  ( 1.000000000000000000, -0.000000000000000000, 0.000000000000000000 ) ) ;
#3139=CIRCLE ( 'NONE', #7183, 2.000000000000003109 ) ;
#3141=EDGE_CURVE ( 'NONE', #30, #11958, #4961, .T. ) ;
#3142=CARTESIAN_POINT ( 'NONE',  ( -15.29705854078139105, -10.48808792804187284, 1.852046186812095429E-17 ) ) ;
#3143=CARTESIAN_POINT ( 'NONE',  ( 15.29705854078138749, 76.22148119144830503, 1.740418857596141236E-15 ) ) ;
#3146=AXIS2_PLACEMENT_3D ( 'NONE', #7655, #7583, #2261 ) ;
#3148=DIRECTION ( 'NONE',  ( -0.8907235428302473501, 0.4545454545454531425, 0.000000000000000000 ) ) ;
#3154=CARTESIAN_POINT ( 'NONE',  ( -0.8598734018918594568, -151.0707854172325426, -1.652135397942386064 ) ) ;
#3161=EDGE_CURVE ( 'NONE', #1460, #10921, #2254, .T. ) ;
#3166=CARTESIAN_POINT ( 'NONE',  ( 7.846342596345671438, -93.17560321804917578, 3.276283083350423730 ) ) ;
#3167=CARTESIAN_POINT ( 'NONE',  ( -15.29705854078138927, -8.601520358636511432, -30.59411708156278564 ) ) ;
#3168=CYLINDRICAL_SURFACE ( 'NONE', #2731, 8.385254915620292238 ) ;
#3169=CARTESIAN_POINT ( 'NONE',  ( -2.008006351130390499, -80.00378950643924725, -9.910921267331605833 ) ) ;
#3170=ADVANCED_FACE ( 'NONE', ( #7630 ), #9607, .T. ) ;
#3171=CARTESIAN_POINT ( 'NONE',  ( -8.385254915620290461, 22.12961257269105531, -16.77050983124058803 ) ) ;
#3173=CARTESIAN_POINT ( 'NONE',  ( 0.2899689842974736975, -80.99999999999971578, -10.01379011345939851 ) ) ;
#3174=DIRECTION ( 'NONE',  ( 0.000000000000000000, 0.000000000000000000, 1.000000000000000000 ) ) ;
#3175=CARTESIAN_POINT ( 'NONE',  ( -12.99553232110414491, 29.92431064457076673, 25.99106464220827917 ) ) ;
#3178=CARTESIAN_POINT ( 'NONE',  ( 15.29705854078139460, 74.33491362204296138, -30.59411708156277854 ) ) ;
#3179=ORIENTED_EDGE ( 'NONE', *, *, #8308, .F. ) ;
#3183=FACE_OUTER_BOUND ( 'NONE', #10497, .T. ) ;
#3186=DIRECTION ( 'NONE',  ( 1.000000000000000000, 0.000000000000000000, 0.000000000000000000 ) ) ;
#3188=CARTESIAN_POINT ( 'NONE',  ( 8.355983819232738696, -73.45454545667848834, 17.50953411836414730 ) ) ;
#3189=EDGE_CURVE ( 'NONE', #12042, #8931, #4052, .T. ) ;
#3190=CARTESIAN_POINT ( 'NONE',  ( 4.980291965142508381, -118.2727272727225056, 1.265069668247140955 ) ) ;
#3192=CARTESIAN_POINT ( 'NONE',  ( -12.99553232110413958, 11.07475474455194053, -3.208141528222677273E-15 ) ) ;
#3193=DIRECTION ( 'NONE',  ( 1.000000000000000000, 0.000000000000000000, 0.000000000000000000 ) ) ;
#3194=DIRECTION ( 'NONE',  ( -1.000000000000000000, 0.000000000000000000, 0.000000000000000000 ) ) ;
#3197=ORIENTED_EDGE ( 'NONE', *, *, #3710, .T. ) ;
#3200=EDGE_LOOP ( 'NONE', ( #7220, #6516, #4931, #8490 ) ) ;
#3201=FACE_OUTER_BOUND ( 'NONE', #8209, .T. ) ;
#3204=LINE ( 'NONE', #1307, #2375 ) ;
#3205=CARTESIAN_POINT ( 'NONE',  ( -6.266477149339306330, -76.69310177716063492, -7.966230677900265178 ) ) ;
#3210=VERTEX_POINT ( 'NONE', #2297 ) ;
#3212=ORIENTED_EDGE ( 'NONE', *, *, #6988, .F. ) ;
#3215=CARTESIAN_POINT ( 'NONE',  ( 1.958204620527036102E-15, -69.99999999999998579, 1.236099792129133461E-16 ) ) ;
#3216=VECTOR ( 'NONE', #3790, 1000.000000000000000 ) ;
#3217=( BOUNDED_SURFACE ( )  B_SPLINE_SURFACE ( 3, 3, ( 
 ( #13837, #7274, #10369, #9251 ),
 ( #10500, #1950, #5038, #2802 ),
 ( #13565, #3919, #9321, #12627 ),
 ( #8265, #12558, #7207, #2942 ) ),
 .UNSPECIFIED., .F., .F., .F. ) 
 B_SPLINE_SURFACE_WITH_KNOTS ( ( 4, 4 ),
 ( 4, 4 ),
 ( 0.000000000000000000, 1.000000000000000000 ),
 ( 0.000000000000000000, 1.000000000000000000 ),
 .UNSPECIFIED. ) 
 GEOMETRIC_REPRESENTATION_ITEM ( )  RATIONAL_B_SPLINE_SURFACE ( (
 ( 1.000000000000000000, 0.3333333333333334259, 0.3333333333333334259, 1.000000000000000000),
 ( 1.000000000000000000, 0.3333333333333334259, 0.3333333333333334259, 1.000000000000000000),
 ( 1.000000000000000000, 0.3333333333333334259, 0.3333333333333334259, 1.000000000000000000),
 ( 1.000000000000000000, 0.3333333333333334259, 0.3333333333333334259, 1.000000000000000000) ) ) 
 REPRESENTATION_ITEM ( '' )  SURFACE ( )  );
#3220=CARTESIAN_POINT ( 'NONE',  ( 15.29705854078138572, 66.79670324143890525, 1.757061666260240493E-15 ) ) ;
#3221=CARTESIAN_POINT ( 'NONE',  ( -7.706471693472447981, -95.44282728834829754, -2.820513248663373496 ) ) ;
#3222=CARTESIAN_POINT ( 'NONE',  ( 25.00000000000000355, 120.0000000000000284, 0.5000000000000000000 ) ) ;
#3223=ORIENTED_EDGE ( 'NONE', *, *, #10707, .F. ) ;
#3224=VECTOR ( 'NONE', #449, 1000.000000000000000 ) ;
#3225=ORIENTED_EDGE ( 'NONE', *, *, #3340, .F. ) ;
#3230=FACE_OUTER_BOUND ( 'NONE', #2196, .T. ) ;
#3231=DIRECTION ( 'NONE',  ( 0.000000000000000000, 0.000000000000000000, 1.000000000000000000 ) ) ;
#3232=CARTESIAN_POINT ( 'NONE',  ( -3.339827705271122937, -118.5554015396263878, -4.233164074552941081 ) ) ;
#3233=CARTESIAN_POINT ( 'NONE',  ( -12.99579180576516002, 7.534841976936127672, -25.99158361153033070 ) ) ;
#3235=CIRCLE ( 'NONE', #11082, 42.00000000000001421 ) ;
#3236=CARTESIAN_POINT ( 'NONE',  ( 0.7701066202684784257, -168.0000000000001421, 1.909695209560601681 ) ) ;
#3237=CARTESIAN_POINT ( 'NONE',  ( -10.03938689678716045, -69.87878787879108700, -0.2267434780641402192 ) ) ;
#3239=TOROIDAL_SURFACE ( 'NONE', #350, 16.99999999999998934, 2.000000000000000000 ) ;
#3242=EDGE_CURVE ( 'NONE', #887, #7475, #6092, .T. ) ;
#3248=CARTESIAN_POINT ( 'NONE',  ( -1.024862805779478135E-15, 36.63580182200523438, -6.469358145237827718E-17 ) ) ;
#3253=VECTOR ( 'NONE', #12432, 1000.000000000000000 ) ;
#3254=CARTESIAN_POINT ( 'NONE',  ( -2.517691654963332357E-15, 90.00000000000000000, -1.589271161308885878E-16 ) ) ;
#3255=CARTESIAN_POINT ( 'NONE',  ( -12.99579180576517601, 26.38439787695498495, 25.99158361153033425 ) ) ;
#3256=LINE ( 'NONE', #7530, #8783 ) ;
#3257=CARTESIAN_POINT ( 'NONE',  ( 8.385254915620292238, -22.36966495935058319, 1.068716529980328346E-15 ) ) ;
#3258=CARTESIAN_POINT ( 'NONE',  ( 15.29705854078138927, 10.24803554138234318, -30.59411708156276788 ) ) ;
#3264=EDGE_CURVE ( 'NONE', #2504, #12042, #1531, .T. ) ;
#3265=AXIS2_PLACEMENT_3D ( 'NONE', #2105, #5604, #5394 ) ;
#3268=ADVANCED_FACE ( 'NONE', ( #3707 ), #9049, .T. ) ;
#3270=CIRCLE ( 'NONE', #7520, 8.385254915620290461 ) ;
#3274=CYLINDRICAL_SURFACE ( 'NONE', #6073, 2.000000000000001776 ) ;
#3282=ORIENTED_EDGE ( 'NONE', *, *, #2082, .F. ) ;
#3283=CYLINDRICAL_SURFACE ( 'NONE', #3133, 2.000000000000000000 ) ;
#3284=EDGE_LOOP ( 'NONE', ( #5814, #6647, #8077, #11520 ) ) ;
#3285=CARTESIAN_POINT ( 'NONE',  ( 12.99579180576516002, 73.50828762700210461, 25.99158361153033425 ) ) ;
#3288=LINE ( 'NONE', #9815, #12176 ) ;
#3289=CARTESIAN_POINT ( 'NONE',  ( -8.193545109616771072, -89.96337882711635814, 3.459978222445851515 ) ) ;
#3290=CARTESIAN_POINT ( 'NONE',  ( -10.00000000000000711, 92.00000000000000000, 0.5000000000000000000 ) ) ;
#3293=ORIENTED_EDGE ( 'NONE', *, *, #2935, .T. ) ;
#3294=( BOUNDED_SURFACE ( )  B_SPLINE_SURFACE ( 3, 3, ( 
 ( #3567, #5752, #8986, #9126 ),
 ( #1618, #8074, #13291, #13441 ),
 ( #3930, #12638, #9401, #12493 ),
 ( #11631, #10383, #5051, #10508 ) ),
 .UNSPECIFIED., .F., .F., .F. ) 
 B_SPLINE_SURFACE_WITH_KNOTS ( ( 4, 4 ),
 ( 4, 4 ),
 ( 0.000000000000000000, 1.000000000000000000 ),
 ( 0.000000000000000000, 1.000000000000000000 ),
 .UNSPECIFIED. ) 
 GEOMETRIC_REPRESENTATION_ITEM ( )  RATIONAL_B_SPLINE_SURFACE ( (
 ( 1.000000000000000000, 0.3333333333333334259, 0.3333333333333334259, 1.000000000000000000),
 ( 1.000000000000000000, 0.3333333333333334259, 0.3333333333333334259, 1.000000000000000000),
 ( 1.000000000000000000, 0.3333333333333334259, 0.3333333333333334259, 1.000000000000000000),
 ( 1.000000000000000000, 0.3333333333333334259, 0.3333333333333334259, 1.000000000000000000) ) ) 
 REPRESENTATION_ITEM ( '' )  SURFACE ( )  );
#3295=CARTESIAN_POINT ( 'NONE',  ( -2.482863863605453414, 89.99999999999998579, 4.353049703108321289 ) ) ;
#3296=EDGE_LOOP ( 'NONE', ( #1863, #5946, #10075 ) ) ;
#3297=DIRECTION ( 'NONE',  ( -0.5999999999999989786, -0.8000000000000008216, 0.000000000000000000 ) ) ;
#3298=CARTESIAN_POINT ( 'NONE',  ( 0.9875500501441598633, -80.00464164738322381, -10.06307372056550342 ) ) ;
#3299=CARTESIAN_POINT ( 'NONE',  ( -15.29705854078138394, 8.361467971976955127, -30.59411708156277854 ) ) ;
#3301=CARTESIAN_POINT ( 'NONE',  ( -0.04956920568762178403, -160.9696969682810561, 0.4964001826923840621 ) ) ;
#3302=CARTESIAN_POINT ( 'NONE',  ( -6.967039245478320098, -74.45454545454718698, -7.244513656184790484 ) ) ;
#3303=CARTESIAN_POINT ( 'NONE',  ( -35.45454545454546036, 140.4866414850956744, -0.5000000000000000000 ) ) ;
#3315=ORIENTED_EDGE ( 'NONE', *, *, #12528, .T. ) ;
#3319=AXIS2_PLACEMENT_3D ( 'NONE', #13898, #143, #7617 ) ;
#3320=CARTESIAN_POINT ( 'NONE',  ( 12.99579180576517068, 54.65873172698324112, -25.99158361153033070 ) ) ;
#3325=( BOUNDED_SURFACE ( )  B_SPLINE_SURFACE ( 3, 3, ( 
 ( #1522, #423, #4762, #9036 ),
 ( #13350, #3767, #6999, #2649 ),
 ( #11209, #12335, #2725, #11279 ),
 ( #1035, #10564, #10494, #2993 ) ),
 .UNSPECIFIED., .F., .F., .T. ) 
 B_SPLINE_SURFACE_WITH_KNOTS ( ( 4, 4 ),
 ( 4, 4 ),
 ( 0.000000000000000000, 1.000000000000000000 ),
 ( 0.000000000000000000, 1.000000000000000000 ),
 .UNSPECIFIED. ) 
 GEOMETRIC_REPRESENTATION_ITEM ( )  RATIONAL_B_SPLINE_SURFACE ( (
 ( 1.000000000000000000, 0.3333333333333334259, 0.3333333333333334259, 1.000000000000000000),
 ( 1.000000000000000000, 0.3333333333333334259, 0.3333333333333334259, 1.000000000000000000),
 ( 1.000000000000000000, 0.3333333333333334259, 0.3333333333333334259, 1.000000000000000000),
 ( 1.000000000000000000, 0.3333333333333334259, 0.3333333333333334259, 1.000000000000000000) ) ) 
 REPRESENTATION_ITEM ( '' )  SURFACE ( )  );
#3328=CARTESIAN_POINT ( 'NONE',  ( -12.99579180576517068, 16.95961992694555676, 25.99158361153032359 ) ) ;
#3330=ORIENTED_EDGE ( 'NONE', *, *, #11633, .F. ) ;
#3332=ADVANCED_FACE ( 'NONE', ( #8463 ), #1813, .T. ) ;
#3336=DIRECTION ( 'NONE',  ( -0.000000000000000000, -0.000000000000000000, -1.000000000000000000 ) ) ;
#3339=ADVANCED_FACE ( 'NONE', ( #6301 ), #6623, .T. ) ;
#3340=EDGE_CURVE ( 'NONE', #3968, #5518, #6513, .T. ) ;
#3343=CYLINDRICAL_SURFACE ( 'NONE', #3319, 8.385254915620292238 ) ;
#3344=ORIENTED_EDGE ( 'NONE', *, *, #8677, .T. ) ;
#3349=ORIENTED_EDGE ( 'NONE', *, *, #4817, .T. ) ;
#3350=CARTESIAN_POINT ( 'NONE',  ( -8.385254915620292238, 71.87811454074363837, 16.77050983124057382 ) ) ;
#3351=CARTESIAN_POINT ( 'NONE',  ( 25.00000000000000355, 120.0000000000000284, 2.500000000000000000 ) ) ;
#3353=ADVANCED_FACE ( 'NONE', ( #5238 ), #3217, .T. ) ;
#3355=CYLINDRICAL_SURFACE ( 'NONE', #1412, 8.385254915620295790 ) ;
#3359=ORIENTED_EDGE ( 'NONE', *, *, #5951, .F. ) ;
#3362=ORIENTED_EDGE ( 'NONE', *, *, #6959, .F. ) ;
#3367=LINE ( 'NONE', #11993, #313 ) ;
#3368=CARTESIAN_POINT ( 'NONE',  ( -15.29705854078139460, 36.63580182200524149, 30.59411708156277498 ) ) ;
#3371=CARTESIAN_POINT ( 'NONE',  ( -0.4692480219583425871, -80.00113634546181629, -9.989149782162604296 ) ) ;
#3372=CARTESIAN_POINT ( 'NONE',  ( -1.830305755785371247, -166.5454545179101444, -12.49768923203297000 ) ) ;
#3374=CARTESIAN_POINT ( 'NONE',  ( -0.1760972876107445573, -80.66666666666708352, -10.02690338805403059 ) ) ;
#3377=ORIENTED_EDGE ( 'NONE', *, *, #11978, .T. ) ;
#3378=AXIS2_PLACEMENT_3D ( 'NONE', #12095, #9997, #405 ) ;
#3381=DIRECTION ( 'NONE',  ( -1.000000000000000000, 0.000000000000000000, 0.000000000000000000 ) ) ;
#3382=DIRECTION ( 'NONE',  ( -2.797435172181481150E-17, 1.000000000000000000, -1.765856845898762549E-18 ) ) ;
#3383=ORIENTED_EDGE ( 'NONE', *, *, #11733, .T. ) ;
#3388=B_SPLINE_SURFACE_WITH_KNOTS ( 'NONE', 3, 3, ( 
 ( #12939, #3439, #7448, #6603, #9829, #10937, #9764, #13874, #173, #1155, #4219, #11728, #4498, #10868 ),
 ( #3173, #3374, #8776, #13087, #2118, #9563, #6406, #10673, #7581, #5281, #1083, #3237, #7516, #11864 ),
 ( #2389, #8574, #5542, #5345, #9631, #38, #4292, #3302, #2259, #12873, #1215, #11797, #6542, #2186 ),
 ( #6471, #10738, #5411, #9694, #102, #4418, #4354, #13007, #8638, #10800, #5479, #8702, #13691, #559 ) ),
 .UNSPECIFIED., .F., .F., .F.,
 ( 4, 4 ),
 ( 4, 1, 1, 1, 1, 1, 1, 1, 1, 1, 1, 4 ),
 ( -0.003299999999999999982, 0.0002999999999999999195 ),
 ( 0.07900000000000000078, 0.08000000000000000167, 0.08063636363636363102, 0.08172727272727271786, 0.08336363636363636198, 0.08445454545454544881, 0.08554545454545453564, 0.08663636363636362248, 0.08827272727272726660, 0.08936363636363635343, 0.08999999999999998279, 0.09099999999999998368 ),
 .UNSPECIFIED. ) ;
#3395=ADVANCED_FACE ( 'NONE', ( #10438 ), #839, .T. ) ;
#3396=DIRECTION ( 'NONE',  ( 1.000000000000000000, 0.000000000000000000, 0.000000000000000000 ) ) ;
#3400=DIRECTION ( 'NONE',  ( -1.000000000000000000, 0.000000000000000000, 0.000000000000000000 ) ) ;
#3402=CARTESIAN_POINT ( 'NONE',  ( -15.29705854078139105, 27.21102387199583816, -4.805077278827845308E-17 ) ) ;
#3404=AXIS2_PLACEMENT_3D ( 'NONE', #5505, #9789, #262 ) ;
#3406=CARTESIAN_POINT ( 'NONE',  ( 10.69346802281033959, 11.89973432371241202, 21.38693604562068984 ) ) ;
#3407=EDGE_LOOP ( 'NONE', ( #8138, #12920, #11329, #10765 ) ) ;
#3410=ADVANCED_FACE ( 'NONE', ( #1044 ), #6365, .T. ) ;
#3413=B_SPLINE_CURVE_WITH_KNOTS ( 'NONE', 3,
 ( #4985, #12573, #3933, #13847, #10318, #11436, #4129, #11634, #12769, #4191, #9261, #10387, #12706, #2031, #6114, #8475 ),
 .UNSPECIFIED., .F., .F.,
 ( 4, 2, 2, 2, 2, 2, 2, 4 ),
 ( 0.000000000000000000, 0.0005014865247272646664, 0.001002973049454529333, 0.001504459574181793999, 0.002005946098909058666, 0.002507432623636323549, 0.003008919148363587998, 0.004011892197818117331 ),
 .UNSPECIFIED. ) ;
#3414=CARTESIAN_POINT ( 'NONE',  ( 1.031578115675553693E-15, -36.87585420866476227, 6.511747960273540061E-17 ) ) ;
#3418=DIRECTION ( 'NONE',  ( -2.797435172181481150E-17, 1.000000000000000000, -1.765856845898762549E-18 ) ) ;
#3420=CARTESIAN_POINT ( 'NONE',  ( -0.2039587671352304787, -79.18543995220413478, -10.12004280472452322 ) ) ;
#3422=CARTESIAN_POINT ( 'NONE',  ( 39.99999999999999289, 120.0000000000000284, 0.5000000000000000000 ) ) ;
#3423=CARTESIAN_POINT ( 'NONE',  ( -2.627534660932791866, -83.45264110882523312, 9.274001503740121777 ) ) ;
#3426=ORIENTED_EDGE ( 'NONE', *, *, #1994, .T. ) ;
#3427=ADVANCED_FACE ( 'NONE', ( #3201 ), #7479, .T. ) ;
#3431=EDGE_CURVE ( 'NONE', #6129, #5860, #7415, .T. ) ;
#3434=CARTESIAN_POINT ( 'NONE',  ( 12.99579180576516002, -1.889935973073298081, 25.99158361153033070 ) ) ;
#3438=CARTESIAN_POINT ( 'NONE',  ( 0.9182679296299990357, -167.9999999999998863, 0.7188769083877146748 ) ) ;
#3439=CARTESIAN_POINT ( 'NONE',  ( -1.376272962219557749, -80.66666666666647245, -10.07778225401753147 ) ) ;
#3443=ORIENTED_EDGE ( 'NONE', *, *, #969, .T. ) ;
#3445=DIRECTION ( 'NONE',  ( -5.551115123125776539E-17, 1.000000000000000000, 3.204747427460360459E-31 ) ) ;
#3446=ORIENTED_EDGE ( 'NONE', *, *, #7911, .F. ) ;
#3448=ADVANCED_FACE ( 'NONE', ( #10696 ), #8062, .T. ) ;
#3449=DIRECTION ( 'NONE',  ( -2.797435172181481150E-17, 1.000000000000000000, -1.765856845898762549E-18 ) ) ;
#3451=ORIENTED_EDGE ( 'NONE', *, *, #6098, .T. ) ;
#3452=AXIS2_PLACEMENT_3D ( 'NONE', #4306, #6349, #4103 ) ;
#3454=EDGE_LOOP ( 'NONE', ( #9211, #12621, #11759, #7218 ) ) ;
#3455=CARTESIAN_POINT ( 'NONE',  ( 6.991987007918878033E-16, -24.99427717735608212, 4.413631546192547049E-17 ) ) ;
#3456=CARTESIAN_POINT ( 'NONE',  ( 48.00000000000000000, 120.0000000000000284, 0.5000000000000000000 ) ) ;
#3457=CARTESIAN_POINT ( 'NONE',  ( 10.69381717166375445, 44.40900277213413716, 1.251590067034001600E-15 ) ) ;
#3458=VECTOR ( 'NONE', #5220, 1000.000000000000000 ) ;
#3459=DIRECTION ( 'NONE',  ( 1.000000000000000000, 0.000000000000000000, 0.000000000000000000 ) ) ;
#3462=FACE_OUTER_BOUND ( 'NONE', #7527, .T. ) ;
#3465=AXIS2_PLACEMENT_3D ( 'NONE', #11722, #3231, #7510 ) ;
#3466=CIRCLE ( 'NONE', #5723, 42.00000000000001421 ) ;
#3467=ORIENTED_EDGE ( 'NONE', *, *, #11589, .F. ) ;
#3468=DIRECTION ( 'NONE',  ( -2.797435172181481150E-17, 1.000000000000000000, -1.765856845898762549E-18 ) ) ;
#3471=DIRECTION ( 'NONE',  ( -1.000000000000000000, 0.000000000000000000, 0.000000000000000000 ) ) ;
#3486=CARTESIAN_POINT ( 'NONE',  ( -12.99579180576517423, -30.16426982310158067, -3.167125725528906618E-15 ) ) ;
#3487=LINE ( 'NONE', #293, #10647 ) ;
#3489=VERTEX_POINT ( 'NONE', #4583 ) ;
#3492=DIRECTION ( 'NONE',  ( -2.797435172181481150E-17, 1.000000000000000000, -1.765856845898762549E-18 ) ) ;
#3496=CARTESIAN_POINT ( 'NONE',  ( 10.69346802281034314, 59.02362407375952102, 1.239914983259925247E-15 ) ) ;
#3497=EDGE_CURVE ( 'NONE', #12645, #1929, #5913, .T. ) ;
#3499=CARTESIAN_POINT ( 'NONE',  ( 5.390560935658633923, -117.0909090909101451, 3.329211565281263940 ) ) ;
#3501=CARTESIAN_POINT ( 'NONE',  ( -8.385254915620294014, -15.56949922734665570, -2.023984266965477934E-15 ) ) ;
#3503=EDGE_CURVE ( 'NONE', #7000, #5403, #1159, .T. ) ;
#3509=B_SPLINE_CURVE_WITH_KNOTS ( 'NONE', 3,
 ( #9457, #7202, #834, #897 ),
 .UNSPECIFIED., .F., .F.,
 ( 4, 4 ),
 ( 0.000000000000000000, 1.000000000000000000 ),
 .UNSPECIFIED. ) ;
#3510=ORIENTED_EDGE ( 'NONE', *, *, #3869, .F. ) ;
#3518=VERTEX_POINT ( 'NONE', #13540 ) ;
#3520=ORIENTED_EDGE ( 'NONE', *, *, #13836, .F. ) ;
#3522=CARTESIAN_POINT ( 'NONE',  ( 4.390129302555905610, 91.34360472797649777, -2.393760519723236779 ) ) ;
#3523=CARTESIAN_POINT ( 'NONE',  ( 10.69381717166375800, 44.40900277213413716, -21.38763434332750890 ) ) ;
#3528=CARTESIAN_POINT ( 'NONE',  ( 8.385254915620295790, -31.79444290936001138, 2.053795118489800793E-15 ) ) ;
#3530=ADVANCED_FACE ( 'NONE', ( #9150 ), #2905, .T. ) ;
#3532=FACE_OUTER_BOUND ( 'NONE', #1448, .T. ) ;
#3535=VERTEX_POINT ( 'NONE', #8105 ) ;
#3542=EDGE_CURVE ( 'NONE', #2048, #4278, #3821, .T. ) ;
#3544=AXIS2_PLACEMENT_3D ( 'NONE', #13497, #7987, #7755 ) ;
#3545=CARTESIAN_POINT ( 'NONE',  ( 3.164093758375789989, -79.18419793333841028, 9.628149030606312664 ) ) ;
#3547=EDGE_LOOP ( 'NONE', ( #13830, #688, #7566, #1189 ) ) ;
#3550=VERTEX_POINT ( 'NONE', #8233 ) ;
#3553=ORIENTED_EDGE ( 'NONE', *, *, #2516, .T. ) ;
#3561=AXIS2_PLACEMENT_3D ( 'NONE', #12803, #6404, #7245 ) ;
#3562=ORIENTED_EDGE ( 'NONE', *, *, #13243, .T. ) ;
#3563=ORIENTED_EDGE ( 'NONE', *, *, #7336, .F. ) ;
#3564=VECTOR ( 'NONE', #6964, 1000.000000000000000 ) ;
#3567=CARTESIAN_POINT ( 'NONE',  ( -8.385254915620297567, -6.144721277337256815, -1.005196162977448937E-15 ) ) ;
#3569=CARTESIAN_POINT ( 'NONE',  ( -1.485233070515140197, -80.99999999999981526, 9.907277990170733517 ) ) ;
#3572=CARTESIAN_POINT ( 'NONE',  ( -15.29705854078139105, 57.37192529142945574, -3.849675066834626958E-15 ) ) ;
#3576=CARTESIAN_POINT ( 'NONE',  ( 10.69346802281034847, -16.37459952631584059, 1.341678554766028988E-15 ) ) ;
#3577=CARTESIAN_POINT ( 'NONE',  ( 2.889799813501469306, -137.4545454544992822, 1.105612428329187047 ) ) ;
#3578=CIRCLE ( 'NONE', #12786, 16.99999999999998934 ) ;
#3579=FACE_OUTER_BOUND ( 'NONE', #415, .T. ) ;
#3585=EDGE_LOOP ( 'NONE', ( #2735, #3932, #12125, #5749 ) ) ;
#3586=LINE ( 'NONE', #7875, #3564 ) ;
#3587=ORIENTED_EDGE ( 'NONE', *, *, #9954, .F. ) ;
#3593=DIRECTION ( 'NONE',  ( 1.000000000000000000, 3.469446951953615372E-15, 0.000000000000000000 ) ) ;
#3594=CARTESIAN_POINT ( 'NONE',  ( 38.79999999999999716, 101.5999999999999943, -0.5000000000000000000 ) ) ;
#3595=ADVANCED_FACE ( 'NONE', ( #6139 ), #12388, .T. ) ;
#3598=CARTESIAN_POINT ( 'NONE',  ( -8.385254915620292238, 71.87811454074363837, -1.269264606320675724E-16 ) ) ;
#3600=ADVANCED_FACE ( 'NONE', ( #4943 ), #5180, .T. ) ;
#3601=CARTESIAN_POINT ( 'NONE',  ( 0.000000000000000000, 71.01020514433645303, -0.5000000000000000000 ) ) ;
#3609=CARTESIAN_POINT ( 'NONE',  ( -10.69346802281034847, -6.949821576306442594, -2.606381880848196280E-15 ) ) ;
#3611=CARTESIAN_POINT ( 'NONE',  ( -10.69381717166375800, 53.83378072214353693, -2.739695864762105467E-15 ) ) ;
#3616=EDGE_CURVE ( 'NONE', #11767, #5587, #8324, .T. ) ;
#3623=PRODUCT_DEFINITION_CONTEXT ( 'detailed design', #4587, 'design' ) ;
#3624=CARTESIAN_POINT ( 'NONE',  ( 4.259889153847074894, -78.36053266853434707, 9.185913434196624650 ) ) ;
#3627=VERTEX_POINT ( 'NONE', #11460 ) ;
#3631=ORIENTED_EDGE ( 'NONE', *, *, #6026, .T. ) ;
#3633=DIRECTION ( 'NONE',  ( -2.797435172181481150E-17, 1.000000000000000000, -1.765856845898762549E-18 ) ) ;
#3634=CARTESIAN_POINT ( 'NONE',  ( -9.661733384749148001, -70.21865067344228351, -3.001891213421562732 ) ) ;
#3636=CARTESIAN_POINT ( 'NONE',  ( 7.721449841176848849, -88.91797570967655417, -4.656840822883729913 ) ) ;
#3637=CARTESIAN_POINT ( 'NONE',  ( 10.69381717166375445, 16.13466892210585613, 1.286493866206055931E-15 ) ) ;
#3638=VERTEX_POINT ( 'NONE', #3958 ) ;
#3639=VECTOR ( 'NONE', #1251, 1000.000000000000000 ) ;
#3640=ORIENTED_EDGE ( 'NONE', *, *, #4741, .T. ) ;
#3643=CIRCLE ( 'NONE', #13347, 15.29705854078138749 ) ;
#3644=ORIENTED_EDGE ( 'NONE', *, *, #7132, .T. ) ;
#3647=CARTESIAN_POINT ( 'NONE',  ( -7.612107525059103041E-16, 27.21102387199583816, -4.805077278827845308E-17 ) ) ;
#3649=DIRECTION ( 'NONE',  ( -2.797435172181481150E-17, 1.000000000000000000, -1.765856845898762549E-18 ) ) ;
#3652=CARTESIAN_POINT ( 'NONE',  ( -1.423465862495650436, -128.7272727272635962, 3.918423281947951864 ) ) ;
#3654=CARTESIAN_POINT ( 'NONE',  ( -8.385254915620294014, 12.70483462268159869, -2.243491919447391838E-17 ) ) ;
#3655=CARTESIAN_POINT ( 'NONE',  ( 0.5078243831711967138, -154.2164502166737066, 1.847253022829126623 ) ) ;
#3656=DIRECTION ( 'NONE',  ( -2.797435172181481150E-17, 1.000000000000000000, -1.765856845898762549E-18 ) ) ;
#3657=CARTESIAN_POINT ( 'NONE',  ( -10.69346802281034492, 21.32451227372186864, -1.384884210559934224E-15 ) ) ;
#3659=ORIENTED_EDGE ( 'NONE', *, *, #10287, .T. ) ;
#3660=ORIENTED_EDGE ( 'NONE', *, *, #3858, .T. ) ;
#3662=CARTESIAN_POINT ( 'NONE',  ( 1.823996912523629943, -150.1972678403818122, -0.6830470970659942020 ) ) ;
#3665=CARTESIAN_POINT ( 'NONE',  ( -0.4120236738796625442, -101.0325188118372068, -7.520994285903035426 ) ) ;
#3669=CARTESIAN_POINT ( 'NONE',  ( -2.517691654963332357E-15, 90.00000000000000000, -1.589271161308885878E-16 ) ) ;
#3670=ORIENTED_EDGE ( 'NONE', *, *, #7148, .T. ) ;
#3672=DIRECTION ( 'NONE',  ( -2.797435172181481150E-17, 1.000000000000000000, -1.765856845898762549E-18 ) ) ;
#3673=CARTESIAN_POINT ( 'NONE',  ( -0.8895390116475855313, -145.6397668398474821, 2.172994011171002882 ) ) ;
#3674=CARTESIAN_POINT ( 'NONE',  ( 4.367873154833908700, 91.47215508561177444, -2.433639722925613924 ) ) ;
#3675=DIRECTION ( 'NONE',  ( 0.000000000000000000, 0.000000000000000000, 1.000000000000000000 ) ) ;
#3680=EDGE_CURVE ( 'NONE', #2958, #2969, #10254, .T. ) ;
#3681=CARTESIAN_POINT ( 'NONE',  ( 10.69346802281034847, -25.79937747632526879, 0.000000000000000000 ) ) ;
#3682=CARTESIAN_POINT ( 'NONE',  ( -8.385254915620292238, 15.32944684068712782, -1.081036776539837060E-15 ) ) ;
#3683=AXIS2_PLACEMENT_3D ( 'NONE', #1179, #9726, #8807 ) ;
#3684=ORIENTED_EDGE ( 'NONE', *, *, #12975, .T. ) ;
#3685=CARTESIAN_POINT ( 'NONE',  ( 3.917571877187554286, 90.55481622686230025, 3.109379165354180685 ) ) ;
#3686=VERTEX_POINT ( 'NONE', #7177 ) ;
#3687=CARTESIAN_POINT ( 'NONE',  ( 4.481549107982976565, -153.6493506492915628, -1.751282401325547022 ) ) ;
#3688=CIRCLE ( 'NONE', #5947, 8.385254915620292238 ) ;
#3689=ORIENTED_EDGE ( 'NONE', *, *, #969, .F. ) ;
#3690=CARTESIAN_POINT ( 'NONE',  ( -10.00000000000000000, 98.00000000000000000, -2.500000000000000000 ) ) ;
#3692=CARTESIAN_POINT ( 'NONE',  ( -12.02287503513836775, -157.8181818181456322, 0.9430477860708889049 ) ) ;
#3694=DIRECTION ( 'NONE',  ( -2.797435172181481150E-17, 1.000000000000000000, -1.765856845898762549E-18 ) ) ;
#3697=ADVANCED_FACE ( 'NONE', ( #10469 ), #3168, .T. ) ;
#3698=CARTESIAN_POINT ( 'NONE',  ( -10.69346802281034492, 21.32451227372186864, -1.384884210559934224E-15 ) ) ;
#3699=CARTESIAN_POINT ( 'NONE',  ( -14.13596196814457784, -39.17949320881311337, 28.27192393628914502 ) ) ;
#3700=STYLED_ITEM ( 'NONE', ( #11925 ), #7406 ) ;
#3702=EDGE_CURVE ( 'NONE', #2835, #11415, #5387, .T. ) ;
#3707=FACE_OUTER_BOUND ( 'NONE', #489, .T. ) ;
#3710=EDGE_CURVE ( 'NONE', #5877, #575, #4969, .T. ) ;
#3712=LINE ( 'NONE', #7846, #11108 ) ;
#3713=CARTESIAN_POINT ( 'NONE',  ( 0.1370278527897716703, -81.54378588852601695, -9.869404650674356461 ) ) ;
#3714=B_SPLINE_CURVE_WITH_KNOTS ( 'NONE', 3,
 ( #8484, #12457, #8426, #7300 ),
 .UNSPECIFIED., .F., .F.,
 ( 4, 4 ),
 ( 0.000000000000000000, 1.000000000000000000 ),
 .UNSPECIFIED. ) ;
#3715=CARTESIAN_POINT ( 'NONE',  ( -10.69381717166375623, -30.98922082794128485, -21.38763434332751956 ) ) ;
#3717=ORIENTED_EDGE ( 'NONE', *, *, #8736, .F. ) ;
#3718=EDGE_CURVE ( 'NONE', #10192, #357, #1070, .T. ) ;
#3719=VERTEX_POINT ( 'NONE', #7312 ) ;
#3725=CARTESIAN_POINT ( 'NONE',  ( -2.224254061606479205, -80.66666666666665719, 9.925145656127780214 ) ) ;
#3726=ORIENTED_EDGE ( 'NONE', *, *, #7911, .T. ) ;
#3728=DIRECTION ( 'NONE',  ( -1.000000000000000000, 0.000000000000000000, 0.000000000000000000 ) ) ;
#3729=B_SPLINE_CURVE_WITH_KNOTS ( 'NONE', 3,
 ( #9231, #7049, #7114, #8109 ),
 .UNSPECIFIED., .F., .F.,
 ( 4, 4 ),
 ( 0.000000000000000000, 1.000000000000000000 ),
 .UNSPECIFIED. ) ;
#3730=CARTESIAN_POINT ( 'NONE',  ( 6.459897978785722472, -117.0909090909104435, 0.7661034210344527251 ) ) ;
#3731=CARTESIAN_POINT ( 'NONE',  ( 12.99579180576516002, 45.23395377697383424, 25.99158361153033070 ) ) ;
#3733=CARTESIAN_POINT ( 'NONE',  ( 1.995220113909527360, -142.5800865799446058, 1.459423439933475564 ) ) ;
#3734=CYLINDRICAL_SURFACE ( 'NONE', #10851, 50.00000000000001421 ) ;
#3738=ORIENTED_EDGE ( 'NONE', *, *, #2009, .T. ) ;
#3739=CIRCLE ( 'NONE', #12256, 14.99999999999999112 ) ;
#3740=CARTESIAN_POINT ( 'NONE',  ( 1.669761519840590847, -153.2741505684571166, 0.4353783135838689700 ) ) ;
#3742=CARTESIAN_POINT ( 'NONE',  ( 0.1741682660668757709, -122.8707046542772616, 4.915355393405350881 ) ) ;
#3744=CARTESIAN_POINT ( 'NONE',  ( 0.000000000000000000, 71.01020514433645303, 2.500000000000000000 ) ) ;
#3747=DIRECTION ( 'NONE',  ( 0.000000000000000000, 0.000000000000000000, 1.000000000000000000 ) ) ;
#3752=PLANE ( 'NONE',  #9792 ) ;
#3753=CARTESIAN_POINT ( 'NONE',  ( -2.517691654963332357E-15, 90.00000000000000000, -1.589271161308885878E-16 ) ) ;
#3758=CARTESIAN_POINT ( 'NONE',  ( -8.723672207955784685, -129.7272727272731743, 9.720751085824094417 ) ) ;
#3759=EDGE_LOOP ( 'NONE', ( #13531, #13895, #13897, #3293 ) ) ;
#3760=ORIENTED_EDGE ( 'NONE', *, *, #4741, .F. ) ;
#3761=FACE_OUTER_BOUND ( 'NONE', #2918, .T. ) ;
#3762=( BOUNDED_SURFACE ( )  B_SPLINE_SURFACE ( 3, 3, ( 
 ( #7597, #120, #1095, #1231 ),
 ( #9847, #11947, #11745, #2200 ),
 ( #11880, #13024, #2406, #9645 ),
 ( #8791, #6488, #2133, #4307 ) ),
 .UNSPECIFIED., .F., .F., .T. ) 
 B_SPLINE_SURFACE_WITH_KNOTS ( ( 4, 4 ),
 ( 4, 4 ),
 ( 0.000000000000000000, 1.000000000000000000 ),
 ( 0.000000000000000000, 1.000000000000000000 ),
 .UNSPECIFIED. ) 
 GEOMETRIC_REPRESENTATION_ITEM ( )  RATIONAL_B_SPLINE_SURFACE ( (
 ( 1.000000000000000000, 0.3333333333333334259, 0.3333333333333334259, 1.000000000000000000),
 ( 1.000000000000000000, 0.3333333333333334259, 0.3333333333333334259, 1.000000000000000000),
 ( 1.000000000000000000, 0.3333333333333334259, 0.3333333333333334259, 1.000000000000000000),
 ( 1.000000000000000000, 0.3333333333333334259, 0.3333333333333334259, 1.000000000000000000) ) ) 
 REPRESENTATION_ITEM ( '' )  SURFACE ( )  );
#3765=CARTESIAN_POINT ( 'NONE',  ( 15.29705854078139282, 36.63580182200524149, -30.59411708156277854 ) ) ;
#3766=DIRECTION ( 'NONE',  ( -2.797435172181481150E-17, 1.000000000000000000, -1.765856845898762549E-18 ) ) ;
#3767=CARTESIAN_POINT ( 'NONE',  ( -10.69346802281034847, -35.22415542633469698, 21.38693604562069339 ) ) ;
#3768=CARTESIAN_POINT ( 'NONE',  ( 2.595030052768164897, -79.59366867652133237, 9.795566994422893359 ) ) ;
#3774=CARTESIAN_POINT ( 'NONE',  ( 8.385254915620297567, -24.99427717735608567, -16.77050983124058803 ) ) ;
#3778=ADVANCED_FACE ( 'NONE', ( #6402 ), #5640, .T. ) ;
#3782=CARTESIAN_POINT ( 'NONE',  ( -10.69346802281035558, 77.87317997377837742, 21.38693604562069694 ) ) ;
#3783=CARTESIAN_POINT ( 'NONE',  ( -9.243399937414574552, -71.03723845604672249, -4.118320465786138307 ) ) ;
#3785=CARTESIAN_POINT ( 'NONE',  ( 7.116416985698259090, -87.92852090411608401, -5.737785015158151758 ) ) ;
#3786=CARTESIAN_POINT ( 'NONE',  ( 12.99579180576516357, 16.95961992694555676, 1.563427368938892079E-15 ) ) ;
#3788=ORIENTED_EDGE ( 'NONE', *, *, #7724, .T. ) ;
#3789=AXIS2_PLACEMENT_3D ( 'NONE', #12515, #2899, #2971 ) ;
#3790=DIRECTION ( 'NONE',  ( -2.797435172181481150E-17, 1.000000000000000000, -1.765856845898762549E-18 ) ) ;
#3792=CARTESIAN_POINT ( 'NONE',  ( 1.376272962219654117, -80.66666666666658614, 10.07778225401747996 ) ) ;
#3794=CARTESIAN_POINT ( 'NONE',  ( 8.043602938545538095, -72.64880123058061656, 6.161478615796911029 ) ) ;
#3795=EDGE_CURVE ( 'NONE', #8398, #11958, #5477, .T. ) ;
#3796=CARTESIAN_POINT ( 'NONE',  ( 6.267146549263187261, -111.2727272727290142, -1.834821170859801009 ) ) ;
#3798=CARTESIAN_POINT ( 'NONE',  ( -12.99553232110413958, 11.07475474455194053, -1.630606568990249473E-15 ) ) ;
#3799=CARTESIAN_POINT ( 'NONE',  ( 4.114679947050920994, -133.0909090909029260, 0.08888163046386921007 ) ) ;
#3801=DIRECTION ( 'NONE',  ( 1.000000000000000000, 0.000000000000000000, 0.000000000000000000 ) ) ;
#3803=AXIS2_PLACEMENT_3D ( 'NONE', #9143, #8025, #1566 ) ;
#3805=CARTESIAN_POINT ( 'NONE',  ( -9.561354441693807661E-16, 34.17900274070598243, -6.035522597566817733E-17 ) ) ;
#3806=VERTEX_POINT ( 'NONE', #7579 ) ;
#3807=CARTESIAN_POINT ( 'NONE',  ( 4.962868326705308419, -115.9843930091672632, 2.901736775568028559 ) ) ;
#3808=DIRECTION ( 'NONE',  ( -1.000000000000000000, 0.000000000000000000, 0.000000000000000000 ) ) ;
#3813=ORIENTED_EDGE ( 'NONE', *, *, #12940, .F. ) ;
#3816=CARTESIAN_POINT ( 'NONE',  ( 3.290186468814228160, -129.2036444113705613, -2.543516287984220359 ) ) ;
#3817=EDGE_CURVE ( 'NONE', #3719, #12589, #2554, .T. ) ;
#3818=CIRCLE ( 'NONE', #2931, 14.99999999999998934 ) ;
#3820=DIRECTION ( 'NONE',  ( -0.000000000000000000, -0.000000000000000000, -1.000000000000000000 ) ) ;
#3821=LINE ( 'NONE', #12450, #9888 ) ;
#3826=CIRCLE ( 'NONE', #491, 24.99999999999998934 ) ;
#3827=ORIENTED_EDGE ( 'NONE', *, *, #2226, .F. ) ;
#3830=CARTESIAN_POINT ( 'NONE',  ( -2.139171520327136644, -164.3636363670092635, -0.7092570210252939766 ) ) ;
#3833=CARTESIAN_POINT ( 'NONE',  ( -1.288514859053046853E-15, 46.06057977201469100, -8.133639011647813827E-17 ) ) ;
#3836=CARTESIAN_POINT ( 'NONE',  ( -11.18807966363002215, -153.6493506493714563, 7.768796162323401866 ) ) ;
#3838=AXIS2_PLACEMENT_3D ( 'NONE', #11485, #2800, #8126 ) ;
#3844=ORIENTED_EDGE ( 'NONE', *, *, #13336, .T. ) ;
#3849=CARTESIAN_POINT ( 'NONE',  ( 41.99999999999999289, 120.0000000000000284, 2.500000000000000000 ) ) ;
#3851=CARTESIAN_POINT ( 'NONE',  ( -0.8141822005786675254, -105.2536593339433750, 6.965733946918862607 ) ) ;
#3853=CARTESIAN_POINT ( 'NONE',  ( 8.385254915620295790, -31.79444290936001138, 1.085359338644428786E-15 ) ) ;
#3855=ORIENTED_EDGE ( 'NONE', *, *, #5817, .T. ) ;
#3858=EDGE_CURVE ( 'NONE', #5091, #5381, #268, .T. ) ;
#3860=CARTESIAN_POINT ( 'NONE',  ( -10.69346802281034670, -25.79937747632526879, -1.218456123918935934E-15 ) ) ;
#3863=CARTESIAN_POINT ( 'NONE',  ( 9.704377265864934543, -70.11112484142813628, 2.862656032674172568 ) ) ;
#3864=( LENGTH_UNIT ( ) NAMED_UNIT ( * ) SI_UNIT ( .MILLI., .METRE. ) );
#3865=CARTESIAN_POINT ( 'NONE',  ( -10.69381717166375623, 44.40900277213413716, -1.466454780123922280E-15 ) ) ;
#3866=( BOUNDED_SURFACE ( )  B_SPLINE_SURFACE ( 3, 3, ( 
 ( #2328, #3178, #318, #1160 ),
 ( #1088, #4425, #11870, #1281 ),
 ( #11735, #10873, #1346, #12813 ),
 ( #9837, #8781, #13093, #5417 ) ),
 .UNSPECIFIED., .F., .F., .T. ) 
 B_SPLINE_SURFACE_WITH_KNOTS ( ( 4, 4 ),
 ( 4, 4 ),
 ( 0.000000000000000000, 1.000000000000000000 ),
 ( 0.000000000000000000, 1.000000000000000000 ),
 .UNSPECIFIED. ) 
 GEOMETRIC_REPRESENTATION_ITEM ( )  RATIONAL_B_SPLINE_SURFACE ( (
 ( 1.000000000000000000, 0.3333333333333334259, 0.3333333333333334259, 1.000000000000000000),
 ( 1.000000000000000000, 0.3333333333333334259, 0.3333333333333334259, 1.000000000000000000),
 ( 1.000000000000000000, 0.3333333333333334259, 0.3333333333333334259, 1.000000000000000000),
 ( 1.000000000000000000, 0.3333333333333334259, 0.3333333333333334259, 1.000000000000000000) ) ) 
 REPRESENTATION_ITEM ( '' )  SURFACE ( )  );
#3867=CARTESIAN_POINT ( 'NONE',  ( 2.301581772533156212, -133.0909090909184158, -3.282526544929044832 ) ) ;
#3869=EDGE_CURVE ( 'NONE', #13685, #6795, #7715, .T. ) ;
#3871=DIRECTION ( 'NONE',  ( -2.797435172181481150E-17, 1.000000000000000000, -1.765856845898762549E-18 ) ) ;
#3872=CIRCLE ( 'NONE', #2759, 15.29705854078138927 ) ;
#3877=CARTESIAN_POINT ( 'NONE',  ( 1.825346184638892089, -151.7272952153482493, -0.1028462948019921580 ) ) ;
#3881=CARTESIAN_POINT ( 'NONE',  ( -3.965212879745630747, -97.74628899555017369, -6.871886594889189404 ) ) ;
#3883=DIRECTION ( 'NONE',  ( 0.000000000000000000, 0.000000000000000000, 1.000000000000000000 ) ) ;
#3888=CARTESIAN_POINT ( 'NONE',  ( 0.01149510067628621221, -159.4799678529391826, -1.513478599014171477 ) ) ;
#3891=CARTESIAN_POINT ( 'NONE',  ( 10.69346802281035202, 2.474956373702985601, -21.38693604562069339 ) ) ;
#3894=CARTESIAN_POINT ( 'NONE',  ( 38.79999999999999716, 101.5999999999999943, -2.500000000000000000 ) ) ;
#3895=CARTESIAN_POINT ( 'NONE',  ( 12.99579180576516890, 64.08350967699263379, 3.183050967463143379E-15 ) ) ;
#3897=ORIENTED_EDGE ( 'NONE', *, *, #275, .F. ) ;
#3898=CARTESIAN_POINT ( 'NONE',  ( 4.067971666435306943, 90.77778941963205739, 2.909847887424534374 ) ) ;
#3901=VERTEX_POINT ( 'NONE', #6540 ) ;
#3902=VERTEX_POINT ( 'NONE', #7865 ) ;
#3904=CARTESIAN_POINT ( 'NONE',  ( -4.545447045960951726, 90.76293396533760927, -2.092248084982493594 ) ) ;
#3907=B_SPLINE_CURVE_WITH_KNOTS ( 'NONE', 3,
 ( #10543, #6339, #1015, #9433 ),
 .UNSPECIFIED., .F., .F.,
 ( 4, 4 ),
 ( 0.000000000000000000, 1.000000000000000000 ),
 .UNSPECIFIED. ) ;
#3908=CARTESIAN_POINT ( 'NONE',  ( -12.99579180576517068, 7.534841976936127672, 25.99158361153032359 ) ) ;
#3909=FACE_OUTER_BOUND ( 'NONE', #9734, .T. ) ;
#3912=CARTESIAN_POINT ( 'NONE',  ( -7.612107525059103041E-16, 27.21102387199583816, -4.805077278827845308E-17 ) ) ;
#3915=AXIS2_PLACEMENT_3D ( 'NONE', #13488, #1792, #9306 ) ;
#3919=CARTESIAN_POINT ( 'NONE',  ( 10.69381717166375978, -21.56444287793185310, -21.38763434332751245 ) ) ;
#3920=CIRCLE ( 'NONE', #11753, 15.29705854078139105 ) ;
#3921=VECTOR ( 'NONE', #8788, 1000.000000000000000 ) ;
#3922=CARTESIAN_POINT ( 'NONE',  ( 8.385254915620292238, -3.520109059331755219, 1.035430912652129043E-15 ) ) ;
#3923=CARTESIAN_POINT ( 'NONE',  ( -35.45454545454546036, 140.4866414850956744, 0.5000000000000000000 ) ) ;
#3924=CARTESIAN_POINT ( 'NONE',  ( 8.502150441026719463, -90.92014524198424397, -2.331827081617004360 ) ) ;
#3926=ORIENTED_EDGE ( 'NONE', *, *, #5869, .T. ) ;
#3928=VECTOR ( 'NONE', #5998, 1000.000000000000000 ) ;
#3929=CARTESIAN_POINT ( 'NONE',  ( 15.29705854078138927, 90.00000000000000000, 1.714422261702872766E-15 ) ) ;
#3930=CARTESIAN_POINT ( 'NONE',  ( -12.99553232110414491, -7.774801155466915858, -1.564035334333850472E-15 ) ) ;
#3932=ORIENTED_EDGE ( 'NONE', *, *, #11602, .F. ) ;
#3933=CARTESIAN_POINT ( 'NONE',  ( -4.318061424038324603, 91.66495677434029687, -2.521242278247964208 ) ) ;
#3935=ORIENTED_EDGE ( 'NONE', *, *, #11692, .T. ) ;
#3940=CIRCLE ( 'NONE', #7509, 22.99999999999999645 ) ;
#3943=CARTESIAN_POINT ( 'NONE',  ( -1.158071465989066962, -149.5103943980214467, -1.626766656952254086 ) ) ;
#3945=VECTOR ( 'NONE', #12804, 1000.000000000000000 ) ;
#3946=EDGE_LOOP ( 'NONE', ( #13145, #13172, #3349, #11716 ) ) ;
#3948=ORIENTED_EDGE ( 'NONE', *, *, #5469, .T. ) ;
#3949=CARTESIAN_POINT ( 'NONE',  ( 5.923806222615441541, -113.5015096987964114, 0.9909073766846139275 ) ) ;
#3952=FACE_OUTER_BOUND ( 'NONE', #223, .T. ) ;
#3953=ORIENTED_EDGE ( 'NONE', *, *, #571, .T. ) ;
#3958=CARTESIAN_POINT ( 'NONE',  ( 15.29705854078139282, 8.361467971976981772, 1.856918518244840178E-15 ) ) ;
#3965=DIRECTION ( 'NONE',  ( 0.000000000000000000, 0.000000000000000000, 1.000000000000000000 ) ) ;
#3968=VERTEX_POINT ( 'NONE', #10935 ) ;
#3969=CARTESIAN_POINT ( 'NONE',  ( -19.28867027886077068, -167.3636363460783798, 6.559046148772988083 ) ) ;
#3970=ORIENTED_EDGE ( 'NONE', *, *, #13162, .F. ) ;
#3972=CARTESIAN_POINT ( 'NONE',  ( -4.961404791891401267, 89.99999999999998579, -0.6346456166747422856 ) ) ;
#3974=CARTESIAN_POINT ( 'NONE',  ( 1.026257021570081918, -73.45454546207005819, 21.46608457194884068 ) ) ;
#3975=CARTESIAN_POINT ( 'NONE',  ( 8.385254915620290461, 34.17900274070598243, -16.77050983124057737 ) ) ;
#3976=EDGE_CURVE ( 'NONE', #2454, #3686, #2202, .T. ) ;
#3977=CARTESIAN_POINT ( 'NONE',  ( -10.69346802281035380, 49.59884612375012836, 21.38693604562069339 ) ) ;
#3978=CARTESIAN_POINT ( 'NONE',  ( -8.385254915620292238, 15.32944684068712782, -2.706960864746847057E-17 ) ) ;
#3979=CARTESIAN_POINT ( 'NONE',  ( -1.410017725396658984E-15, 50.40394642271930792, -8.900615385087330109E-17 ) ) ;
#3982=CARTESIAN_POINT ( 'NONE',  ( -10.69381717166375267, -12.13966492792242846, -21.38763434332751601 ) ) ;
#3984=EDGE_CURVE ( 'NONE', #13867, #11837, #12052, .T. ) ;
#3986=CARTESIAN_POINT ( 'NONE',  ( -15.29705854078139282, -1.063309978032445979, -3.758510681017264029E-15 ) ) ;
#3987=DIRECTION ( 'NONE',  ( -2.797435172181481150E-17, 1.000000000000000000, -1.765856845898762549E-18 ) ) ;
#3988=CARTESIAN_POINT ( 'NONE',  ( 0.1949906707164464070, -155.7802847986947654, 1.574602209766050143 ) ) ;
#3990=CYLINDRICAL_SURFACE ( 'NONE', #6459, 15.29705854078139105 ) ;
#3994=EDGE_LOOP ( 'NONE', ( #9587, #3999, #10983, #8139 ) ) ;
#3995=CARTESIAN_POINT ( 'NONE',  ( -10.69381717166375800, -12.13966492792242846, -1.266741076154724095E-15 ) ) ;
#3999=ORIENTED_EDGE ( 'NONE', *, *, #6941, .T. ) ;
#4000=LINE ( 'NONE', #2098, #8577 ) ;
#4001=VECTOR ( 'NONE', #11166, 1000.000000000000114 ) ;
#4003=CARTESIAN_POINT ( 'NONE',  ( -1.146365672123090463E-15, 40.97916847270985130, -7.236334518677345233E-17 ) ) ;
#4004=CARTESIAN_POINT ( 'NONE',  ( -6.190615655759536180E-16, 22.12961257269105531, -3.907772785857374249E-17 ) ) ;
#4005=CARTESIAN_POINT ( 'NONE',  ( 3.905416522049567796, -121.2486883143391481, 3.232865067491931921 ) ) ;
#4006=CYLINDRICAL_SURFACE ( 'NONE', #12909, 14.99999999999998934 ) ;
#4008=ADVANCED_FACE ( 'NONE', ( #8148 ), #6460, .T. ) ;
#4009=ORIENTED_EDGE ( 'NONE', *, *, #5084, .T. ) ;
#4010=ORIENTED_EDGE ( 'NONE', *, *, #8489, .T. ) ;
#4011=CARTESIAN_POINT ( 'NONE',  ( 0.1084562595890940784, -143.6327608500317012, -2.541581260578934742 ) ) ;
#4016=DIRECTION ( 'NONE',  ( 2.797435172181480534E-17, -1.000000000000000000, 1.765856845898762164E-18 ) ) ;
#4017=CARTESIAN_POINT ( 'NONE',  ( -5.728966446173876292, -108.7068931125657087, 3.285836578437095756 ) ) ;
#4018=AXIS2_PLACEMENT_3D ( 'NONE', #9966, #649, #12283 ) ;
#4019=CARTESIAN_POINT ( 'NONE',  ( 10.11144057928414242, -69.99977036137985920, -0.2534939170199681513 ) ) ;
#4020=DIRECTION ( 'NONE',  ( -2.797435172181481150E-17, 1.000000000000000000, -1.765856845898762549E-18 ) ) ;
#4022=DIRECTION ( 'NONE',  ( 1.000000000000000000, 0.000000000000000000, 0.000000000000000000 ) ) ;
#4023=CARTESIAN_POINT ( 'NONE',  ( 10.69381717166375623, -2.714886977913000266, 0.000000000000000000 ) ) ;
#4026=DIRECTION ( 'NONE',  ( -2.797435172181481150E-17, 1.000000000000000000, -1.765856845898762549E-18 ) ) ;
#4033=EDGE_LOOP ( 'NONE', ( #7053, #12030, #4009, #6536, #7237, #5949 ) ) ;
#4036=ORIENTED_EDGE ( 'NONE', *, *, #6337, .T. ) ;
#4039=CARTESIAN_POINT ( 'NONE',  ( -2.339066459587731637E-16, 8.361467971976981772, -1.476515546007874940E-17 ) ) ;
#4040=CARTESIAN_POINT ( 'NONE',  ( -3.722721133223385603, -134.6363636363710725, 2.741844555832380070 ) ) ;
#4042=CYLINDRICAL_SURFACE ( 'NONE', #4941, 15.29705854078139460 ) ;
#4045=CARTESIAN_POINT ( 'NONE',  ( 10.69381717166376333, -30.98922082794128130, 0.000000000000000000 ) ) ;
#4046=AXIS2_PLACEMENT_3D ( 'NONE', #10265, #5006, #8140 ) ;
#4051=EDGE_CURVE ( 'NONE', #9012, #10192, #7939, .T. ) ;
#4052=CIRCLE ( 'NONE', #705, 5.000000000000000000 ) ;
#4053=AXIS2_PLACEMENT_3D ( 'NONE', #3805, #1635, #4721 ) ;
#4055=DIRECTION ( 'NONE',  ( -1.000000000000000000, 0.000000000000000000, 0.000000000000000000 ) ) ;
#4058=CARTESIAN_POINT ( 'NONE',  ( 15.29705854078139282, -1.063309978032445091, 1.888916609591544936E-15 ) ) ;
#4059=CARTESIAN_POINT ( 'NONE',  ( -0.1852015970780942489, -159.9999997928953235, 1.488522644435750886 ) ) ;
#4060=CARTESIAN_POINT ( 'NONE',  ( -15.29705854078138749, 47.94714734142005597, -30.59411708156277854 ) ) ;
#4065=DIRECTION ( 'NONE',  ( -1.000000000000000000, -2.797435172181480534E-17, 0.000000000000000000 ) ) ;
#4066=ORIENTED_EDGE ( 'NONE', *, *, #11940, .T. ) ;
#4067=VERTEX_POINT ( 'NONE', #7092 ) ;
#4068=FACE_OUTER_BOUND ( 'NONE', #4850, .T. ) ;
#4072=DIRECTION ( 'NONE',  ( 1.000000000000000000, 0.000000000000000000, 0.000000000000000000 ) ) ;
#4075=CARTESIAN_POINT ( 'NONE',  ( -2.980405791994721554, -137.4311428799600492, 1.166279635936706693 ) ) ;
#4076=CARTESIAN_POINT ( 'NONE',  ( -8.385254915620294014, 90.00000000000000000, -1.589271161308885878E-16 ) ) ;
#4079=ORIENTED_EDGE ( 'NONE', *, *, #1818, .T. ) ;
#4083=CARTESIAN_POINT ( 'NONE',  ( -6.172719407040554884, -110.2881872775037237, 1.857052143282659440 ) ) ;
#4086=AXIS2_PLACEMENT_3D ( 'NONE', #6629, #2415, #6694 ) ;
#4088=CARTESIAN_POINT ( 'NONE',  ( -10.69346802281034314, 2.474956373702985157, -21.38693604562069694 ) ) ;
#4094=VECTOR ( 'NONE', #12191, 1000.000000000000000 ) ;
#4096=CARTESIAN_POINT ( 'NONE',  ( -8.931512003262966459, -153.6493506494496160, 10.28374512068630686 ) ) ;
#4099=B_SPLINE_CURVE_WITH_KNOTS ( 'NONE', 3,
 ( #119, #12952, #6556, #6686 ),
 .UNSPECIFIED., .F., .F.,
 ( 4, 4 ),
 ( 0.000000000000000000, 1.000000000000000000 ),
 .UNSPECIFIED. ) ;
#4100=CARTESIAN_POINT ( 'NONE',  ( -15.29705854078139460, -10.48808792804187284, 30.59411708156277854 ) ) ;
#4101=ORIENTED_EDGE ( 'NONE', *, *, #7999, .F. ) ;
#4103=DIRECTION ( 'NONE',  ( -1.000000000000000000, 0.000000000000000000, 0.000000000000000000 ) ) ;
#4106=CARTESIAN_POINT ( 'NONE',  ( -3.345128319330075151, -82.89610389611301855, 14.18235785815877037 ) ) ;
#4107=FACE_OUTER_BOUND ( 'NONE', #12568, .T. ) ;
#4109=CARTESIAN_POINT ( 'NONE',  ( 8.385254915620295790, -31.79444290936001138, 1.085359338644428786E-15 ) ) ;
#4110=CARTESIAN_POINT ( 'NONE',  ( 11.81226048336476531, -40.00941361824966691, 23.62452096672953061 ) ) ;
#4116=DIRECTION ( 'NONE',  ( 0.000000000000000000, 1.000000000000000000, 0.000000000000000000 ) ) ;
#4119=FACE_OUTER_BOUND ( 'NONE', #1071, .T. ) ;
#4120=ADVANCED_FACE ( 'NONE', ( #5985 ), #8508, .T. ) ;
#4122=EDGE_CURVE ( 'NONE', #6577, #11197, #5120, .T. ) ;
#4123=CARTESIAN_POINT ( 'NONE',  ( -3.237931855445342677, -122.4890033182045812, -3.753960870359740465 ) ) ;
#4126=ORIENTED_EDGE ( 'NONE', *, *, #5929, .T. ) ;
#4128=CIRCLE ( 'NONE', #11305, 2.000000000000000000 ) ;
#4129=CARTESIAN_POINT ( 'NONE',  ( -4.067971666435313161, 90.77778941963205739, -2.909847887424534374 ) ) ;
#4132=CARTESIAN_POINT ( 'NONE',  ( 15.29705854078139460, -38.76242177807012723, -30.59411708156277498 ) ) ;
#4135=CARTESIAN_POINT ( 'NONE',  ( -8.385254915620297567, 31.55439052270045508, -5.572053652267360357E-17 ) ) ;
#4137=CARTESIAN_POINT ( 'NONE',  ( 8.385254915620292238, 22.12961257269105531, 9.855024866598291022E-16 ) ) ;
#4141=CARTESIAN_POINT ( 'NONE',  ( -0.2126761085232016235, -104.1813795433902214, -7.142456545591105765 ) ) ;
#4144=ORIENTED_EDGE ( 'NONE', *, *, #8510, .F. ) ;
#4145=VERTEX_POINT ( 'NONE', #9608 ) ;
#4147=( GEOMETRIC_REPRESENTATION_CONTEXT ( 3 ) GLOBAL_UNCERTAINTY_ASSIGNED_CONTEXT ( ( #10363 ) ) GLOBAL_UNIT_ASSIGNED_CONTEXT ( ( #3864, #1696, #10322 ) ) REPRESENTATION_CONTEXT ( 'NONE', 'WORKASPACE' ) );
#4148=VERTEX_POINT ( 'NONE', #5325 ) ;
#4150=AXIS2_PLACEMENT_3D ( 'NONE', #13789, #729, #11579 ) ;
#4151=CARTESIAN_POINT ( 'NONE',  ( -2.517691654963332357E-15, 90.00000000000000000, -1.589271161308885878E-16 ) ) ;
#4152=CARTESIAN_POINT ( 'NONE',  ( -0.4106197315061012598, -101.8078744002022944, 7.425433182683227606 ) ) ;
#4153=CARTESIAN_POINT ( 'NONE',  ( -1.214590548353025268, -168.0000000000001421, 1.662759693958066221 ) ) ;
#4154=CARTESIAN_POINT ( 'NONE',  ( 8.385254915620290461, 62.45333659073423860, 9.631531405059305263E-16 ) ) ;
#4157=CIRCLE ( 'NONE', #7066, 71.99999999999998579 ) ;
#4158=CARTESIAN_POINT ( 'NONE',  ( 12.99553232110414847, 1.649976794542512337, -25.99106464220827917 ) ) ;
#4159=CARTESIAN_POINT ( 'NONE',  ( -8.385254915620294014, -15.56949922734665570, -9.719105456492490422E-16 ) ) ;
#4163=CARTESIAN_POINT ( 'NONE',  ( 3.345128319332408839, -82.89610389611962660, -14.18235785815831917 ) ) ;
#4165=CARTESIAN_POINT ( 'NONE',  ( 10.69381717166375800, -12.13966492792242846, 2.619229793989004345E-15 ) ) ;
#4166=ORIENTED_EDGE ( 'NONE', *, *, #6323, .F. ) ;
#4168=DIRECTION ( 'NONE',  ( 1.000000000000000000, 0.000000000000000000, 0.000000000000000000 ) ) ;
#4170=CARTESIAN_POINT ( 'NONE',  ( 0.01432886326166990174, -82.89610389604476381, 5.147384767213183387 ) ) ;
#4171=DIRECTION ( 'NONE',  ( -0.000000000000000000, -0.000000000000000000, -1.000000000000000000 ) ) ;
#4173=DIRECTION ( 'NONE',  ( 0.1234677578012386562, 1.701584941912606716E-18, -0.9923485843107423543 ) ) ;
#4177=EDGE_LOOP ( 'NONE', ( #10448, #3717, #3659, #13376 ) ) ;
#4179=ORIENTED_EDGE ( 'NONE', *, *, #1120, .T. ) ;
#4180=CARTESIAN_POINT ( 'NONE',  ( -2.303009741871944172E-17, 0.8232575913728890082, -1.453755053663958216E-18 ) ) ;
#4182=CARTESIAN_POINT ( 'NONE',  ( -8.385254915620297567, 31.55439052270045508, -2.137983544802758185E-15 ) ) ;
#4184=CARTESIAN_POINT ( 'NONE',  ( -1.899183197727328576, -124.6925521901340090, -4.281368322782853397 ) ) ;
#4186=ORIENTED_EDGE ( 'NONE', *, *, #1543, .T. ) ;
#4187=EDGE_CURVE ( 'NONE', #1478, #5877, #9380, .T. ) ;
#4190=EDGE_CURVE ( 'NONE', #1478, #10661, #428, .T. ) ;
#4191=CARTESIAN_POINT ( 'NONE',  ( -3.632360187558554721, 90.29910261214918421, -3.439149220787172556 ) ) ;
#4193=CARTESIAN_POINT ( 'NONE',  ( -14.13596196814457429, -39.17949320881311337, -3.385655485371662251E-15 ) ) ;
#4196=( BOUNDED_SURFACE ( )  B_SPLINE_SURFACE ( 3, 3, ( 
 ( #4470, #2366, #8547, #9809 ),
 ( #5323, #13061, #3285, #10910 ),
 ( #10651, #7694, #4540, #5454 ),
 ( #6650, #3350, #8819, #12849 ) ),
 .UNSPECIFIED., .F., .F., .T. ) 
 B_SPLINE_SURFACE_WITH_KNOTS ( ( 4, 4 ),
 ( 4, 4 ),
 ( 0.000000000000000000, 1.000000000000000000 ),
 ( 0.000000000000000000, 1.000000000000000000 ),
 .UNSPECIFIED. ) 
 GEOMETRIC_REPRESENTATION_ITEM ( )  RATIONAL_B_SPLINE_SURFACE ( (
 ( 1.000000000000000000, 0.3333333333333334259, 0.3333333333333334259, 1.000000000000000000),
 ( 1.000000000000000000, 0.3333333333333334259, 0.3333333333333334259, 1.000000000000000000),
 ( 1.000000000000000000, 0.3333333333333334259, 0.3333333333333334259, 1.000000000000000000),
 ( 1.000000000000000000, 0.3333333333333334259, 0.3333333333333334259, 1.000000000000000000) ) ) 
 REPRESENTATION_ITEM ( '' )  SURFACE ( )  );
#4197=B_SPLINE_CURVE_WITH_KNOTS ( 'NONE', 3,
 ( #12316, #11037, #5713, #10960 ),
 .UNSPECIFIED., .F., .F.,
 ( 4, 4 ),
 ( 0.000000000000000000, 1.000000000000000000 ),
 .UNSPECIFIED. ) ;
#4199=CARTESIAN_POINT ( 'NONE',  ( -3.469499288793235436, -73.45454545754009246, -20.14723442201650272 ) ) ;
#4203=CARTESIAN_POINT ( 'NONE',  ( -0.1946493556060955588, -155.7833351585698267, -1.574489734363575311 ) ) ;
#4204=DIRECTION ( 'NONE',  ( 1.000000000000000000, 0.000000000000000000, 0.000000000000000000 ) ) ;
#4207=ORIENTED_EDGE ( 'NONE', *, *, #11602, .T. ) ;
#4209=AXIS2_PLACEMENT_3D ( 'NONE', #13529, #3871, #8152 ) ;
#4215=CARTESIAN_POINT ( 'NONE',  ( -10.69346802281034670, 40.17406817374066463, -2.714638868194240665E-15 ) ) ;
#4216=CARTESIAN_POINT ( 'NONE',  ( 8.874474818771595608, -89.41029592820135008, -1.238859673556061525 ) ) ;
#4219=CARTESIAN_POINT ( 'NONE',  ( -10.17548876272777036, -70.78787878787981924, -0.6371443735352790849 ) ) ;
#4220=AXIS2_PLACEMENT_3D ( 'NONE', #3979, #8256, #9720 ) ;
#4221=CARTESIAN_POINT ( 'NONE',  ( 3.621248221984613947E-16, -12.94488700934118341, 2.285881734483108495E-17 ) ) ;
#4222=CARTESIAN_POINT ( 'NONE',  ( -10.69346802281034847, 30.74929022373126841, -1.418169827888134119E-15 ) ) ;
#4225=CARTESIAN_POINT ( 'NONE',  ( 25.00000000000000355, 120.0000000000000284, -2.500000000000000000 ) ) ;
#4227=CARTESIAN_POINT ( 'NONE',  ( -4.154595973944807064, -61.00000000000002842, 0.9946518452611590178 ) ) ;
#4229=ORIENTED_EDGE ( 'NONE', *, *, #6100, .F. ) ;
#4233=DIRECTION ( 'NONE',  ( 0.000000000000000000, 0.000000000000000000, 1.000000000000000000 ) ) ;
#4236=CARTESIAN_POINT ( 'NONE',  ( 12.09338464843078143, -60.99999999999997158, -0.006909782851249028461 ) ) ;
#4237=DIRECTION ( 'NONE',  ( 1.000000000000000000, 0.000000000000000000, 0.000000000000000000 ) ) ;
#4238=CARTESIAN_POINT ( 'NONE',  ( 8.385254915620295790, 12.70483462268160046, -16.77050983124058448 ) ) ;
#4245=ORIENTED_EDGE ( 'NONE', *, *, #1974, .T. ) ;
#4248=EDGE_LOOP ( 'NONE', ( #663, #6417, #9350, #4126 ) ) ;
#4253=CARTESIAN_POINT ( 'NONE',  ( -25.00000000000000355, 120.0000000000000284, 2.500000000000000000 ) ) ;
#4255=CARTESIAN_POINT ( 'NONE',  ( 1.160247953126058107, -149.4998025384539915, 1.626383737532501650 ) ) ;
#4256=CARTESIAN_POINT ( 'NONE',  ( -15.29705854078138927, 10.24803554138234318, 30.59411708156276788 ) ) ;
#4258=AXIS2_PLACEMENT_3D ( 'NONE', #7449, #2120, #4022 ) ;
#4262=DIRECTION ( 'NONE',  ( -1.000000000000000000, 0.000000000000000000, 0.000000000000000000 ) ) ;
#4266=FACE_OUTER_BOUND ( 'NONE', #392, .T. ) ;
#4267=EDGE_CURVE ( 'NONE', #7855, #10906, #1980, .T. ) ;
#4268=CARTESIAN_POINT ( 'NONE',  ( 0.000000000000000000, 71.01020514433645303, 0.5000000000000000000 ) ) ;
#4271=CARTESIAN_POINT ( 'NONE',  ( -1.381416026885722292, -78.35919761624415969, -10.01283214670341160 ) ) ;
#4273=CARTESIAN_POINT ( 'NONE',  ( -1.552166912326615374E-15, 55.48535772202409078, -9.797919878057798703E-17 ) ) ;
#4274=LINE ( 'NONE', #7047, #10019 ) ;
#4276=CARTESIAN_POINT ( 'NONE',  ( 1.792607291163630601, -80.16257883281073759, 9.968655783465312226 ) ) ;
#4278=VERTEX_POINT ( 'NONE', #12648 ) ;
#4279=VERTEX_POINT ( 'NONE', #7296 ) ;
#4280=ORIENTED_EDGE ( 'NONE', *, *, #207, .T. ) ;
#4281=B_SPLINE_SURFACE_WITH_KNOTS ( 'NONE', 3, 3, ( 
 ( #1985, #13539, #8232, #4153 ),
 ( #5140, #745, #5009, #9289 ),
 ( #12520, #13604, #2904, #11459 ),
 ( #10408, #808, #13671, #2974 ),
 ( #7243, #11527, #1919, #6208 ),
 ( #10468, #8567, #11793, #8772 ),
 ( #2183, #10934, #10670, #13083 ),
 ( #7444, #9627, #1078, #13871 ),
 ( #11725, #5476, #2114, #12870 ),
 ( #5408, #96, #8633, #5838 ),
 ( #8841, #3652, #7782, #4787 ),
 ( #9064, #11012, #13380, #13151 ),
 ( #3730, #8014, #3499, #12291 ),
 ( #2463, #2681, #3796, #12366 ),
 ( #2750, #6743, #5690, #9974 ),
 ( #385, #7091, #4990, #9478 ),
 ( #5061, #3084, #9343, #13653 ),
 ( #12579, #1903, #6190, #10456 ),
 ( #5984, #9409, #7352, #3026 ),
 ( #991, #12821, #828, #11676 ),
 ( #8322, #890, #3118, #9449 ),
 ( #7327, #1941, #5094, #10559 ),
 ( #3188, #13695, #1795, #3974 ),
 ( #6225, #13822, #9378, #10358 ) ),
 .UNSPECIFIED., .F., .F., .F.,
 ( 4, 1, 1, 1, 1, 1, 1, 1, 1, 1, 1, 1, 1, 1, 1, 1, 1, 1, 1, 1, 1, 4 ),
 ( 4, 4 ),
 ( -0.1668267180224854429, -0.1624291228870498593, -0.1587644602741868916, -0.1580315277516142758, -0.1536339326161787200, -0.1471422445591071271, -0.1404411472098719693, -0.1360435520744363858, -0.1316459569390008300, -0.1272483618035652464, -0.1228507666681296628, -0.1140555763972584957, -0.1096579812618229260, -0.1052603861263873425, -0.1008627909909517728, -0.09646519585551618925, -0.08976409850628104536, -0.08327241044920945245, -0.07887481531377388277, -0.07814188279120128089, -0.07447722017833829922, -0.07007962504290271566 ),
 ( 0.003200000000000001888, 0.006800000000000002223 ),
 .UNSPECIFIED. ) ;
#4284=CARTESIAN_POINT ( 'NONE',  ( 8.385254915620294014, 40.97916847270985130, 9.905219695108654260E-16 ) ) ;
#4285=CARTESIAN_POINT ( 'NONE',  ( 7.223390746404686702, -85.44318711194655691, -6.107340895223999588 ) ) ;
#4286=ADVANCED_FACE ( 'NONE', ( #13853, #3027 ), #12711, .T. ) ;
#4289=EDGE_CURVE ( 'NONE', #1176, #1421, #9813, .T. ) ;
#4291=CARTESIAN_POINT ( 'NONE',  ( -15.29705854078139460, -27.45107625865536605, 4.847467093863555185E-17 ) ) ;
#4292=CARTESIAN_POINT ( 'NONE',  ( -5.783440176334588401, -75.54545454545275618, -8.231660884606981199 ) ) ;
#4296=EDGE_CURVE ( 'NONE', #13011, #6322, #645, .T. ) ;
#4301=DIRECTION ( 'NONE',  ( -2.797435172181481150E-17, 1.000000000000000000, -1.765856845898762549E-18 ) ) ;
#4303=DIRECTION ( 'NONE',  ( -2.797435172181481150E-17, 1.000000000000000000, -1.765856845898762549E-18 ) ) ;
#4305=CARTESIAN_POINT ( 'NONE',  ( 25.00000000000000355, 120.0000000000000284, -0.5000000000000000000 ) ) ;
#4306=CARTESIAN_POINT ( 'NONE',  ( 0.000000000000000000, 71.01020514433645303, 2.500000000000000000 ) ) ;
#4307=CARTESIAN_POINT ( 'NONE',  ( 15.29705854078139637, 0.8232575913729167638, 3.746698755667523989E-15 ) ) ;
#4309=CARTESIAN_POINT ( 'NONE',  ( -12.05308885558866550, -134.6363636363568901, 5.101645771607369539 ) ) ;
#4310=CARTESIAN_POINT ( 'NONE',  ( -8.385254915620295790, 24.75422479069652582, -2.113967306380547611E-15 ) ) ;
#4311=CARTESIAN_POINT ( 'NONE',  ( 10.69381717166375800, -21.56444287793185666, 0.000000000000000000 ) ) ;
#4314=AXIS2_PLACEMENT_3D ( 'NONE', #4324, #8744, #6569 ) ;
#4316=EDGE_LOOP ( 'NONE', ( #3726, #8280, #12512, #8695 ) ) ;
#4320=CARTESIAN_POINT ( 'NONE',  ( 15.29705854078139105, 46.06057977201469100, 1.790347283588440782E-15 ) ) ;
#4322=DIRECTION ( 'NONE',  ( -2.797435172181481150E-17, 1.000000000000000000, -1.765856845898762549E-18 ) ) ;
#4324=CARTESIAN_POINT ( 'NONE',  ( -2.200973885217364349E-15, 78.67828027274755698, -1.389345798431728350E-16 ) ) ;
#4325=LINE ( 'NONE', #8606, #11617 ) ;
#4326=EDGE_LOOP ( 'NONE', ( #5462, #135, #6632, #3827 ) ) ;
#4329=DIRECTION ( 'NONE',  ( -1.000000000000000000, 0.000000000000000000, 0.000000000000000000 ) ) ;
#4332=CARTESIAN_POINT ( 'NONE',  ( -5.938565187887739683, -74.76276780260269561, -8.199189674694745023 ) ) ;
#4334=FACE_OUTER_BOUND ( 'NONE', #13293, .T. ) ;
#4335=CARTESIAN_POINT ( 'NONE',  ( -2.227027882156173089, -83.13467912880821586, 9.407963499362976378 ) ) ;
#4341=AXIS2_PLACEMENT_3D ( 'NONE', #2853, #7127, #13625 ) ;
#4349=CARTESIAN_POINT ( 'NONE',  ( 15.29705854078139105, 8.361467971976955127, 1.858555455282030396E-15 ) ) ;
#4353=CARTESIAN_POINT ( 'NONE',  ( 0.5850150888149016071, -160.9696969693212623, -1.917718896954408336 ) ) ;
#4354=CARTESIAN_POINT ( 'NONE',  ( -4.840675591955100110, -75.54545454545453254, -8.982239580829959991 ) ) ;
#4358=VERTEX_POINT ( 'NONE', #11777 ) ;
#4360=CARTESIAN_POINT ( 'NONE',  ( 12.99553232110414491, 1.649976794542512559, 0.000000000000000000 ) ) ;
#4362=ORIENTED_EDGE ( 'NONE', *, *, #6470, .T. ) ;
#4364=EDGE_CURVE ( 'NONE', #6810, #8545, #12743, .T. ) ;
#4365=CYLINDRICAL_SURFACE ( 'NONE', #8179, 15.29705854078139105 ) ;
#4368=EDGE_CURVE ( 'NONE', #1714, #4148, #12050, .T. ) ;
#4369=ORIENTED_EDGE ( 'NONE', *, *, #4899, .T. ) ;
#4370=DIRECTION ( 'NONE',  ( -2.797435172181481150E-17, 1.000000000000000000, -1.765856845898762549E-18 ) ) ;
#4371=AXIS2_PLACEMENT_3D ( 'NONE', #8289, #7234, #11584 ) ;
#4372=EDGE_CURVE ( 'NONE', #10190, #9777, #5385, .T. ) ;
#4374=CARTESIAN_POINT ( 'NONE',  ( 15.29705854078139282, 55.48535772202409788, -30.59411708156277854 ) ) ;
#4376=DIRECTION ( 'NONE',  ( -2.797435172181481150E-17, 1.000000000000000000, -1.765856845898762549E-18 ) ) ;
#4379=CYLINDRICAL_SURFACE ( 'NONE', #4086, 8.385254915620295790 ) ;
#4382=ORIENTED_EDGE ( 'NONE', *, *, #7402, .T. ) ;
#4384=ORIENTED_EDGE ( 'NONE', *, *, #8558, .T. ) ;
#4387=EDGE_LOOP ( 'NONE', ( #459, #9617, #3225, #6736 ) ) ;
#4394=ORIENTED_EDGE ( 'NONE', *, *, #5316, .F. ) ;
#4395=ORIENTED_EDGE ( 'NONE', *, *, #5133, .F. ) ;
#4396=ADVANCED_FACE ( 'NONE', ( #8684 ), #13127, .F. ) ;
#4397=EDGE_LOOP ( 'NONE', ( #11029, #9398, #8543, #9771 ) ) ;
#4399=ORIENTED_EDGE ( 'NONE', *, *, #4817, .F. ) ;
#4403=DIRECTION ( 'NONE',  ( -2.797435172181481150E-17, 1.000000000000000000, -1.765856845898762549E-18 ) ) ;
#4405=CARTESIAN_POINT ( 'NONE',  ( 8.385254915620294014, 24.75422479069652582, 9.855024866598292994E-16 ) ) ;
#4406=EDGE_LOOP ( 'NONE', ( #1490, #8222, #10555, #8448 ) ) ;
#4407=B_SPLINE_CURVE_WITH_KNOTS ( 'NONE', 3,
 ( #12183, #6704, #6853, #7678 ),
 .UNSPECIFIED., .F., .F.,
 ( 4, 4 ),
 ( 0.000000000000000000, 1.000000000000000000 ),
 .UNSPECIFIED. ) ;
#4412=CARTESIAN_POINT ( 'NONE',  ( -15.29705854078139460, -1.063309978032445979, 30.59411708156277854 ) ) ;
#4418=CARTESIAN_POINT ( 'NONE',  ( -3.188279143310615904, -76.81818181818212565, -9.710576830322478870 ) ) ;
#4419=EDGE_CURVE ( 'NONE', #4551, #5287, #13665, .T. ) ;
#4423=EDGE_LOOP ( 'NONE', ( #6880, #601, #9700, #3451 ) ) ;
#4424=FACE_OUTER_BOUND ( 'NONE', #3284, .T. ) ;
#4425=CARTESIAN_POINT ( 'NONE',  ( 12.99579180576517068, 73.50828762700210461, -25.99158361153033070 ) ) ;
#4429=PLANE ( 'NONE',  #12561 ) ;
#4434=AXIS2_PLACEMENT_3D ( 'NONE', #9037, #10015, #4682 ) ;
#4435=CARTESIAN_POINT ( 'NONE',  ( -15.29705854078139460, 55.48535772202409078, -3.843012250319258015E-15 ) ) ;
#4440=EDGE_CURVE ( 'NONE', #6322, #13011, #8461, .T. ) ;
#4444=EDGE_CURVE ( 'NONE', #8621, #5403, #10762, .T. ) ;
#4447=ORIENTED_EDGE ( 'NONE', *, *, #6628, .T. ) ;
#4450=EDGE_LOOP ( 'NONE', ( #6346, #8394, #10400, #11834 ) ) ;
#4451=CARTESIAN_POINT ( 'NONE',  ( 8.385254915620294014, 31.55439052270045508, 9.688596779957294507E-16 ) ) ;
#4453=CIRCLE ( 'NONE', #9626, 8.385254915620292238 ) ;
#4454=DIRECTION ( 'NONE',  ( 1.000000000000000000, 0.000000000000000000, 0.000000000000000000 ) ) ;
#4455=DIRECTION ( 'NONE',  ( -0.000000000000000000, -0.000000000000000000, -1.000000000000000000 ) ) ;
#4457=DIRECTION ( 'NONE',  ( -2.797435172181481150E-17, 1.000000000000000000, -1.765856845898762549E-18 ) ) ;
#4462=AXIS2_PLACEMENT_3D ( 'NONE', #9784, #13177, #5711 ) ;
#4464=AXIS2_PLACEMENT_3D ( 'NONE', #9369, #9440, #952 ) ;
#4465=AXIS2_PLACEMENT_3D ( 'NONE', #320, #3382, #9991 ) ;
#4468=DIRECTION ( 'NONE',  ( -1.000000000000000000, 0.000000000000000000, 0.000000000000000000 ) ) ;
#4470=CARTESIAN_POINT ( 'NONE',  ( -15.29705854078139637, 74.33491362204294717, -2.135879010051317068E-15 ) ) ;
#4472=DIRECTION ( 'NONE',  ( -1.000000000000000000, 0.000000000000000000, 0.000000000000000000 ) ) ;
#4474=CARTESIAN_POINT ( 'NONE',  ( -7.476762168534553332, -73.27151470233611974, -6.844715463267832867 ) ) ;
#4475=CARTESIAN_POINT ( 'NONE',  ( -2.517691654963332357E-15, 90.00000000000000000, -1.589271161308885878E-16 ) ) ;
#4476=CARTESIAN_POINT ( 'NONE',  ( -8.385254915620294014, 90.00000000000000000, -1.589271161308885878E-16 ) ) ;
#4477=CIRCLE ( 'NONE', #1807, 5.000000000000000000 ) ;
#4478=CARTESIAN_POINT ( 'NONE',  ( -15.29705854078140170, -29.33764382806072746, -3.749737291961210528E-15 ) ) ;
#4479=CARTESIAN_POINT ( 'NONE',  ( 12.99579180576516890, 26.38439787695498495, 0.000000000000000000 ) ) ;
#4481=ADVANCED_FACE ( 'NONE', ( #5819 ), #4972, .F. ) ;
#4482=AXIS2_PLACEMENT_3D ( 'NONE', #1600, #2723, #5884 ) ;
#4485=EDGE_LOOP ( 'NONE', ( #9194, #3013, #7660, #12086 ) ) ;
#4486=DIRECTION ( 'NONE',  ( -2.797435172181481150E-17, 1.000000000000000000, -1.765856845898762549E-18 ) ) ;
#4489=ORIENTED_EDGE ( 'NONE', *, *, #6260, .T. ) ;
#4490=CARTESIAN_POINT ( 'NONE',  ( 1.958204620527036497E-15, -70.00000000000000000, 1.236099792129133461E-16 ) ) ;
#4492=CARTESIAN_POINT ( 'NONE',  ( 12.99579180576516535, 35.80917582696438473, 3.183050967463142196E-15 ) ) ;
#4494=CARTESIAN_POINT ( 'NONE',  ( 12.99579180576516535, 7.534841976936129448, 1.578957136884995801E-15 ) ) ;
#4497=CARTESIAN_POINT ( 'NONE',  ( 1.111302931123402171, -163.8787878463619734, 2.940232648233732426 ) ) ;
#4498=CARTESIAN_POINT ( 'NONE',  ( -10.14773761995943069, -69.33333333333402493, 0.3621078539017010822 ) ) ;
#4506=ORIENTED_EDGE ( 'NONE', *, *, #5568, .F. ) ;
#4508=CARTESIAN_POINT ( 'NONE',  ( -15.29705854078140170, 90.00000000000000000, -1.589271161308885878E-16 ) ) ;
#4509=CARTESIAN_POINT ( 'NONE',  ( 10.69381717166375090, 25.55944687211528787, 21.38763434332751245 ) ) ;
#4511=DIRECTION ( 'NONE',  ( -2.797435172181481150E-17, 1.000000000000000000, -1.765856845898762549E-18 ) ) ;
#4513=CARTESIAN_POINT ( 'NONE',  ( 10.69381717166375800, -30.98922082794128485, 21.38763434332752666 ) ) ;
#4514=CARTESIAN_POINT ( 'NONE',  ( -8.385254915620297567, 90.00000000000000000, -1.589271161308885878E-16 ) ) ;
#4517=CARTESIAN_POINT ( 'NONE',  ( -0.6173387890061912131, -40.00941361824966691, 4.961742921553712549 ) ) ;
#4519=EDGE_LOOP ( 'NONE', ( #13835, #11111, #12104, #11102 ) ) ;
#4522=VERTEX_POINT ( 'NONE', #2596 ) ;
#4526=VECTOR ( 'NONE', #334, 1000.000000000000000 ) ;
#4528=FACE_OUTER_BOUND ( 'NONE', #12363, .T. ) ;
#4529=VERTEX_POINT ( 'NONE', #5742 ) ;
#4530=ORIENTED_EDGE ( 'NONE', *, *, #6935, .F. ) ;
#4531=ADVANCED_FACE ( 'NONE', ( #9117 ), #11377, .T. ) ;
#4533=CARTESIAN_POINT ( 'NONE',  ( 12.99553232110414136, 29.92431064457076673, 0.000000000000000000 ) ) ;
#4538=ORIENTED_EDGE ( 'NONE', *, *, #12547, .F. ) ;
#4539=EDGE_CURVE ( 'NONE', #149, #11311, #11071, .T. ) ;
#4540=CARTESIAN_POINT ( 'NONE',  ( 10.69381717166374735, 72.68333662216240043, 21.38763434332750890 ) ) ;
#4541=ADVANCED_FACE ( 'NONE', ( #13711 ), #12832, .T. ) ;
#4542=DIRECTION ( 'NONE',  ( -1.000000000000000000, 0.000000000000000000, 0.000000000000000000 ) ) ;
#4545=DIRECTION ( 'NONE',  ( -2.797435172181481150E-17, 1.000000000000000000, -1.765856845898762549E-18 ) ) ;
#4546=CARTESIAN_POINT ( 'NONE',  ( 4.330127018922190096, 91.82970358694004176, -2.500000000000000444 ) ) ;
#4547=CARTESIAN_POINT ( 'NONE',  ( -8.540654091808187687, -91.31629189966393767, 1.858473920087736930 ) ) ;
#4548=DIRECTION ( 'NONE',  ( -2.797435172181481150E-17, 1.000000000000000000, -1.765856845898762549E-18 ) ) ;
#4551=VERTEX_POINT ( 'NONE', #5177 ) ;
#4553=ORIENTED_EDGE ( 'NONE', *, *, #7477, .F. ) ;
#4555=CARTESIAN_POINT ( 'NONE',  ( 8.385254915620292238, 90.00000000000000000, 8.679704431140114636E-16 ) ) ;
#4557=CARTESIAN_POINT ( 'NONE',  ( 8.385254915620288685, -3.520109059331755219, 16.77050983124058448 ) ) ;
#4558=( NAMED_UNIT ( * ) SI_UNIT ( $, .STERADIAN. ) SOLID_ANGLE_UNIT ( ) );
#4559=CARTESIAN_POINT ( 'NONE',  ( -10.69381717166375800, 34.98422482212468054, 21.38763434332750535 ) ) ;
#4561=CARTESIAN_POINT ( 'NONE',  ( 8.385254915620292238, 90.00000000000000000, 8.679704431140114636E-16 ) ) ;
#4564=CARTESIAN_POINT ( 'NONE',  ( -8.385254915620297567, 90.00000000000000000, -1.589271161308885878E-16 ) ) ;
#4565=CARTESIAN_POINT ( 'NONE',  ( 8.385254915620288685, 53.02855864072483882, 9.355740606675293587E-16 ) ) ;
#4566=CARTESIAN_POINT ( 'NONE',  ( -12.99553232110414847, -17.19957910547634228, 25.99106464220827917 ) ) ;
#4568=CIRCLE ( 'NONE', #117, 2.000000000000003997 ) ;
#4569=ORIENTED_EDGE ( 'NONE', *, *, #2863, .T. ) ;
#4573=CARTESIAN_POINT ( 'NONE',  ( -10.00000000000000533, 92.00000000000000000, 2.500000000000000000 ) ) ;
#4574=DIRECTION ( 'NONE',  ( -2.797435172181481150E-17, 1.000000000000000000, -1.765856845898762549E-18 ) ) ;
#4576=AXIS2_PLACEMENT_3D ( 'NONE', #6416, #7460, #885 ) ;
#4577=ORIENTED_EDGE ( 'NONE', *, *, #8238, .T. ) ;
#4578=DIRECTION ( 'NONE',  ( -0.000000000000000000, -0.000000000000000000, -1.000000000000000000 ) ) ;
#4580=DIRECTION ( 'NONE',  ( 0.000000000000000000, 0.000000000000000000, 1.000000000000000000 ) ) ;
#4582=CARTESIAN_POINT ( 'NONE',  ( 15.29705854078139105, 27.21102387199583816, 3.746698755667522411E-15 ) ) ;
#4583=CARTESIAN_POINT ( 'NONE',  ( 35.45454545454547457, 140.4866414850956744, -2.500000000000000000 ) ) ;
#4584=VECTOR ( 'NONE', #4578, 1000.000000000000000 ) ;
#4585=CARTESIAN_POINT ( 'NONE',  ( -10.00000000000000711, 139.9999999999999716, -2.500000000000000000 ) ) ;
#4587=APPLICATION_CONTEXT ( 'automotive_design' ) ;
#4590=DIRECTION ( 'NONE',  ( -1.000000000000000000, 0.000000000000000000, 0.000000000000000000 ) ) ;
#4591=CARTESIAN_POINT ( 'NONE',  ( 10.69346802281034847, -6.949821576306441706, 0.000000000000000000 ) ) ;
#4594=CYLINDRICAL_SURFACE ( 'NONE', #2704, 50.00000000000001421 ) ;
#4596=CARTESIAN_POINT ( 'NONE',  ( -0.1852016367018560761, -70.00000000000000000, 1.488522876466114253 ) ) ;
#4599=CARTESIAN_POINT ( 'NONE',  ( 10.11144057928414242, -69.99977036137985920, -0.2534939170199681513 ) ) ;
#4610=CARTESIAN_POINT ( 'NONE',  ( 9.346811155104262525, -72.85217758658251341, 3.836677952648664292 ) ) ;
#4612=EDGE_LOOP ( 'NONE', ( #8102, #1205, #6834, #12067 ) ) ;
#4614=CARTESIAN_POINT ( 'NONE',  ( -8.385254915620290461, -24.99427717735608567, -16.77050983124058803 ) ) ;
#4621=CARTESIAN_POINT ( 'NONE',  ( 5.570495138619319060E-16, -19.91286587805129926, 3.516327053222078456E-17 ) ) ;
#4624=CARTESIAN_POINT ( 'NONE',  ( 3.521437233922025456, 90.23421079890158580, -3.553194557407191034 ) ) ;
#4626=ADVANCED_FACE ( 'NONE', ( #5107 ), #2866, .T. ) ;
#4630=ADVANCED_FACE ( 'NONE', ( #4119 ), #374, .T. ) ;
#4632=DIRECTION ( 'NONE',  ( -1.000000000000000000, -2.797435172181480534E-17, -0.000000000000000000 ) ) ;
#4633=VERTEX_POINT ( 'NONE', #9728 ) ;
#4634=CARTESIAN_POINT ( 'NONE',  ( 6.629834776934352192, -74.11811802551933681, 7.660853572563749658 ) ) ;
#4636=CARTESIAN_POINT ( 'NONE',  ( 10.69346802281034670, 59.02362407375952102, -21.38693604562068629 ) ) ;
#4639=CARTESIAN_POINT ( 'NONE',  ( -9.561354441693807661E-16, 34.17900274070598243, -6.035522597566817733E-17 ) ) ;
#4640=CARTESIAN_POINT ( 'NONE',  ( 9.849578953078907517, -91.60173160171747497, -1.758148290379567769 ) ) ;
#4644=DIRECTION ( 'NONE',  ( 1.000000000000000000, 0.000000000000000000, 0.000000000000000000 ) ) ;
#4645=ORIENTED_EDGE ( 'NONE', *, *, #6212, .T. ) ;
#4646=ORIENTED_EDGE ( 'NONE', *, *, #10643, .T. ) ;
#4647=DIRECTION ( 'NONE',  ( 2.797435172181480534E-17, -1.000000000000000000, 1.765856845898762164E-18 ) ) ;
#4652=CYLINDRICAL_SURFACE ( 'NONE', #6487, 24.99999999999998934 ) ;
#4655=ORIENTED_EDGE ( 'NONE', *, *, #6137, .F. ) ;
#4656=ORIENTED_EDGE ( 'NONE', *, *, #10866, .F. ) ;
#4658=VERTEX_POINT ( 'NONE', #2288 ) ;
#4661=CARTESIAN_POINT ( 'NONE',  ( 10.69381717166375267, 72.68333662216238622, 0.000000000000000000 ) ) ;
#4662=CARTESIAN_POINT ( 'NONE',  ( 15.29705854078138927, 36.63580182200523438, 1.806990092252540434E-15 ) ) ;
#4666=AXIS2_PLACEMENT_3D ( 'NONE', #4268, #8284, #4072 ) ;
#4667=DIRECTION ( 'NONE',  ( -1.000000000000000000, 0.000000000000000000, 0.000000000000000000 ) ) ;
#4668=CARTESIAN_POINT ( 'NONE',  ( 10.69346802281035202, -6.949821576306441706, -21.38693604562069339 ) ) ;
#4670=CARTESIAN_POINT ( 'NONE',  ( 4.330127018922190985, 92.00000000000000000, 2.500000000000000000 ) ) ;
#4671=VERTEX_POINT ( 'NONE', #7071 ) ;
#4675=FACE_OUTER_BOUND ( 'NONE', #1039, .T. ) ;
#4678=CARTESIAN_POINT ( 'NONE',  ( -49.99999999999999289, 120.0000000000000284, -0.5000000000000000000 ) ) ;
#4680=DIRECTION ( 'NONE',  ( 1.000000000000000000, 0.000000000000000000, 0.000000000000000000 ) ) ;
#4681=AXIS2_PLACEMENT_3D ( 'NONE', #13560, #10364, #3064 ) ;
#4682=DIRECTION ( 'NONE',  ( -1.000000000000000000, 0.000000000000000000, 0.000000000000000000 ) ) ;
#4683=AXIS2_PLACEMENT_3D ( 'NONE', #672, #13323, #9225 ) ;
#4687=ORIENTED_EDGE ( 'NONE', *, *, #2997, .T. ) ;
#4693=CARTESIAN_POINT ( 'NONE',  ( -0.2881385893809246812, -81.23289783331699709, -9.920954048540957970 ) ) ;
#4694=CARTESIAN_POINT ( 'NONE',  ( 8.385254915620292238, 59.82872437272870769, 2.053795118489800004E-15 ) ) ;
#4697=ORIENTED_EDGE ( 'NONE', *, *, #10470, .T. ) ;
#4700=EDGE_CURVE ( 'NONE', #849, #575, #2154, .T. ) ;
#4701=CARTESIAN_POINT ( 'NONE',  ( 15.29705854078139637, -27.45107625865536605, 3.746698755667523989E-15 ) ) ;
#4702=EDGE_CURVE ( 'NONE', #10679, #3210, #3204, .T. ) ;
#4705=CARTESIAN_POINT ( 'NONE',  ( 4.330127018922190985, 92.00000000000000000, 2.500000000000000000 ) ) ;
#4707=CARTESIAN_POINT ( 'NONE',  ( 8.385254915620285132, 34.17900274070598243, 16.77050983124058092 ) ) ;
#4713=CARTESIAN_POINT ( 'NONE',  ( -6.459897978785787309, -117.0909090909085393, -0.7661034210343102835 ) ) ;
#4715=DIRECTION ( 'NONE',  ( 2.797435172181480534E-17, -1.000000000000000000, 1.765856845898762164E-18 ) ) ;
#4717=CARTESIAN_POINT ( 'NONE',  ( 8.385254915620292238, 90.00000000000000000, 8.679704431140114636E-16 ) ) ;
#4721=DIRECTION ( 'NONE',  ( -1.000000000000000000, 0.000000000000000000, 0.000000000000000000 ) ) ;
#4723=CARTESIAN_POINT ( 'NONE',  ( 1.149505143677158392, -121.5517071194484089, 4.892824251472469577 ) ) ;
#4724=DIRECTION ( 'NONE',  ( -1.000000000000000000, 0.000000000000000000, 0.000000000000000000 ) ) ;
#4729=CARTESIAN_POINT ( 'NONE',  ( -15.29705854078139460, -18.02629830864596627, 3.183186227453577089E-17 ) ) ;
#4730=EDGE_CURVE ( 'NONE', #3489, #4551, #11345, .T. ) ;
#4731=CYLINDRICAL_SURFACE ( 'NONE', #11434, 15.29705854078139460 ) ;
#4734=VERTEX_POINT ( 'NONE', #10831 ) ;
#4735=ADVANCED_FACE ( 'NONE', ( #204 ), #5992, .T. ) ;
#4737=CARTESIAN_POINT ( 'NONE',  ( -25.00000000000000355, 120.0000000000000284, -0.5000000000000000000 ) ) ;
#4741=EDGE_CURVE ( 'NONE', #3627, #3001, #10923, .T. ) ;
#4746=DIRECTION ( 'NONE',  ( -1.000000000000000000, 0.000000000000000000, 0.000000000000000000 ) ) ;
#4747=B_SPLINE_CURVE_WITH_KNOTS ( 'NONE', 3,
 ( #657, #3657, #2822, #1629 ),
 .UNSPECIFIED., .F., .F.,
 ( 4, 4 ),
 ( 0.000000000000000000, 1.000000000000000000 ),
 .UNSPECIFIED. ) ;
#4748=CARTESIAN_POINT ( 'NONE',  ( -2.517691654963332357E-15, 90.00000000000000000, -1.589271161308885878E-16 ) ) ;
#4749=ORIENTED_EDGE ( 'NONE', *, *, #4440, .T. ) ;
#4754=DIRECTION ( 'NONE',  ( -1.000000000000000000, 0.000000000000000000, 0.000000000000000000 ) ) ;
#4758=CARTESIAN_POINT ( 'NONE',  ( -11.95302590259205111, -161.0909090909570409, -5.173310689868307222 ) ) ;
#4759=EDGE_CURVE ( 'NONE', #7271, #717, #3739, .T. ) ;
#4760=CARTESIAN_POINT ( 'NONE',  ( -15.29705854078139282, 8.361467971976955127, 30.59411708156277498 ) ) ;
#4762=CARTESIAN_POINT ( 'NONE',  ( 8.385254915620295790, -34.41905512736551032, 16.77050983124059513 ) ) ;
#4764=FACE_OUTER_BOUND ( 'NONE', #12154, .T. ) ;
#4767=EDGE_LOOP ( 'NONE', ( #3587, #10789, #8586, #10566 ) ) ;
#4770=CARTESIAN_POINT ( 'NONE',  ( 10.69346802281034847, -35.22415542633469698, 1.384126719801006158E-15 ) ) ;
#4771=CARTESIAN_POINT ( 'NONE',  ( -15.29705854078139105, 76.22148119144830503, -2.142541826566686405E-15 ) ) ;
#4772=CARTESIAN_POINT ( 'NONE',  ( -36.36363636363635976, 142.2680885707561629, 2.500000000000000000 ) ) ;
#4774=CARTESIAN_POINT ( 'NONE',  ( 3.581682357367548697, -100.7588871204822283, 6.662357539611612367 ) ) ;
#4775=( BOUNDED_SURFACE ( )  B_SPLINE_SURFACE ( 3, 3, ( 
 ( #7674, #11954, #7404, #6495 ),
 ( #5431, #3328, #1240, #6630 ),
 ( #8876, #8955, #2416, #11194 ),
 ( #3682, #7967, #483, #1369 ) ),
 .UNSPECIFIED., .F., .F., .T. ) 
 B_SPLINE_SURFACE_WITH_KNOTS ( ( 4, 4 ),
 ( 4, 4 ),
 ( 0.000000000000000000, 1.000000000000000000 ),
 ( 0.000000000000000000, 1.000000000000000000 ),
 .UNSPECIFIED. ) 
 GEOMETRIC_REPRESENTATION_ITEM ( )  RATIONAL_B_SPLINE_SURFACE ( (
 ( 1.000000000000000000, 0.3333333333333334259, 0.3333333333333334259, 1.000000000000000000),
 ( 1.000000000000000000, 0.3333333333333334259, 0.3333333333333334259, 1.000000000000000000),
 ( 1.000000000000000000, 0.3333333333333334259, 0.3333333333333334259, 1.000000000000000000),
 ( 1.000000000000000000, 0.3333333333333334259, 0.3333333333333334259, 1.000000000000000000) ) ) 
 REPRESENTATION_ITEM ( '' )  SURFACE ( )  );
#4779=ORIENTED_EDGE ( 'NONE', *, *, #13832, .F. ) ;
#4783=CARTESIAN_POINT ( 'NONE',  ( 1.010510313258186077, -79.21212121212082025, 9.990963482113931704 ) ) ;
#4785=CARTESIAN_POINT ( 'NONE',  ( 4.769557440008696858, 90.26587002877201371, 1.504714191168455617 ) ) ;
#4787=CARTESIAN_POINT ( 'NONE',  ( -3.692320488640446374, -128.7272727272685131, 2.755591346289536059 ) ) ;
#4789=CARTESIAN_POINT ( 'NONE',  ( 8.385254915620295790, -15.56949922734665570, 1.052073721316228892E-15 ) ) ;
#4790=CARTESIAN_POINT ( 'NONE',  ( -4.855892414095311693, -117.0909090909095340, -4.610765637404268702 ) ) ;
#4793=DIRECTION ( 'NONE',  ( 1.000000000000000000, 0.000000000000000000, 0.000000000000000000 ) ) ;
#4797=AXIS2_PLACEMENT_3D ( 'NONE', #8840, #12070, #1411 ) ;
#4798=CARTESIAN_POINT ( 'NONE',  ( 0.1617766054438460888, -158.9591451343941344, 1.491567609517463255 ) ) ;
#4802=CIRCLE ( 'NONE', #6575, 15.29705854078138927 ) ;
#4804=FACE_OUTER_BOUND ( 'NONE', #10031, .T. ) ;
#4807=ORIENTED_EDGE ( 'NONE', *, *, #10458, .T. ) ;
#4808=CARTESIAN_POINT ( 'NONE',  ( -0.7078152277712073115, -145.1309382821781924, 2.289704460722573387 ) ) ;
#4809=CARTESIAN_POINT ( 'NONE',  ( 4.974937185533097050, 90.00000000000000000, -0.5000000000000000000 ) ) ;
#4811=AXIS2_PLACEMENT_3D ( 'NONE', #7822, #13039, #4262 ) ;
#4817=EDGE_CURVE ( 'NONE', #11439, #2969, #6873, .T. ) ;
#4819=DIRECTION ( 'NONE',  ( -1.000000000000000000, 0.000000000000000000, 0.000000000000000000 ) ) ;
#4820=CARTESIAN_POINT ( 'NONE',  ( 1.275238607054845374, -147.1038961039289177, -4.986937111405163492 ) ) ;
#4824=CIRCLE ( 'NONE', #7493, 8.385254915620292238 ) ;
#4825=ORIENTED_EDGE ( 'NONE', *, *, #26, .T. ) ;
#4826=CARTESIAN_POINT ( 'NONE',  ( 0.5000000000000032196, -40.00941361824966691, -2.499999999999982236 ) ) ;
#4827=CARTESIAN_POINT ( 'NONE',  ( 15.29705854078138572, 57.37192529142945574, 1.773704474924340342E-15 ) ) ;
#4829=CARTESIAN_POINT ( 'NONE',  ( 15.29705854078139105, 36.63580182200523438, 1.806990092252540434E-15 ) ) ;
#4830=CARTESIAN_POINT ( 'NONE',  ( 10.69381717166375623, 6.709890972096427042, 2.619229793989003951E-15 ) ) ;
#4842=CIRCLE ( 'NONE', #8414, 5.000000000000000000 ) ;
#4846=CARTESIAN_POINT ( 'NONE',  ( 6.636652343254445086, -87.27833817527823612, -6.409095190688999466 ) ) ;
#4847=CARTESIAN_POINT ( 'NONE',  ( 10.69346802281035025, 49.59884612375012836, -21.38693604562069339 ) ) ;
#4849=VERTEX_POINT ( 'NONE', #2579 ) ;
#4850=EDGE_LOOP ( 'NONE', ( #11065, #5434, #4950, #13553 ) ) ;
#4853=LINE ( 'NONE', #13442, #3216 ) ;
#4854=CARTESIAN_POINT ( 'NONE',  ( 7.783279735887545847, -74.45454545454821016, 6.359494517302611172 ) ) ;
#4856=CARTESIAN_POINT ( 'NONE',  ( 1.381416096079823630, -78.35919756719752627, 10.01283213701209540 ) ) ;
#4857=DIRECTION ( 'NONE',  ( -2.797435172181481150E-17, 1.000000000000000000, -1.765856845898762549E-18 ) ) ;
#4858=CARTESIAN_POINT ( 'NONE',  ( -7.670607444602973501, -76.12121212000219828, -4.175606131682665811 ) ) ;
#4861=ORIENTED_EDGE ( 'NONE', *, *, #10805, .T. ) ;
#4862=ORIENTED_EDGE ( 'NONE', *, *, #2049, .F. ) ;
#4865=ORIENTED_EDGE ( 'NONE', *, *, #27, .F. ) ;
#4866=CARTESIAN_POINT ( 'NONE',  ( -2.357122643816039087, -126.8853818545090348, 3.740305772406630869 ) ) ;
#4869=ORIENTED_EDGE ( 'NONE', *, *, #8928, .T. ) ;
#4871=CARTESIAN_POINT ( 'NONE',  ( -0.2492428495092258167, -158.6992603437087723, -1.476418605036174725 ) ) ;
#4872=ADVANCED_FACE ( 'NONE', ( #11136 ), #12012, .T. ) ;
#4879=CARTESIAN_POINT ( 'NONE',  ( 2.179449471770333435, 90.00000000000000000, 4.500000000000000888 ) ) ;
#4881=CARTESIAN_POINT ( 'NONE',  ( 4.364119526983701647, -68.90909090873145715, 1.457038019206917223 ) ) ;
#4887=EDGE_CURVE ( 'NONE', #2529, #5403, #8188, .T. ) ;
#4888=CARTESIAN_POINT ( 'NONE',  ( -3.682460330434897067, -161.0909090908357371, -2.758257593116285822 ) ) ;
#4891=CARTESIAN_POINT ( 'NONE',  ( -12.99553232110414491, 20.49953269456136695, 25.99106464220827917 ) ) ;
#4892=UNCERTAINTY_MEASURE_WITH_UNIT (LENGTH_MEASURE( 1.000000000000000082E-05 ), #2535, 'distance_accuracy_value', 'NONE');
#4893=CARTESIAN_POINT ( 'NONE',  ( 3.989522629621962579, -78.56682793483436456, 9.305603774495006419 ) ) ;
#4896=ORIENTED_EDGE ( 'NONE', *, *, #2226, .T. ) ;
#4897=AXIS2_PLACEMENT_3D ( 'NONE', #3351, #218, #4472 ) ;
#4898=CARTESIAN_POINT ( 'NONE',  ( -1.868713978126510744, -80.62942566232119646, 9.873777329404955339 ) ) ;
#4899=EDGE_CURVE ( 'NONE', #5287, #10825, #1052, .T. ) ;
#4902=CARTESIAN_POINT ( 'NONE',  ( -8.385254915620295790, -6.144721277337255927, 1.085069813372578838E-17 ) ) ;
#4903=EDGE_CURVE ( 'NONE', #2222, #13867, #13629, .T. ) ;
#4907=CARTESIAN_POINT ( 'NONE',  ( -5.609076778736961089, -113.1406196337631229, 2.279675803883993268 ) ) ;
#4908=CIRCLE ( 'NONE', #4683, 2.000000000000000000 ) ;
#4909=CARTESIAN_POINT ( 'NONE',  ( 10.69381717166375800, 16.13466892210585257, -21.38763434332750535 ) ) ;
#4914=CARTESIAN_POINT ( 'NONE',  ( -35.45454545454546036, 140.4866414850956744, -2.500000000000000000 ) ) ;
#4917=LINE ( 'NONE', #10246, #8515 ) ;
#4922=CARTESIAN_POINT ( 'NONE',  ( 2.966263562845762980, -142.5800865801409145, 0.5601050917291978681 ) ) ;
#4923=EDGE_CURVE ( 'NONE', #3901, #8317, #164, .T. ) ;
#4928=ORIENTED_EDGE ( 'NONE', *, *, #6323, .T. ) ;
#4930=EDGE_LOOP ( 'NONE', ( #11350, #11586, #73, #10437 ) ) ;
#4931=ORIENTED_EDGE ( 'NONE', *, *, #9279, .F. ) ;
#4934=CARTESIAN_POINT ( 'NONE',  ( 6.207397642386911052, -111.4641340365256355, -0.7891162744033484167 ) ) ;
#4937=CYLINDRICAL_SURFACE ( 'NONE', #248, 79.99999999999997158 ) ;
#4940=CARTESIAN_POINT ( 'NONE',  ( 0.7922720876982874971, -124.2424753664742667, -4.680861543279757342 ) ) ;
#4941=AXIS2_PLACEMENT_3D ( 'NONE', #9579, #12825, #831 ) ;
#4942=AXIS2_PLACEMENT_3D ( 'NONE', #9605, #11905, #8680 ) ;
#4943=FACE_OUTER_BOUND ( 'NONE', #3454, .T. ) ;
#4948=CARTESIAN_POINT ( 'NONE',  ( -15.29705854078139637, 64.91013567203349055, -2.102593392723117370E-15 ) ) ;
#4950=ORIENTED_EDGE ( 'NONE', *, *, #3680, .T. ) ;
#4952=CARTESIAN_POINT ( 'NONE',  ( 10.69346802281034492, 40.17406817374066463, 0.000000000000000000 ) ) ;
#4954=CARTESIAN_POINT ( 'NONE',  ( -0.7140975576127730484, -124.8181818181825093, 13.04184819563903197 ) ) ;
#4955=ORIENTED_EDGE ( 'NONE', *, *, #4419, .T. ) ;
#4956=EDGE_LOOP ( 'NONE', ( #9738, #1256, #5576, #3362 ) ) ;
#4960=CARTESIAN_POINT ( 'NONE',  ( -2.920448137081767204, -118.2727272727305063, -4.227847206581263784 ) ) ;
#4961=CIRCLE ( 'NONE', #6730, 2.000000000000000000 ) ;
#4963=CARTESIAN_POINT ( 'NONE',  ( 15.29705854078138394, 8.361467971976955127, 30.59411708156277854 ) ) ;
#4966=ORIENTED_EDGE ( 'NONE', *, *, #1994, .F. ) ;
#4967=ADVANCED_FACE ( 'NONE', ( #13558 ), #9783, .T. ) ;
#4969=CIRCLE ( 'NONE', #13280, 2.000000000000003997 ) ;
#4970=EDGE_LOOP ( 'NONE', ( #5649, #8529, #11734, #5482 ) ) ;
#4971=DIRECTION ( 'NONE',  ( -1.000000000000000000, -2.835060530349834805E-17, 0.000000000000000000 ) ) ;
#4972=CYLINDRICAL_SURFACE ( 'NONE', #10490, 14.99999999999998934 ) ;
#4974=AXIS2_PLACEMENT_3D ( 'NONE', #7827, #4026, #9367 ) ;
#4975=CARTESIAN_POINT ( 'NONE',  ( 41.99999999999999289, 120.0000000000000284, 0.5000000000000000000 ) ) ;
#4976=CARTESIAN_POINT ( 'NONE',  ( -4.163221732489563287, -120.7404873314440295, -2.994388017321735429 ) ) ;
#4978=ADVANCED_FACE ( 'NONE', ( #3909 ), #13502, .T. ) ;
#4979=ORIENTED_EDGE ( 'NONE', *, *, #1217, .T. ) ;
#4981=LINE ( 'NONE', #3929, #8303 ) ;
#4982=ADVANCED_FACE ( 'NONE', ( #9649 ), #5298, .T. ) ;
#4984=ORIENTED_EDGE ( 'NONE', *, *, #2327, .F. ) ;
#4985=CARTESIAN_POINT ( 'NONE',  ( -4.330127018922195425, 92.00000000000000000, -2.500000000000000000 ) ) ;
#4986=CARTESIAN_POINT ( 'NONE',  ( 9.977514653935656952, -69.33333333333050064, 0.8249805266091517764 ) ) ;
#4988=CARTESIAN_POINT ( 'NONE',  ( 15.29705854078138749, 10.24803554138234496, 1.856918518244839783E-15 ) ) ;
#4990=CARTESIAN_POINT ( 'NONE',  ( 0.4173931308547985108, -102.5454545454719266, -7.668730708680674191 ) ) ;
#4995=DIRECTION ( 'NONE',  ( 0.000000000000000000, 0.000000000000000000, 1.000000000000000000 ) ) ;
#4998=VERTEX_POINT ( 'NONE', #1296 ) ;
#4999=ORIENTED_EDGE ( 'NONE', *, *, #11919, .T. ) ;
#5000=ORIENTED_EDGE ( 'NONE', *, *, #4887, .F. ) ;
#5001=CARTESIAN_POINT ( 'NONE',  ( 5.055407487860802185, -107.2968172642280109, -4.489258388536537581 ) ) ;
#5002=AXIS2_PLACEMENT_3D ( 'NONE', #8629, #1408, #3297 ) ;
#5004=FACE_OUTER_BOUND ( 'NONE', #13268, .T. ) ;
#5006=DIRECTION ( 'NONE',  ( -2.797435172181481150E-17, 1.000000000000000000, -1.765856845898762549E-18 ) ) ;
#5008=CARTESIAN_POINT ( 'NONE',  ( 1.008311300638476515, -141.1586168970593178, 2.610279145673827461 ) ) ;
#5009=CARTESIAN_POINT ( 'NONE',  ( 0.6121604144011097981, -166.5454543771828924, 9.081467142972524442 ) ) ;
#5014=CARTESIAN_POINT ( 'NONE',  ( 8.385254915620295790, 31.55439052270045508, 2.053795118489801188E-15 ) ) ;
#5015=STYLED_ITEM ( 'NONE', ( #9982 ), #12476 ) ;
#5018=ORIENTED_EDGE ( 'NONE', *, *, #13162, .T. ) ;
#5019=CARTESIAN_POINT ( 'NONE',  ( -4.154595973944846143, -169.0000000000000853, 0.9946518452610447758 ) ) ;
#5020=ADVANCED_FACE ( 'NONE', ( #6491 ), #5741, .T. ) ;
#5023=AXIS2_PLACEMENT_3D ( 'NONE', #1517, #10648, #10896 ) ;
#5028=DIRECTION ( 'NONE',  ( 0.000000000000000000, 0.000000000000000000, 1.000000000000000000 ) ) ;
#5029=CARTESIAN_POINT ( 'NONE',  ( -25.00000000000000355, 120.0000000000000284, -0.5000000000000000000 ) ) ;
#5032=DIRECTION ( 'NONE',  ( 1.000000000000000000, -0.000000000000000000, 0.000000000000000000 ) ) ;
#5033=AXIS2_PLACEMENT_3D ( 'NONE', #7528, #52, #11609 ) ;
#5034=ORIENTED_EDGE ( 'NONE', *, *, #11404, .F. ) ;
#5035=VECTOR ( 'NONE', #757, 1000.000000000000000 ) ;
#5038=CARTESIAN_POINT ( 'NONE',  ( -12.99579180576516535, -20.73949187309215247, -25.99158361153034136 ) ) ;
#5041=ADVANCED_FACE ( 'NONE', ( #8523 ), #10426, .T. ) ;
#5043=VECTOR ( 'NONE', #4370, 1000.000000000000000 ) ;
#5044=CARTESIAN_POINT ( 'NONE',  ( 8.385254915620290461, 62.45333659073423860, 9.189312520034297072E-16 ) ) ;
#5046=CARTESIAN_POINT ( 'NONE',  ( 2.621224576962791986, -142.3792347905090594, 0.5672744485101375300 ) ) ;
#5048=DIRECTION ( 'NONE',  ( 2.797435172181480534E-17, -1.000000000000000000, 1.765856845898762164E-18 ) ) ;
#5051=CARTESIAN_POINT ( 'NONE',  ( 15.29705854078138927, -8.601520358636511432, 30.59411708156278564 ) ) ;
#5056=ORIENTED_EDGE ( 'NONE', *, *, #4289, .T. ) ;
#5057=CARTESIAN_POINT ( 'NONE',  ( 9.314636722532569024, -70.78787878787778709, 4.145366960882150842 ) ) ;
#5061=CARTESIAN_POINT ( 'NONE',  ( -7.181435285655783041, -97.41991341991587205, -5.065585088375700096 ) ) ;
#5063=AXIS2_PLACEMENT_3D ( 'NONE', #12746, #7401, #13508 ) ;
#5065=CARTESIAN_POINT ( 'NONE',  ( -2.179449471770338320, 90.00000000000000000, 4.500000000000000888 ) ) ;
#5066=CARTESIAN_POINT ( 'NONE',  ( -1.778232137369847088, -131.6676658674560940, 3.416367881604213785 ) ) ;
#5069=AXIS2_PLACEMENT_3D ( 'NONE', #12540, #7056, #9163 ) ;
#5072=ORIENTED_EDGE ( 'NONE', *, *, #13852, .F. ) ;
#5075=CARTESIAN_POINT ( 'NONE',  ( 0.4950592182222878224, -80.00113774393089727, 9.987843023254374231 ) ) ;
#5077=CARTESIAN_POINT ( 'NONE',  ( 8.218400508506594093, -92.47990103503111925, 2.510678252300570623 ) ) ;
#5080=CARTESIAN_POINT ( 'NONE',  ( 0.7584178690488649899, -80.00107432488880477, -10.05132151820344966 ) ) ;
#5081=DIRECTION ( 'NONE',  ( 0.000000000000000000, 0.000000000000000000, 1.000000000000000000 ) ) ;
#5082=CARTESIAN_POINT ( 'NONE',  ( -10.69346802281034847, 2.474956373702985157, -2.628033278317404684E-15 ) ) ;
#5084=EDGE_CURVE ( 'NONE', #1705, #9083, #12171, .T. ) ;
#5085=CARTESIAN_POINT ( 'NONE',  ( 10.69346802281034137, 30.74929022373127196, 21.38693604562069339 ) ) ;
#5091=VERTEX_POINT ( 'NONE', #477 ) ;
#5092=CARTESIAN_POINT ( 'NONE',  ( -4.804172150869138846, 90.20479154739604155, -1.391179344134541473 ) ) ;
#5094=CARTESIAN_POINT ( 'NONE',  ( 7.670607446487990977, -76.12121213288367017, 4.175606128970697384 ) ) ;
#5096=CARTESIAN_POINT ( 'NONE',  ( 57.42269783589186005, -167.3636363757462391, -5.376878111557598316 ) ) ;
#5100=DIRECTION ( 'NONE',  ( -1.000000000000000000, 0.000000000000000000, 0.000000000000000000 ) ) ;
#5101=CARTESIAN_POINT ( 'NONE',  ( -4.545390705139096710, 90.76307318580400363, 2.092381513276357463 ) ) ;
#5103=CARTESIAN_POINT ( 'NONE',  ( -8.724264547992721219, -88.38328649526096115, 2.552360124988750645 ) ) ;
#5104=ORIENTED_EDGE ( 'NONE', *, *, #4923, .T. ) ;
#5105=CARTESIAN_POINT ( 'NONE',  ( 12.99579180576516890, -11.31471392308272605, 1.630544471709826084E-15 ) ) ;
#5107=FACE_OUTER_BOUND ( 'NONE', #2816, .T. ) ;
#5108=CARTESIAN_POINT ( 'NONE',  ( -10.69381717166375090, -2.714886977913000710, -21.38763434332751245 ) ) ;
#5109=TOROIDAL_SURFACE ( 'NONE', #1527, 16.99999999999998934, 2.000000000000000000 ) ;
#5113=FACE_OUTER_BOUND ( 'NONE', #2952, .T. ) ;
#5117=CARTESIAN_POINT ( 'NONE',  ( 14.13596196814457606, -39.17949320881311337, 1.792870180259218362E-15 ) ) ;
#5120=CIRCLE ( 'NONE', #11831, 15.29705854078139460 ) ;
#5121=CARTESIAN_POINT ( 'NONE',  ( 8.385254915620285132, 43.60378069071538221, 16.77050983124058092 ) ) ;
#5123=CARTESIAN_POINT ( 'NONE',  ( 12.99553232110414136, 20.49953269456136695, 0.000000000000000000 ) ) ;
#5125=CARTESIAN_POINT ( 'NONE',  ( 1.857895717451711892, -124.7597759017244528, 4.290688988966868678 ) ) ;
#5129=CIRCLE ( 'NONE', #886, 8.385254915620295790 ) ;
#5133=EDGE_CURVE ( 'NONE', #10906, #1805, #2732, .T. ) ;
#5135=CARTESIAN_POINT ( 'NONE',  ( 8.385254915620290461, 40.97916847270985841, 16.77050983124059158 ) ) ;
#5137=CARTESIAN_POINT ( 'NONE',  ( 12.99553232110413781, 39.34908859458022334, 1.535118538324121067E-15 ) ) ;
#5138=CARTESIAN_POINT ( 'NONE',  ( 7.900400410507671722, -86.42170959821115162, -4.992527905362919682 ) ) ;
#5140=CARTESIAN_POINT ( 'NONE',  ( -1.824130267666668859, -166.5454545046794408, 2.249022964271035985 ) ) ;
#5141=CYLINDRICAL_SURFACE ( 'NONE', #12084, 8.385254915620292238 ) ;
#5145=CARTESIAN_POINT ( 'NONE',  ( -15.29705854078139282, 29.09759144140119957, 30.59411708156277498 ) ) ;
#5146=CARTESIAN_POINT ( 'NONE',  ( -15.29705854078138749, 38.52236939141059935, -6.802498971006334016E-17 ) ) ;
#5150=AXIS2_PLACEMENT_3D ( 'NONE', #4003, #11368, #13586 ) ;
#5151=CARTESIAN_POINT ( 'NONE',  ( -12.87330105402729785, -111.7272727272713553, 6.772701765862009893 ) ) ;
#5154=VECTOR ( 'NONE', #8915, 1000.000000000000000 ) ;
#5156=ADVANCED_FACE ( 'NONE', ( #2489 ), #3752, .F. ) ;
#5157=EDGE_LOOP ( 'NONE', ( #1442, #4179, #4245, #11293 ) ) ;
#5159=EDGE_CURVE ( 'NONE', #10377, #10478, #4197, .T. ) ;
#5162=CARTESIAN_POINT ( 'NONE',  ( -17.09331748273503848, -62.63636360940330405, -11.08568378743039595 ) ) ;
#5169=EDGE_LOOP ( 'NONE', ( #3760, #1938, #12185, #12270 ) ) ;
#5173=AXIS2_PLACEMENT_3D ( 'NONE', #282, #506, #6793 ) ;
#5174=ORIENTED_EDGE ( 'NONE', *, *, #9297, .T. ) ;
#5177=CARTESIAN_POINT ( 'NONE',  ( 48.00000000000000000, 120.0000000000000284, -2.500000000000000000 ) ) ;
#5178=CARTESIAN_POINT ( 'NONE',  ( 0.000000000000000000, 71.01020514433645303, 0.5000000000000000000 ) ) ;
#5180=TOROIDAL_SURFACE ( 'NONE', #6987, 48.00000000000001421, 2.000000000000000000 ) ;
#5181=VERTEX_POINT ( 'NONE', #13256 ) ;
#5182=DIRECTION ( 'NONE',  ( -2.797435172181481150E-17, 1.000000000000000000, -1.765856845898762549E-18 ) ) ;
#5183=VERTEX_POINT ( 'NONE', #7738 ) ;
#5184=ORIENTED_EDGE ( 'NONE', *, *, #4903, .T. ) ;
#5186=CARTESIAN_POINT ( 'NONE',  ( -12.99553232110413425, 77.04820039461787928, -25.99106464220827561 ) ) ;
#5189=( BOUNDED_SURFACE ( )  B_SPLINE_SURFACE ( 3, 3, ( 
 ( #13722, #4132, #10585, #2882 ),
 ( #5117, #7155, #1832, #4193 ),
 ( #2957, #8478, #8350, #11573 ),
 ( #6116, #9406, #10389, #9340 ) ),
 .UNSPECIFIED., .F., .F., .T. ) 
 B_SPLINE_SURFACE_WITH_KNOTS ( ( 4, 4 ),
 ( 4, 4 ),
 ( 0.000000000000000000, 1.000000000000000000 ),
 ( 0.000000000000000000, 1.000000000000000000 ),
 .UNSPECIFIED. ) 
 GEOMETRIC_REPRESENTATION_ITEM ( )  RATIONAL_B_SPLINE_SURFACE ( (
 ( 1.000000000000000000, 0.3333333333333334259, 0.3333333333333334259, 1.000000000000000000),
 ( 1.000000000000000000, 0.3333333333333334259, 0.3333333333333334259, 1.000000000000000000),
 ( 1.000000000000000000, 0.3333333333333334259, 0.3333333333333334259, 1.000000000000000000),
 ( 1.000000000000000000, 0.3333333333333334259, 0.3333333333333334259, 1.000000000000000000) ) ) 
 REPRESENTATION_ITEM ( '' )  SURFACE ( )  );
#5193=CARTESIAN_POINT ( 'NONE',  ( -8.355259927329338865, -76.12121211926928765, -3.018973158331568651 ) ) ;
#5195=CARTESIAN_POINT ( 'NONE',  ( -8.385254915620292238, 69.25350232273815720, -16.77050983124058803 ) ) ;
#5196=CARTESIAN_POINT ( 'NONE',  ( 2.559300467072437968, -107.2281355222008159, -6.269538958562518083 ) ) ;
#5201=DIRECTION ( 'NONE',  ( -2.797435172181481150E-17, 1.000000000000000000, -1.765856845898762549E-18 ) ) ;
#5205=CARTESIAN_POINT ( 'NONE',  ( -5.939735700749026570, -113.5442540614846365, -1.042476841765012985 ) ) ;
#5207=CARTESIAN_POINT ( 'NONE',  ( -8.385254915620288685, 62.45333659073424570, -16.77050983124058092 ) ) ;
#5210=DIRECTION ( 'NONE',  ( -1.000000000000000000, 0.000000000000000000, 0.000000000000000000 ) ) ;
#5212=DIRECTION ( 'NONE',  ( -0.5999999999999989786, 0.8000000000000008216, 0.000000000000000000 ) ) ;
#5213=DIRECTION ( 'NONE',  ( 1.000000000000000000, 0.000000000000000000, 0.000000000000000000 ) ) ;
#5216=CARTESIAN_POINT ( 'NONE',  ( -2.503528417663017258, -105.1818181818192812, 12.81920766435409931 ) ) ;
#5218=CARTESIAN_POINT ( 'NONE',  ( -8.385254915620294014, 90.00000000000000000, -1.589271161308885878E-16 ) ) ;
#5219=ORIENTED_EDGE ( 'NONE', *, *, #12536, .F. ) ;
#5220=DIRECTION ( 'NONE',  ( -2.797435172181481150E-17, 1.000000000000000000, -1.765856845898762549E-18 ) ) ;
#5221=DIRECTION ( 'NONE',  ( -0.000000000000000000, -0.000000000000000000, -1.000000000000000000 ) ) ;
#5223=VECTOR ( 'NONE', #12290, 1000.000000000000114 ) ;
#5224=CARTESIAN_POINT ( 'NONE',  ( -2.078065351797288685, -164.3636363689741984, 0.8722068071970994207 ) ) ;
#5226=DIRECTION ( 'NONE',  ( 0.000000000000000000, 0.000000000000000000, 1.000000000000000000 ) ) ;
#5227=CARTESIAN_POINT ( 'NONE',  ( -15.29705854078139460, 47.94714734142005597, 30.59411708156277498 ) ) ;
#5229=EDGE_CURVE ( 'NONE', #8317, #5237, #4274, .T. ) ;
#5230=DIRECTION ( 'NONE',  ( 0.1234677578012386701, 0.000000000000000000, -0.9923485843107424653 ) ) ;
#5237=VERTEX_POINT ( 'NONE', #2777 ) ;
#5238=FACE_OUTER_BOUND ( 'NONE', #6965, .T. ) ;
#5241=CARTESIAN_POINT ( 'NONE',  ( 15.29705854078139282, 29.09759144140119957, -30.59411708156276788 ) ) ;
#5243=CARTESIAN_POINT ( 'NONE',  ( -5.799822669222908011, -77.11029879918604024, -8.314269053643187135 ) ) ;
#5244=CARTESIAN_POINT ( 'NONE',  ( 2.879696806288778888, -140.3684069432085266, -0.06694681502240752702 ) ) ;
#5246=ORIENTED_EDGE ( 'NONE', *, *, #1914, .T. ) ;
#5248=ORIENTED_EDGE ( 'NONE', *, *, #12552, .F. ) ;
#5249=LINE ( 'NONE', #8474, #5371 ) ;
#5251=DIRECTION ( 'NONE',  ( -2.797435172181481150E-17, 1.000000000000000000, -1.765856845898762549E-18 ) ) ;
#5253=CARTESIAN_POINT ( 'NONE',  ( -10.69346802281034670, 77.87317997377837742, -21.38693604562070050 ) ) ;
#5256=DIRECTION ( 'NONE',  ( -2.797435172181481150E-17, 1.000000000000000000, -1.765856845898762549E-18 ) ) ;
#5260=PLANE ( 'NONE',  #8137 ) ;
#5261=CARTESIAN_POINT ( 'NONE',  ( 4.723947684841503403, -119.5046656414372990, 2.345268719995682538 ) ) ;
#5266=ORIENTED_EDGE ( 'NONE', *, *, #7684, .T. ) ;
#5267=AXIS2_PLACEMENT_3D ( 'NONE', #12659, #941, #10466 ) ;
#5269=CARTESIAN_POINT ( 'NONE',  ( 1.204398987562338208, -146.6404311885195568, -1.908543418242987677 ) ) ;
#5271=LINE ( 'NONE', #9423, #11188 ) ;
#5272=ORIENTED_EDGE ( 'NONE', *, *, #7784, .T. ) ;
#5273=VECTOR ( 'NONE', #1712, 1000.000000000000000 ) ;
#5274=FACE_OUTER_BOUND ( 'NONE', #5169, .T. ) ;
#5275=CARTESIAN_POINT ( 'NONE',  ( 7.633069938044322100, -93.52166883861728763, 3.640362836796851465 ) ) ;
#5279=CARTESIAN_POINT ( 'NONE',  ( -15.29705854078139105, 19.67281349139177138, -3.783103832178228351E-15 ) ) ;
#5281=CARTESIAN_POINT ( 'NONE',  ( -9.536547895815854048, -71.90909090909266865, -3.228601540706718787 ) ) ;
#5283=CARTESIAN_POINT ( 'NONE',  ( 12.99579180576516713, -1.889935973073297859, 0.000000000000000000 ) ) ;
#5284=EDGE_LOOP ( 'NONE', ( #3970, #8862, #9147, #8681 ) ) ;
#5287=VERTEX_POINT ( 'NONE', #9229 ) ;
#5288=CARTESIAN_POINT ( 'NONE',  ( -12.85629483955644581, -68.90909090901422474, 2.086541329742040318 ) ) ;
#5293=CARTESIAN_POINT ( 'NONE',  ( -2.517691654963332357E-15, 90.00000000000000000, -1.589271161308885878E-16 ) ) ;
#5295=CARTESIAN_POINT ( 'NONE',  ( 8.943257790336033963, -76.35064935063256542, 10.27353203465967546 ) ) ;
#5297=CARTESIAN_POINT ( 'NONE',  ( 10.69346802281034492, 11.89973432371241380, 1.298086082554878758E-15 ) ) ;
#5298=( BOUNDED_SURFACE ( )  B_SPLINE_SURFACE ( 3, 3, ( 
 ( #2204, #4238, #13028, #126 ),
 ( #5297, #8593, #13890, #9851 ),
 ( #12826, #10623, #7471, #3192 ),
 ( #6560, #3258, #5562, #11813 ) ),
 .UNSPECIFIED., .F., .F., .F. ) 
 B_SPLINE_SURFACE_WITH_KNOTS ( ( 4, 4 ),
 ( 4, 4 ),
 ( 0.000000000000000000, 1.000000000000000000 ),
 ( 0.000000000000000000, 1.000000000000000000 ),
 .UNSPECIFIED. ) 
 GEOMETRIC_REPRESENTATION_ITEM ( )  RATIONAL_B_SPLINE_SURFACE ( (
 ( 1.000000000000000000, 0.3333333333333334259, 0.3333333333333334259, 1.000000000000000000),
 ( 1.000000000000000000, 0.3333333333333334259, 0.3333333333333334259, 1.000000000000000000),
 ( 1.000000000000000000, 0.3333333333333334259, 0.3333333333333334259, 1.000000000000000000),
 ( 1.000000000000000000, 0.3333333333333334259, 0.3333333333333334259, 1.000000000000000000) ) ) 
 REPRESENTATION_ITEM ( '' )  SURFACE ( )  );
#5300=CARTESIAN_POINT ( 'NONE',  ( -8.385254915620292238, 53.02855864072483882, -9.364084330386787485E-17 ) ) ;
#5304=ADVANCED_FACE ( 'NONE', ( #10274 ), #5260, .F. ) ;
#5310=CARTESIAN_POINT ( 'NONE',  ( -8.385254915620294014, 53.02855864072483882, 16.77050983124057737 ) ) ;
#5311=CARTESIAN_POINT ( 'NONE',  ( -5.049283603320642300, -77.73593560939509928, -8.777052014093525756 ) ) ;
#5312=DIRECTION ( 'NONE',  ( -1.000000000000000000, 0.000000000000000000, 0.000000000000000000 ) ) ;
#5316=EDGE_CURVE ( 'NONE', #11767, #11197, #3714, .T. ) ;
#5317=AXIS2_PLACEMENT_3D ( 'NONE', #8338, #12630, #12693 ) ;
#5318=CARTESIAN_POINT ( 'NONE',  ( -15.29705854078139282, 90.00000000000000000, -1.589271161308885878E-16 ) ) ;
#5320=CARTESIAN_POINT ( 'NONE',  ( 8.385254915620292238, 90.00000000000000000, 8.679704431140114636E-16 ) ) ;
#5323=CARTESIAN_POINT ( 'NONE',  ( -12.99579180576517068, 73.50828762700209040, -1.851135709604445740E-15 ) ) ;
#5324=ADVANCED_FACE ( 'NONE', ( #1972 ), #1905, .T. ) ;
#5325=CARTESIAN_POINT ( 'NONE',  ( 10.00000000000000000, 99.99999999999994316, 0.5000000000000000000 ) ) ;
#5326=CARTESIAN_POINT ( 'NONE',  ( -10.00000000000000000, 98.00000000000000000, 2.500000000000000000 ) ) ;
#5329=CARTESIAN_POINT ( 'NONE',  ( 10.00000000000000000, 90.00000000000000000, 2.500000000000000000 ) ) ;
#5330=CARTESIAN_POINT ( 'NONE',  ( -2.974680683949035842, -139.3888474069737242, 0.4051703307436435031 ) ) ;
#5332=ORIENTED_EDGE ( 'NONE', *, *, #2936, .T. ) ;
#5333=ORIENTED_EDGE ( 'NONE', *, *, #5133, .T. ) ;
#5340=CARTESIAN_POINT ( 'NONE',  ( 8.729408204557921991, -88.40583805251594640, -2.523542145620374377 ) ) ;
#5341=EDGE_CURVE ( 'NONE', #3627, #12589, #12136, .T. ) ;
#5343=CARTESIAN_POINT ( 'NONE',  ( 10.69381717166375623, 63.25855867215300066, -21.38763434332750535 ) ) ;
#5345=CARTESIAN_POINT ( 'NONE',  ( -1.010510313258165205, -79.21212121212225554, -9.990963482113517813 ) ) ;
#5347=LINE ( 'NONE', #8576, #12410 ) ;
#5349=ORIENTED_EDGE ( 'NONE', *, *, #1217, .F. ) ;
#5351=CARTESIAN_POINT ( 'NONE',  ( 12.99579180576516890, -11.31471392308272605, 3.183050967463142591E-15 ) ) ;
#5355=CYLINDRICAL_SURFACE ( 'NONE', #1010, 8.385254915620294014 ) ;
#5356=CARTESIAN_POINT ( 'NONE',  ( -1.111721538976399026, -76.35064935050264978, -4.681383094379441445 ) ) ;
#5358=CARTESIAN_POINT ( 'NONE',  ( 8.385254915620295790, 24.75422479069652937, -16.77050983124058448 ) ) ;
#5362=AXIS2_PLACEMENT_3D ( 'NONE', #7514, #12000, #10936 ) ;
#5363=DIRECTION ( 'NONE',  ( 1.000000000000000000, 0.000000000000000000, 0.000000000000000000 ) ) ;
#5369=CARTESIAN_POINT ( 'NONE',  ( 8.385254915620292238, 69.25350232273815720, 2.053795118489800793E-15 ) ) ;
#5371=VECTOR ( 'NONE', #2027, 1000.000000000000000 ) ;
#5373=CARTESIAN_POINT ( 'NONE',  ( -10.00000000000000000, 92.00000000000000000, 2.500000000000000000 ) ) ;
#5376=FACE_OUTER_BOUND ( 'NONE', #6217, .T. ) ;
#5378=CIRCLE ( 'NONE', #9202, 8.385254915620292238 ) ;
#5381=VERTEX_POINT ( 'NONE', #3422 ) ;
#5382=DIRECTION ( 'NONE',  ( 0.000000000000000000, 0.000000000000000000, -1.000000000000000000 ) ) ;
#5385=LINE ( 'NONE', #9672, #13202 ) ;
#5387=CIRCLE ( 'NONE', #8994, 15.29705854078139282 ) ;
#5390=EDGE_CURVE ( 'NONE', #3518, #7666, #3288, .T. ) ;
#5393=CARTESIAN_POINT ( 'NONE',  ( -8.162011110625947197, -94.39444938872335911, -1.717892133943179411 ) ) ;
#5394=DIRECTION ( 'NONE',  ( 1.000000000000000000, 0.000000000000000000, 0.000000000000000000 ) ) ;
#5401=CIRCLE ( 'NONE', #4974, 8.385254915620294014 ) ;
#5403=VERTEX_POINT ( 'NONE', #2369 ) ;
#5405=CARTESIAN_POINT ( 'NONE',  ( -2.517691654963332357E-15, 90.00000000000000000, -1.589271161308885878E-16 ) ) ;
#5406=FACE_OUTER_BOUND ( 'NONE', #12993, .T. ) ;
#5408=CARTESIAN_POINT ( 'NONE',  ( -2.301581772533134895, -133.0909090909001975, 3.282526544929068812 ) ) ;
#5410=CARTESIAN_POINT ( 'NONE',  ( -9.987599105575617031, -70.00000000000054001, -0.7388069302715789544 ) ) ;
#5411=CARTESIAN_POINT ( 'NONE',  ( 1.463793564955054638, -80.12121212121228098, -10.07802918118900237 ) ) ;
#5415=ADVANCED_FACE ( 'NONE', ( #4334 ), #3355, .T. ) ;
#5417=CARTESIAN_POINT ( 'NONE',  ( -8.385254915620292238, 71.87811454074363837, -2.234780678013320345E-15 ) ) ;
#5421=CARTESIAN_POINT ( 'NONE',  ( -15.29705854078138927, 90.00000000000000000, -1.589271161308885878E-16 ) ) ;
#5422=ORIENTED_EDGE ( 'NONE', *, *, #6956, .F. ) ;
#5426=CYLINDRICAL_SURFACE ( 'NONE', #1586, 8.385254915620294014 ) ;
#5427=CARTESIAN_POINT ( 'NONE',  ( -15.29705854078139282, 27.21102387199583816, -3.793083824326958666E-15 ) ) ;
#5429=CARTESIAN_POINT ( 'NONE',  ( -15.29705854078139105, 76.22148119144830503, -1.345962243664627229E-16 ) ) ;
#5431=CARTESIAN_POINT ( 'NONE',  ( -12.99579180576516535, 16.95961992694555676, -1.651422005635246569E-15 ) ) ;
#5433=EDGE_CURVE ( 'NONE', #1229, #8596, #9578, .T. ) ;
#5434=ORIENTED_EDGE ( 'NONE', *, *, #1830, .F. ) ;
#5437=EDGE_LOOP ( 'NONE', ( #11086, #4869, #9506, #798 ) ) ;
#5439=ORIENTED_EDGE ( 'NONE', *, *, #12038, .F. ) ;
#5440=FACE_OUTER_BOUND ( 'NONE', #12531, .T. ) ;
#5441=CARTESIAN_POINT ( 'NONE',  ( 10.69381717166374912, 53.83378072214353693, 21.38763434332751245 ) ) ;
#5444=B_SPLINE_CURVE_WITH_KNOTS ( 'NONE', 3,
 ( #446, #2610, #590, #8917, #4856, #8012, #1695, #2817, #12426, #6048, #8992, #10114, #9130, #4634, #6884, #1549, #5834, #13447, #3794, #5983, #12364, #2748, #7021, #10248, #9199, #13524, #3863, #12577 ),
 .UNSPECIFIED., .F., .F.,
 ( 4, 2, 2, 2, 2, 2, 2, 2, 2, 2, 2, 2, 2, 4 ),
 ( 0.000000000000000000, 0.002162634748517545339, 0.003243952122776318225, 0.004325269497035090678, 0.006487904245552661604, 0.008650538994070231663, 0.009731856368329017126, 0.01081317374258780085, 0.01189449111684658458, 0.01297580849110537005, 0.01513844323962291322, 0.01621976061388167439, 0.01676041930101106539, 0.01730107798814045639 ),
 .UNSPECIFIED. ) ;
#5446=CARTESIAN_POINT ( 'NONE',  ( 12.99553232110413248, 11.07475474455194053, 25.99106464220827561 ) ) ;
#5448=ORIENTED_EDGE ( 'NONE', *, *, #4190, .T. ) ;
#5449=ORIENTED_EDGE ( 'NONE', *, *, #5159, .T. ) ;
#5451=ORIENTED_EDGE ( 'NONE', *, *, #9124, .F. ) ;
#5452=CARTESIAN_POINT ( 'NONE',  ( -15.29705854078139105, 76.22148119144830503, -3.882960684162827838E-15 ) ) ;
#5454=CARTESIAN_POINT ( 'NONE',  ( 10.69381717166375267, 72.68333662216238622, 2.619229793989003556E-15 ) ) ;
#5455=VECTOR ( 'NONE', #11959, 1000.000000000000000 ) ;
#5456=DIRECTION ( 'NONE',  ( -2.797435172181481150E-17, 1.000000000000000000, -1.765856845898762549E-18 ) ) ;
#5460=CARTESIAN_POINT ( 'NONE',  ( -8.385254915620292238, 62.45333659073423860, -1.102836519679677113E-16 ) ) ;
#5461=FACE_OUTER_BOUND ( 'NONE', #12425, .T. ) ;
#5462=ORIENTED_EDGE ( 'NONE', *, *, #7650, .F. ) ;
#5464=EDGE_LOOP ( 'NONE', ( #179, #4010, #8731, #6372 ) ) ;
#5467=AXIS2_PLACEMENT_3D ( 'NONE', #323, #13245, #10059 ) ;
#5469=EDGE_CURVE ( 'NONE', #7762, #7874, #562, .T. ) ;
#5472=CARTESIAN_POINT ( 'NONE',  ( 12.99579180576516713, -1.889935973073297859, 3.183050967463142591E-15 ) ) ;
#5474=DIRECTION ( 'NONE',  ( 1.000000000000000000, 0.000000000000000000, 0.000000000000000000 ) ) ;
#5475=CARTESIAN_POINT ( 'NONE',  ( 8.385254915620292238, 5.904668890677672088, 1.018788103988028800E-15 ) ) ;
#5476=CARTESIAN_POINT ( 'NONE',  ( -3.039669588831499514, -137.4545454544692973, 0.1626128505621707299 ) ) ;
#5477=LINE ( 'NONE', #6744, #714 ) ;
#5478=CARTESIAN_POINT ( 'NONE',  ( -1.134746186792450207, -154.2164502169000855, -0.2399094883757922347 ) ) ;
#5479=CARTESIAN_POINT ( 'NONE',  ( -9.314636722532608104, -70.78787878787781551, -4.145366960882149954 ) ) ;
#5480=CARTESIAN_POINT ( 'NONE',  ( 8.385254915620292238, -15.56949922734665748, 16.77050983124059158 ) ) ;
#5482=ORIENTED_EDGE ( 'NONE', *, *, #11006, .T. ) ;
#5484=DIRECTION ( 'NONE',  ( -9.860761315262647568E-32, -3.204747427460360459E-31, 1.000000000000000000 ) ) ;
#5487=ADVANCED_FACE ( 'NONE', ( #7279 ), #12396, .T. ) ;
#5490=EDGE_CURVE ( 'NONE', #6441, #6908, #9913, .T. ) ;
#5494=ORIENTED_EDGE ( 'NONE', *, *, #8583, .F. ) ;
#5495=CIRCLE ( 'NONE', #8625, 48.00000000000001421 ) ;
#5500=ADVANCED_FACE ( 'NONE', ( #8467 ), #3136, .T. ) ;
#5505=CARTESIAN_POINT ( 'NONE',  ( 9.847276892489302169E-17, -3.520109059331727686, 6.216008680731233110E-18 ) ) ;
#5514=CARTESIAN_POINT ( 'NONE',  ( 12.99579180576516002, 54.65873172698324112, 25.99158361153033425 ) ) ;
#5516=AXIS2_PLACEMENT_3D ( 'NONE', #694, #1800, #2856 ) ;
#5518=VERTEX_POINT ( 'NONE', #9663 ) ;
#5524=CARTESIAN_POINT ( 'NONE',  ( -1.024862805779478135E-15, 36.63580182200523438, -6.469358145237827718E-17 ) ) ;
#5525=CARTESIAN_POINT ( 'NONE',  ( 0.9875500501441598633, -80.00464164738322381, -10.06307372056550342 ) ) ;
#5526=DIRECTION ( 'NONE',  ( -2.797435172181481150E-17, 1.000000000000000000, -1.765856845898762549E-18 ) ) ;
#5527=CARTESIAN_POINT ( 'NONE',  ( 4.267662252619970786, 91.33687515530506573, -2.605658972705547249 ) ) ;
#5528=CARTESIAN_POINT ( 'NONE',  ( 15.29705854078140348, -29.33764382806072746, 1.980000072520088949E-15 ) ) ;
#5530=ORIENTED_EDGE ( 'NONE', *, *, #5903, .T. ) ;
#5533=ORIENTED_EDGE ( 'NONE', *, *, #1284, .F. ) ;
#5534=CARTESIAN_POINT ( 'NONE',  ( -4.330127018922195425, 92.00000000000000000, 2.500000000000000000 ) ) ;
#5535=ORIENTED_EDGE ( 'NONE', *, *, #3869, .T. ) ;
#5540=CARTESIAN_POINT ( 'NONE',  ( -0.8539417517645131461, -80.00115723678993618, -9.969673860083380745 ) ) ;
#5541=CARTESIAN_POINT ( 'NONE',  ( 1.214590548353038368, -168.0000000000000568, -1.662759693958060225 ) ) ;
#5542=CARTESIAN_POINT ( 'NONE',  ( 0.2617580721754693696, -80.12121212121134306, -10.03731802028341136 ) ) ;
#5547=ORIENTED_EDGE ( 'NONE', *, *, #1889, .T. ) ;
#5550=ORIENTED_EDGE ( 'NONE', *, *, #8419, .F. ) ;
#5552=CYLINDRICAL_SURFACE ( 'NONE', #1588, 8.385254915620295790 ) ;
#5553=ORIENTED_EDGE ( 'NONE', *, *, #9317, .F. ) ;
#5554=CARTESIAN_POINT ( 'NONE',  ( -8.385254915620292238, 5.904668890677672088, -1.042679998336861873E-17 ) ) ;
#5558=CARTESIAN_POINT ( 'NONE',  ( -15.29705854078139282, 27.21102387199583816, -1.969450923410318186E-15 ) ) ;
#5561=CARTESIAN_POINT ( 'NONE',  ( -1.341290363786561812E-15, 47.94714734142005597, -8.466779837416320124E-17 ) ) ;
#5562=CARTESIAN_POINT ( 'NONE',  ( -15.29705854078138216, 10.24803554138234318, -30.59411708156277498 ) ) ;
#5563=CARTESIAN_POINT ( 'NONE',  ( -10.69381717166376156, -30.98922082794128130, -1.200169841498325292E-15 ) ) ;
#5566=CARTESIAN_POINT ( 'NONE',  ( 1.958204620527036497E-15, -70.00000000000000000, 1.236099792129133461E-16 ) ) ;
#5568=EDGE_CURVE ( 'NONE', #12557, #11359, #11025, .T. ) ;
#5573=EDGE_CURVE ( 'NONE', #3719, #1421, #6640, .T. ) ;
#5575=( BOUNDED_SURFACE ( )  B_SPLINE_SURFACE ( 3, 3, ( 
 ( #2359, #10834, #7548, #9874 ),
 ( #10904, #11765, #3406, #278 ),
 ( #2221, #9594, #5446, #1253 ),
 ( #1116, #4256, #8674, #6508 ) ),
 .UNSPECIFIED., .F., .F., .T. ) 
 B_SPLINE_SURFACE_WITH_KNOTS ( ( 4, 4 ),
 ( 4, 4 ),
 ( 0.000000000000000000, 1.000000000000000000 ),
 ( 0.000000000000000000, 1.000000000000000000 ),
 .UNSPECIFIED. ) 
 GEOMETRIC_REPRESENTATION_ITEM ( )  RATIONAL_B_SPLINE_SURFACE ( (
 ( 1.000000000000000000, 0.3333333333333334259, 0.3333333333333334259, 1.000000000000000000),
 ( 1.000000000000000000, 0.3333333333333334259, 0.3333333333333334259, 1.000000000000000000),
 ( 1.000000000000000000, 0.3333333333333334259, 0.3333333333333334259, 1.000000000000000000),
 ( 1.000000000000000000, 0.3333333333333334259, 0.3333333333333334259, 1.000000000000000000) ) ) 
 REPRESENTATION_ITEM ( '' )  SURFACE ( )  );
#5576=ORIENTED_EDGE ( 'NONE', *, *, #1952, .F. ) ;
#5577=DIRECTION ( 'NONE',  ( 0.000000000000000000, 0.000000000000000000, 1.000000000000000000 ) ) ;
#5587=VERTEX_POINT ( 'NONE', #1308 ) ;
#5589=CIRCLE ( 'NONE', #5150, 8.385254915620294014 ) ;
#5595=DIRECTION ( 'NONE',  ( 0.1234677578012386701, 0.000000000000000000, -0.9923485843107424653 ) ) ;
#5596=ORIENTED_EDGE ( 'NONE', *, *, #11995, .T. ) ;
#5598=DIRECTION ( 'NONE',  ( 0.000000000000000000, -1.000000000000000000, 0.000000000000000000 ) ) ;
#5600=DIRECTION ( 'NONE',  ( 1.000000000000000000, 0.000000000000000000, 0.000000000000000000 ) ) ;
#5601=DIRECTION ( 'NONE',  ( -2.797435172181481150E-17, 1.000000000000000000, -1.765856845898762549E-18 ) ) ;
#5603=CARTESIAN_POINT ( 'NONE',  ( 10.69381717166376333, -30.98922082794128130, 1.384171912460316962E-15 ) ) ;
#5604=DIRECTION ( 'NONE',  ( 0.000000000000000000, 0.000000000000000000, 1.000000000000000000 ) ) ;
#5609=CARTESIAN_POINT ( 'NONE',  ( -8.713593516913357817, -91.08576818318459800, -0.8596443958658561701 ) ) ;
#5611=CARTESIAN_POINT ( 'NONE',  ( -3.828023344975119979, 90.45717703472959670, 3.219997411495244322 ) ) ;
#5615=DIRECTION ( 'NONE',  ( -1.000000000000000000, 0.000000000000000000, 0.000000000000000000 ) ) ;
#5616=CARTESIAN_POINT ( 'NONE',  ( 10.69381717166375445, 34.98422482212468054, 2.619229793989003951E-15 ) ) ;
#5617=CARTESIAN_POINT ( 'NONE',  ( -12.99553232110414491, -7.774801155466915858, -3.169847907505149691E-15 ) ) ;
#5618=AXIS2_PLACEMENT_3D ( 'NONE', #7104, #10402, #12721 ) ;
#5619=DIRECTION ( 'NONE',  ( 1.000000000000000000, 0.000000000000000000, 0.000000000000000000 ) ) ;
#5620=CARTESIAN_POINT ( 'NONE',  ( -0.3237100442214350671, -158.0606060598179283, -0.5247744424615701231 ) ) ;
#5628=FACE_BOUND ( 'NONE', #10366, .T. ) ;
#5633=CARTESIAN_POINT ( 'NONE',  ( 4.330127018922190985, 90.00000000000000000, -4.500000000000000888 ) ) ;
#5635=DIRECTION ( 'NONE',  ( -1.000000000000000000, 0.000000000000000000, 0.000000000000000000 ) ) ;
#5637=CARTESIAN_POINT ( 'NONE',  ( -15.29705854078139105, 27.21102387199583816, -4.805077278827845308E-17 ) ) ;
#5638=CARTESIAN_POINT ( 'NONE',  ( -12.99579180576516713, 45.23395377697384134, -3.272288958712398313E-15 ) ) ;
#5640=( BOUNDED_SURFACE ( )  B_SPLINE_SURFACE ( 3, 3, ( 
 ( #9429, #10539, #11661, #13741 ),
 ( #944, #12663, #10671, #36 ),
 ( #6334, #5343, #13805, #9628 ),
 ( #4154, #3043, #5207, #8438 ) ),
 .UNSPECIFIED., .F., .F., .T. ) 
 B_SPLINE_SURFACE_WITH_KNOTS ( ( 4, 4 ),
 ( 4, 4 ),
 ( 0.000000000000000000, 1.000000000000000000 ),
 ( 0.000000000000000000, 1.000000000000000000 ),
 .UNSPECIFIED. ) 
 GEOMETRIC_REPRESENTATION_ITEM ( )  RATIONAL_B_SPLINE_SURFACE ( (
 ( 1.000000000000000000, 0.3333333333333334259, 0.3333333333333334259, 1.000000000000000000),
 ( 1.000000000000000000, 0.3333333333333334259, 0.3333333333333334259, 1.000000000000000000),
 ( 1.000000000000000000, 0.3333333333333334259, 0.3333333333333334259, 1.000000000000000000),
 ( 1.000000000000000000, 0.3333333333333334259, 0.3333333333333334259, 1.000000000000000000) ) ) 
 REPRESENTATION_ITEM ( '' )  SURFACE ( )  );
#5641=DIRECTION ( 'NONE',  ( -2.797435172181481150E-17, 1.000000000000000000, -1.765856845898762549E-18 ) ) ;
#5642=DIRECTION ( 'NONE',  ( -2.797435172181479917E-17, 1.000000000000000000, -1.765856845898779112E-18 ) ) ;
#5643=CARTESIAN_POINT ( 'NONE',  ( -8.385254915620294014, -31.79444290936001138, -9.146086898988387700E-16 ) ) ;
#5647=CARTESIAN_POINT ( 'NONE',  ( -1.651792843486753513E-16, 5.904668890677672088, -1.042679998336861873E-17 ) ) ;
#5649=ORIENTED_EDGE ( 'NONE', *, *, #11273, .F. ) ;
#5650=CARTESIAN_POINT ( 'NONE',  ( -8.385254915620294014, 3.280056672672198914, -5.792110530374064999E-18 ) ) ;
#5653=B_SPLINE_CURVE_WITH_KNOTS ( 'NONE', 3,
 ( #4670, #2713, #11196, #486, #619, #11045, #3898, #3685, #6773, #8957, #8041, #1589, #9157, #7970, #5720, #4879 ),
 .UNSPECIFIED., .F., .F.,
 ( 4, 2, 2, 2, 2, 2, 2, 4 ),
 ( 0.000000000000000000, 0.0005014865247272642327, 0.001002973049454528465, 0.001504459574181792698, 0.002005946098909056931, 0.002507432623636320947, 0.003008919148363585396, 0.004011892197818113862 ),
 .UNSPECIFIED. ) ;
#5654=EDGE_CURVE ( 'NONE', #9893, #3489, #295, .T. ) ;
#5655=ORIENTED_EDGE ( 'NONE', *, *, #2379, .F. ) ;
#5658=EDGE_CURVE ( 'NONE', #10679, #6325, #6782, .T. ) ;
#5659=AXIS2_PLACEMENT_3D ( 'NONE', #7813, #11123, #4667 ) ;
#5661=DIRECTION ( 'NONE',  ( -1.000000000000000000, 0.000000000000000000, 0.000000000000000000 ) ) ;
#5662=CARTESIAN_POINT ( 'NONE',  ( 7.521705593689169689, -75.41806776122028566, 6.778495972023521610 ) ) ;
#5667=ORIENTED_EDGE ( 'NONE', *, *, #5736, .F. ) ;
#5671=CARTESIAN_POINT ( 'NONE',  ( 0.6173387890061953209, -69.99999999999998579, -4.961742921553712549 ) ) ;
#5672=CIRCLE ( 'NONE', #5002, 2.000000000000003109 ) ;
#5676=CARTESIAN_POINT ( 'NONE',  ( -7.861734782780223085, -72.85454080786820441, -6.394819305376118201 ) ) ;
#5680=CARTESIAN_POINT ( 'NONE',  ( 12.99553232110413781, 58.19864449459907974, 3.182987412051231773E-15 ) ) ;
#5688=CARTESIAN_POINT ( 'NONE',  ( -15.29705854078138394, 57.37192529142944863, -30.59411708156277854 ) ) ;
#5689=LINE ( 'NONE', #4561, #12180 ) ;
#5690=CARTESIAN_POINT ( 'NONE',  ( 4.418010223187812890, -106.9090909090834742, -5.547116815808206702 ) ) ;
#5692=CARTESIAN_POINT ( 'NONE',  ( 3.189539364161639412, -137.4545454545230143, -1.430838129453004370 ) ) ;
#5694=LINE ( 'NONE', #2617, #12683 ) ;
#5696=CARTESIAN_POINT ( 'NONE',  ( -15.29705854078139815, -18.02629830864593785, 30.59411708156277854 ) ) ;
#5697=DIRECTION ( 'NONE',  ( -2.797435172181481150E-17, 1.000000000000000000, -1.765856845898762549E-18 ) ) ;
#5699=ORIENTED_EDGE ( 'NONE', *, *, #3161, .F. ) ;
#5700=ORIENTED_EDGE ( 'NONE', *, *, #8583, .T. ) ;
#5702=ORIENTED_EDGE ( 'NONE', *, *, #6899, .T. ) ;
#5703=DIRECTION ( 'NONE',  ( -2.797435172181481150E-17, 1.000000000000000000, -1.765856845898762549E-18 ) ) ;
#5706=ORIENTED_EDGE ( 'NONE', *, *, #7517, .F. ) ;
#5710=CARTESIAN_POINT ( 'NONE',  ( 8.385254915620292238, 15.32944684068712782, 1.002145295323929148E-15 ) ) ;
#5711=DIRECTION ( 'NONE',  ( -1.000000000000000000, 0.000000000000000000, 0.000000000000000000 ) ) ;
#5713=CARTESIAN_POINT ( 'NONE',  ( -10.69381717166376156, -30.98922082794128130, -1.200169841498325292E-15 ) ) ;
#5714=CARTESIAN_POINT ( 'NONE',  ( -7.521705564882291029, -75.41806779423124851, -6.778496005277558467 ) ) ;
#5716=CARTESIAN_POINT ( 'NONE',  ( -12.99553232110414136, -36.04913500549519512, -1.464178482349251183E-15 ) ) ;
#5717=FACE_OUTER_BOUND ( 'NONE', #2512, .T. ) ;
#5719=CARTESIAN_POINT ( 'NONE',  ( 10.00000000000000711, 139.9999999999999716, 2.500000000000000000 ) ) ;
#5720=CARTESIAN_POINT ( 'NONE',  ( 2.482729886976819511, 90.00000000000001421, 4.353114590951097540 ) ) ;
#5721=ORIENTED_EDGE ( 'NONE', *, *, #8673, .T. ) ;
#5723=AXIS2_PLACEMENT_3D ( 'NONE', #6585, #10785, #12927 ) ;
#5726=ORIENTED_EDGE ( 'NONE', *, *, #271, .T. ) ;
#5727=CARTESIAN_POINT ( 'NONE',  ( 5.042740091284176371E-16, -18.02629830864596627, 3.183186227453577089E-17 ) ) ;
#5728=CARTESIAN_POINT ( 'NONE',  ( 12.99579180576516890, 64.08350967699263379, 0.000000000000000000 ) ) ;
#5729=DIRECTION ( 'NONE',  ( 1.000000000000000000, 0.000000000000000000, 0.000000000000000000 ) ) ;
#5731=DIRECTION ( 'NONE',  ( 2.797435172181480534E-17, -1.000000000000000000, 1.765856845898762164E-18 ) ) ;
#5732=CARTESIAN_POINT ( 'NONE',  ( 4.918402716924989981, -70.00000000000000000, -0.8996192050778424321 ) ) ;
#5733=EDGE_LOOP ( 'NONE', ( #6029, #6409, #1054, #647, #4966 ) ) ;
#5736=EDGE_CURVE ( 'NONE', #2504, #1229, #1186, .T. ) ;
#5741=TOROIDAL_SURFACE ( 'NONE', #394, 48.00000000000001421, 2.000000000000000000 ) ;
#5742=CARTESIAN_POINT ( 'NONE',  ( 15.29705854078138572, 57.37192529142945574, 1.773704474924340342E-15 ) ) ;
#5745=CARTESIAN_POINT ( 'NONE',  ( -0.9319787617451019690, -80.77036012704304824, -9.970313506240117363 ) ) ;
#5746=FACE_OUTER_BOUND ( 'NONE', #10922, .T. ) ;
#5747=( BOUNDED_SURFACE ( )  B_SPLINE_SURFACE ( 3, 3, ( 
 ( #5528, #9816, #221, #4478 ),
 ( #2446, #7701, #13132, #3486 ),
 ( #5603, #7768, #3715, #2665 ),
 ( #3853, #13511, #8135, #6803 ) ),
 .UNSPECIFIED., .F., .F., .T. ) 
 B_SPLINE_SURFACE_WITH_KNOTS ( ( 4, 4 ),
 ( 4, 4 ),
 ( 0.000000000000000000, 1.000000000000000000 ),
 ( 0.000000000000000000, 1.000000000000000000 ),
 .UNSPECIFIED. ) 
 GEOMETRIC_REPRESENTATION_ITEM ( )  RATIONAL_B_SPLINE_SURFACE ( (
 ( 1.000000000000000000, 0.3333333333333334259, 0.3333333333333334259, 1.000000000000000000),
 ( 1.000000000000000000, 0.3333333333333334259, 0.3333333333333334259, 1.000000000000000000),
 ( 1.000000000000000000, 0.3333333333333334259, 0.3333333333333334259, 1.000000000000000000),
 ( 1.000000000000000000, 0.3333333333333334259, 0.3333333333333334259, 1.000000000000000000) ) ) 
 REPRESENTATION_ITEM ( '' )  SURFACE ( )  );
#5749=ORIENTED_EDGE ( 'NONE', *, *, #6079, .T. ) ;
#5752=CARTESIAN_POINT ( 'NONE',  ( -8.385254915620299343, -6.144721277337256815, 16.77050983124059158 ) ) ;
#5753=EDGE_CURVE ( 'NONE', #2743, #4734, #2796, .T. ) ;
#5754=ADVANCED_FACE ( 'NONE', ( #696 ), #9968, .T. ) ;
#5756=CARTESIAN_POINT ( 'NONE',  ( -15.29705854078139815, -27.45107625865536960, 30.59411708156277854 ) ) ;
#5758=CARTESIAN_POINT ( 'NONE',  ( 9.082088619475626956, -71.90909090908733958, 4.345719731624217985 ) ) ;
#5760=CARTESIAN_POINT ( 'NONE',  ( 4.545447045960947285, 90.76293396533760927, 2.092248084982493594 ) ) ;
#5764=CARTESIAN_POINT ( 'NONE',  ( 1.652786589946103835, -148.3982683981489856, 1.815848636690450268 ) ) ;
#5768=SURFACE_SIDE_STYLE ('',( #12005 ) ) ;
#5773=CARTESIAN_POINT ( 'NONE',  ( -0.01104702316550528959, -159.4786160828277275, 1.513430353261248973 ) ) ;
#5775=CARTESIAN_POINT ( 'NONE',  ( -0.4631675488762010962, -123.7427791793036391, 4.812436839529170562 ) ) ;
#5776=CARTESIAN_POINT ( 'NONE',  ( 1.750805008852563294, -80.00120739911564272, 9.924274110580476815 ) ) ;
#5778=ADVANCED_FACE ( 'NONE', ( #2509 ), #3325, .T. ) ;
#5780=ORIENTED_EDGE ( 'NONE', *, *, #8985, .F. ) ;
#5784=B_SPLINE_CURVE_WITH_KNOTS ( 'NONE', 3,
 ( #989, #11707, #13785, #8420 ),
 .UNSPECIFIED., .F., .F.,
 ( 4, 4 ),
 ( 0.000000000000000000, 1.000000000000000000 ),
 .UNSPECIFIED. ) ;
#5786=FACE_OUTER_BOUND ( 'NONE', #4930, .T. ) ;
#5787=AXIS2_PLACEMENT_3D ( 'NONE', #7215, #7280, #12762 ) ;
#5789=LINE ( 'NONE', #8108, #8083 ) ;
#5790=CARTESIAN_POINT ( 'NONE',  ( -15.29705854078139815, 64.91013567203349055, 30.59411708156277854 ) ) ;
#5791=AXIS2_PLACEMENT_3D ( 'NONE', #11577, #3085, #11640 ) ;
#5792=CARTESIAN_POINT ( 'NONE',  ( -15.29705854078139282, 55.48535772202409078, -9.797919878057798703E-17 ) ) ;
#5793=CARTESIAN_POINT ( 'NONE',  ( 12.99553232110414847, -7.774801155466914970, -25.99106464220827917 ) ) ;
#5796=ORIENTED_EDGE ( 'NONE', *, *, #13243, .F. ) ;
#5797=CARTESIAN_POINT ( 'NONE',  ( 11.18807966363703876, -153.6493506493829102, -7.768796162325410926 ) ) ;
#5799=ORIENTED_EDGE ( 'NONE', *, *, #3702, .F. ) ;
#5801=CARTESIAN_POINT ( 'NONE',  ( 8.385254915620295790, -31.79444290936001138, 1.085359338644428786E-15 ) ) ;
#5803=ORIENTED_EDGE ( 'NONE', *, *, #1814, .T. ) ;
#5804=CARTESIAN_POINT ( 'NONE',  ( 12.99579180576516535, 35.80917582696438473, 1.535149190374665400E-15 ) ) ;
#5807=CARTESIAN_POINT ( 'NONE',  ( -15.29705854078139282, 19.67281349139177138, 30.59411708156277498 ) ) ;
#5809=CARTESIAN_POINT ( 'NONE',  ( 15.29705854078139282, -38.76242177807012723, 3.746698755667522411E-15 ) ) ;
#5814=ORIENTED_EDGE ( 'NONE', *, *, #5753, .F. ) ;
#5815=ORIENTED_EDGE ( 'NONE', *, *, #7684, .F. ) ;
#5816=CARTESIAN_POINT ( 'NONE',  ( 8.385254915620299343, -34.41905512736551032, 1.085359338644428786E-15 ) ) ;
#5817=EDGE_CURVE ( 'NONE', #2958, #11894, #6229, .T. ) ;
#5819=FACE_OUTER_BOUND ( 'NONE', #700, .T. ) ;
#5822=CARTESIAN_POINT ( 'NONE',  ( 8.296475850350821801, -93.99331153395371530, 1.275032287086958815 ) ) ;
#5823=CARTESIAN_POINT ( 'NONE',  ( -10.69381717166375623, 16.13466892210585613, -2.653091794345379119E-15 ) ) ;
#5826=EDGE_LOOP ( 'NONE', ( #2689, #2148, #1901, #3223 ) ) ;
#5827=CARTESIAN_POINT ( 'NONE',  ( -6.913174563124464989, -94.54126257933998545, -4.633799819412218746 ) ) ;
#5829=CIRCLE ( 'NONE', #13008, 15.29705854078139105 ) ;
#5834=CARTESIAN_POINT ( 'NONE',  ( 7.476762187090618461, -73.27151468276238688, 6.844715442818731788 ) ) ;
#5835=ADVANCED_FACE ( 'NONE', ( #8191 ), #10626, .T. ) ;
#5838=CARTESIAN_POINT ( 'NONE',  ( -4.114679947050897013, -133.0909090909224517, -0.08888163046369852716 ) ) ;
#5841=CARTESIAN_POINT ( 'NONE',  ( -6.267146549262783140, -111.2727272727292700, 1.834821170859244344 ) ) ;
#5843=CIRCLE ( 'NONE', #3132, 15.29705854078138927 ) ;
#5845=AXIS2_PLACEMENT_3D ( 'NONE', #606, #2627, #9010 ) ;
#5848=CARTESIAN_POINT ( 'NONE',  ( -1.604942417060130136E-15, 57.37192529142945574, -1.013106070382630377E-16 ) ) ;
#5849=ADVANCED_FACE ( 'NONE', ( #10362 ), #12474, .F. ) ;
#5853=CARTESIAN_POINT ( 'NONE',  ( -0.1852015970780942489, -159.9999997928953235, 1.488522644435750886 ) ) ;
#5855=CARTESIAN_POINT ( 'NONE',  ( 6.202303966384370426, -111.0571250337653879, -1.156479532967471302 ) ) ;
#5856=CIRCLE ( 'NONE', #10105, 15.29705854078138749 ) ;
#5857=CIRCLE ( 'NONE', #11228, 2.000000000000003109 ) ;
#5858=DIRECTION ( 'NONE',  ( -1.000000000000000000, 0.000000000000000000, 0.000000000000000000 ) ) ;
#5860=VERTEX_POINT ( 'NONE', #5300 ) ;
#5861=ORIENTED_EDGE ( 'NONE', *, *, #9043, .T. ) ;
#5862=DIRECTION ( 'NONE',  ( 1.000000000000000000, 0.000000000000000000, 0.000000000000000000 ) ) ;
#5863=ORIENTED_EDGE ( 'NONE', *, *, #3616, .T. ) ;
#5864=CARTESIAN_POINT ( 'NONE',  ( 1.238865979958289509, -140.6626200957464334, 2.568243908262899389 ) ) ;
#5866=CARTESIAN_POINT ( 'NONE',  ( 4.658064847839351152, 90.49194140877688142, -1.819915145876241036 ) ) ;
#5869=EDGE_CURVE ( 'NONE', #10278, #10788, #6553, .T. ) ;
#5870=DIRECTION ( 'NONE',  ( -1.000000000000000000, 0.000000000000000000, 0.000000000000000000 ) ) ;
#5873=CARTESIAN_POINT ( 'NONE',  ( -8.385254915620294014, 62.45333659073424570, 16.77050983124057737 ) ) ;
#5874=ADVANCED_FACE ( 'NONE', ( #833 ), #9581, .F. ) ;
#5875=AXIS2_PLACEMENT_3D ( 'NONE', #7413, #10062, #2486 ) ;
#5876=CARTESIAN_POINT ( 'NONE',  ( 8.385254915620295790, -6.144721277337255927, 1.035430912652129043E-15 ) ) ;
#5877=VERTEX_POINT ( 'NONE', #9384 ) ;
#5878=DIRECTION ( 'NONE',  ( -2.797435172181481150E-17, 1.000000000000000000, -1.765856845898762549E-18 ) ) ;
#5880=CARTESIAN_POINT ( 'NONE',  ( -6.356408396254766835, -164.3636363616015217, -0.5463072361628438234 ) ) ;
#5883=CARTESIAN_POINT ( 'NONE',  ( -12.99579180576516002, 35.80917582696438473, -25.99158361153033070 ) ) ;
#5884=DIRECTION ( 'NONE',  ( -1.000000000000000000, 0.000000000000000000, 0.000000000000000000 ) ) ;
#5886=EDGE_CURVE ( 'NONE', #430, #10108, #7888, .T. ) ;
#5889=CARTESIAN_POINT ( 'NONE',  ( 2.008006476061143353, -80.00378950643523979, 9.910921260988354575 ) ) ;
#5890=ORIENTED_EDGE ( 'NONE', *, *, #6360, .F. ) ;
#5892=CARTESIAN_POINT ( 'NONE',  ( 10.69346802281035202, -25.79937747632526879, -21.38693604562069339 ) ) ;
#5893=ORIENTED_EDGE ( 'NONE', *, *, #13852, .T. ) ;
#5897=CARTESIAN_POINT ( 'NONE',  ( -8.043602924566211954, -72.64880124666912309, -6.161478634331895243 ) ) ;
#5899=CARTESIAN_POINT ( 'NONE',  ( 7.733904924929606572, -95.38813776267139133, 2.765113012216059651 ) ) ;
#5900=CARTESIAN_POINT ( 'NONE',  ( -8.385254915620294014, 50.40394642271930081, -16.77050983124059158 ) ) ;
#5901=ORIENTED_EDGE ( 'NONE', *, *, #13592, .T. ) ;
#5902=VECTOR ( 'NONE', #13699, 1000.000000000000000 ) ;
#5903=EDGE_CURVE ( 'NONE', #4658, #7574, #10401, .T. ) ;
#5904=ORIENTED_EDGE ( 'NONE', *, *, #8743, .T. ) ;
#5905=CARTESIAN_POINT ( 'NONE',  ( 9.456627357064096628, -73.18181818181959386, 3.908318357316015401 ) ) ;
#5910=CARTESIAN_POINT ( 'NONE',  ( -12.99553232110414491, -17.19957910547634228, -3.161261631924336761E-15 ) ) ;
#5911=CARTESIAN_POINT ( 'NONE',  ( -3.628753873973424415, -79.03030303036898374, -9.983370075638070773 ) ) ;
#5913=B_SPLINE_CURVE_WITH_KNOTS ( 'NONE', 3,
 ( #6762, #1433, #2562, #5710 ),
 .UNSPECIFIED., .F., .F.,
 ( 4, 4 ),
 ( 0.000000000000000000, 1.000000000000000000 ),
 .UNSPECIFIED. ) ;
#5914=DIRECTION ( 'NONE',  ( 1.000000000000000000, 0.000000000000000000, 0.000000000000000000 ) ) ;
#5915=DIRECTION ( 'NONE',  ( 1.000000000000000000, 1.156482317317871133E-15, 0.000000000000000000 ) ) ;
#5919=ORIENTED_EDGE ( 'NONE', *, *, #8489, .F. ) ;
#5920=AXIS2_PLACEMENT_3D ( 'NONE', #7249, #11600, #11534 ) ;
#5921=ADVANCED_FACE ( 'NONE', ( #12546 ), #8390, .T. ) ;
#5922=CARTESIAN_POINT ( 'NONE',  ( 1.479030741744671973, -121.1096557515223680, 4.854982109747082220 ) ) ;
#5926=CIRCLE ( 'NONE', #6147, 15.29705854078138572 ) ;
#5928=DIRECTION ( 'NONE',  ( -2.797435172181481150E-17, 1.000000000000000000, -1.765856845898762549E-18 ) ) ;
#5929=EDGE_CURVE ( 'NONE', #4671, #12589, #7446, .T. ) ;
#5930=ORIENTED_EDGE ( 'NONE', *, *, #4702, .T. ) ;
#5931=DIRECTION ( 'NONE',  ( 0.000000000000000000, 0.000000000000000000, 1.000000000000000000 ) ) ;
#5932=CARTESIAN_POINT ( 'NONE',  ( 3.705099044711014589, -132.0105060180018768, -0.8975303730290892235 ) ) ;
#5933=LINE ( 'NONE', #8033, #7808 ) ;
#5934=CARTESIAN_POINT ( 'NONE',  ( 15.29705854078139282, -38.76242177807012723, 1.940132561565339224E-15 ) ) ;
#5940=EDGE_CURVE ( 'NONE', #8621, #10317, #11684, .T. ) ;
#5944=CARTESIAN_POINT ( 'NONE',  ( -0.003226301100687127901, -100.2727272727200756, -4.613888802083975449 ) ) ;
#5946=ORIENTED_EDGE ( 'NONE', *, *, #13247, .T. ) ;
#5947=AXIS2_PLACEMENT_3D ( 'NONE', #13021, #252, #13098 ) ;
#5949=ORIENTED_EDGE ( 'NONE', *, *, #13247, .F. ) ;
#5950=CARTESIAN_POINT ( 'NONE',  ( -4.974937185533102380, 90.00000000000000000, -0.5000000000000000000 ) ) ;
#5951=EDGE_CURVE ( 'NONE', #11359, #4067, #11565, .T. ) ;
#5953=CARTESIAN_POINT ( 'NONE',  ( -10.12341346681890819, -72.18181818172617170, -6.554034102534079587 ) ) ;
#5956=CARTESIAN_POINT ( 'NONE',  ( -2.403405165857241954E-13, -159.9999999999998010, -2.442165393523598738E-13 ) ) ;
#5958=ORIENTED_EDGE ( 'NONE', *, *, #6216, .T. ) ;
#5960=ADVANCED_FACE ( 'NONE', ( #3462 ), #4379, .T. ) ;
#5961=CARTESIAN_POINT ( 'NONE',  ( -3.122627689365423453, -81.55733635889028221, 9.361082846595628837 ) ) ;
#5962=AXIS2_PLACEMENT_3D ( 'NONE', #8100, #667, #3593 ) ;
#5971=CARTESIAN_POINT ( 'NONE',  ( 4.606570477487116122, -99.66561582491799243, 6.166945419414991747 ) ) ;
#5972=CARTESIAN_POINT ( 'NONE',  ( -10.69346802281035025, 49.59884612375012125, -2.736290265663450252E-15 ) ) ;
#5973=CIRCLE ( 'NONE', #6398, 50.00000000000001421 ) ;
#5978=ORIENTED_EDGE ( 'NONE', *, *, #13566, .F. ) ;
#5979=CARTESIAN_POINT ( 'NONE',  ( -15.29705854078139460, -27.45107625865536605, -1.776400035956490916E-15 ) ) ;
#5980=VECTOR ( 'NONE', #11119, 1000.000000000000000 ) ;
#5983=CARTESIAN_POINT ( 'NONE',  ( 8.558795037935681194, -72.03745727283919109, 5.439008144249546817 ) ) ;
#5984=CARTESIAN_POINT ( 'NONE',  ( -5.655105406264300250, -85.78354978356081517, 8.815184813460382074 ) ) ;
#5985=FACE_OUTER_BOUND ( 'NONE', #938, .T. ) ;
#5987=CARTESIAN_POINT ( 'NONE',  ( -5.770059030975961178, -111.2727272727253904, 3.008649887263203926 ) ) ;
#5988=DIRECTION ( 'NONE',  ( -1.000000000000000000, 0.000000000000000000, 0.000000000000000000 ) ) ;
#5989=CARTESIAN_POINT ( 'NONE',  ( 8.385254915620288685, 34.17900274070598243, 9.688596779957292534E-16 ) ) ;
#5990=ORIENTED_EDGE ( 'NONE', *, *, #8238, .F. ) ;
#5992=TOROIDAL_SURFACE ( 'NONE', #7087, 77.99999999999997158, 2.000000000000000000 ) ;
#5993=ORIENTED_EDGE ( 'NONE', *, *, #2967, .T. ) ;
#5994=CARTESIAN_POINT ( 'NONE',  ( 1.403442481258843078, -154.8168939350541393, 0.8939811563333199818 ) ) ;
#5996=CARTESIAN_POINT ( 'NONE',  ( 3.916815862944407645, -105.5671819316534936, -5.801851910426949921 ) ) ;
#5998=DIRECTION ( 'NONE',  ( -0.000000000000000000, -0.000000000000000000, -1.000000000000000000 ) ) ;
#6001=CARTESIAN_POINT ( 'NONE',  ( -2.237684797877293663E-15, 79.99058638175036151, -1.412519245696701158E-16 ) ) ;
#6002=CARTESIAN_POINT ( 'NONE',  ( 2.144143433502907037, -126.4672479063739559, -3.929051445287345512 ) ) ;
#6011=ORIENTED_EDGE ( 'NONE', *, *, #12123, .F. ) ;
#6012=CARTESIAN_POINT ( 'NONE',  ( 12.97432671025186224, -68.90909090921057611, 1.142286363980197006 ) ) ;
#6013=ORIENTED_EDGE ( 'NONE', *, *, #2999, .T. ) ;
#6017=CARTESIAN_POINT ( 'NONE',  ( 3.042673274263369976, -100.2727272727297105, 12.70187379131525418 ) ) ;
#6020=CARTESIAN_POINT ( 'NONE',  ( 10.69381717166375267, -21.56444287793185310, 21.38763434332751601 ) ) ;
#6023=CARTESIAN_POINT ( 'NONE',  ( -4.961407659643952250, 90.00000000000001421, 0.6346170828971220423 ) ) ;
#6024=ADVANCED_FACE ( 'NONE', ( #7673 ), #12959, .T. ) ;
#6025=ORIENTED_EDGE ( 'NONE', *, *, #11862, .T. ) ;
#6026=EDGE_CURVE ( 'NONE', #3686, #2454, #13550, .T. ) ;
#6027=CIRCLE ( 'NONE', #13886, 15.29705854078139460 ) ;
#6029=ORIENTED_EDGE ( 'NONE', *, *, #8487, .T. ) ;
#6031=CARTESIAN_POINT ( 'NONE',  ( -8.385254915620290461, -12.94488700934118341, -16.77050983124058803 ) ) ;
#6036=CARTESIAN_POINT ( 'NONE',  ( 4.498378629186895239, -85.01274099036943710, -8.404829403884384931 ) ) ;
#6037=VECTOR ( 'NONE', #6333, 1000.000000000000114 ) ;
#6038=CYLINDRICAL_SURFACE ( 'NONE', #10701, 5.000000000000000000 ) ;
#6042=AXIS2_PLACEMENT_3D ( 'NONE', #4748, #9023, #10964 ) ;
#6045=CIRCLE ( 'NONE', #8716, 22.99999999999999645 ) ;
#6048=CARTESIAN_POINT ( 'NONE',  ( 4.711442140758930641, -75.83792211546017370, 8.965827202672375762 ) ) ;
#6050=CARTESIAN_POINT ( 'NONE',  ( 10.69381717166375445, 44.40900277213413716, 2.619229793989003951E-15 ) ) ;
#6052=DIRECTION ( 'NONE',  ( 2.797435172181480534E-17, -1.000000000000000000, 1.765856845898762164E-18 ) ) ;
#6059=AXIS2_PLACEMENT_3D ( 'NONE', #7692, #11974, #5595 ) ;
#6062=CARTESIAN_POINT ( 'NONE',  ( 5.365917630196002541, -107.8841580301423448, -3.999906080763434346 ) ) ;
#6065=FACE_OUTER_BOUND ( 'NONE', #296, .T. ) ;
#6066=CARTESIAN_POINT ( 'NONE',  ( -2.517691654963332357E-15, 90.00000000000000000, -1.589271161308885878E-16 ) ) ;
#6067=AXIS2_PLACEMENT_3D ( 'NONE', #8101, #2834, #13599 ) ;
#6070=CARTESIAN_POINT ( 'NONE',  ( -39.99999999999999289, 100.0000000000000000, 0.5000000000000000000 ) ) ;
#6071=FACE_OUTER_BOUND ( 'NONE', #7369, .T. ) ;
#6073=AXIS2_PLACEMENT_3D ( 'NONE', #2218, #3135, #1181 ) ;
#6077=CARTESIAN_POINT ( 'NONE',  ( 8.385254915620288685, 71.87811454074363837, 9.022884433393296612E-16 ) ) ;
#6079=EDGE_CURVE ( 'NONE', #4734, #10317, #12626, .T. ) ;
#6082=CARTESIAN_POINT ( 'NONE',  ( 12.99553232110413781, 58.19864449459907974, 0.000000000000000000 ) ) ;
#6083=DIRECTION ( 'NONE',  ( -1.000000000000000000, 0.000000000000000000, 0.000000000000000000 ) ) ;
#6085=CARTESIAN_POINT ( 'NONE',  ( -4.481549108000151271, -153.6493506493174550, 1.751282401330790162 ) ) ;
#6087=B_SPLINE_CURVE_WITH_KNOTS ( 'NONE', 3,
 ( #2443, #10099, #12208, #10993 ),
 .UNSPECIFIED., .F., .F.,
 ( 4, 4 ),
 ( 0.000000000000000000, 1.000000000000000000 ),
 .UNSPECIFIED. ) ;
#6089=DIRECTION ( 'NONE',  ( 1.000000000000000000, 0.000000000000000000, 0.000000000000000000 ) ) ;
#6092=B_SPLINE_CURVE_WITH_KNOTS ( 'NONE', 3,
 ( #6928, #8058, #10991, #11069 ),
 .UNSPECIFIED., .F., .F.,
 ( 4, 4 ),
 ( 0.000000000000000000, 1.000000000000000000 ),
 .UNSPECIFIED. ) ;
#6093=CARTESIAN_POINT ( 'NONE',  ( 12.97449437267217043, -39.59556244224027211, 25.94898874534434796 ) ) ;
#6094=ORIENTED_EDGE ( 'NONE', *, *, #6602, .F. ) ;
#6096=AXIS2_PLACEMENT_3D ( 'NONE', #12530, #12732, #8312 ) ;
#6097=EDGE_CURVE ( 'NONE', #1633, #2083, #9472, .T. ) ;
#6098=EDGE_CURVE ( 'NONE', #7969, #6913, #968, .T. ) ;
#6100=EDGE_CURVE ( 'NONE', #2744, #10763, #3872, .T. ) ;
#6104=CARTESIAN_POINT ( 'NONE',  ( 8.385254915620295790, 31.55439052270045508, 9.996449125125102610E-16 ) ) ;
#6109=CARTESIAN_POINT ( 'NONE',  ( -2.517691654963332357E-15, 90.00000000000000000, -1.589271161308885878E-16 ) ) ;
#6111=ADVANCED_FACE ( 'NONE', ( #11040 ), #413, .T. ) ;
#6112=EDGE_CURVE ( 'NONE', #11046, #11396, #1526, .T. ) ;
#6114=CARTESIAN_POINT ( 'NONE',  ( -2.482729886976823952, 90.00000000000001421, -4.353114590951097540 ) ) ;
#6116=CARTESIAN_POINT ( 'NONE',  ( 11.81226048336477064, -40.00941361824966691, 1.498154114293980678E-15 ) ) ;
#6117=ORIENTED_EDGE ( 'NONE', *, *, #11756, .T. ) ;
#6118=EDGE_CURVE ( 'NONE', #13042, #3901, #12100, .T. ) ;
#6122=CARTESIAN_POINT ( 'NONE',  ( 25.00000000000000355, 120.0000000000000284, -0.5000000000000000000 ) ) ;
#6125=CARTESIAN_POINT ( 'NONE',  ( -2.992550472303094455, -137.9200387812562667, 0.9708280758990516235 ) ) ;
#6127=DIRECTION ( 'NONE',  ( -2.797435172181479917E-17, 1.000000000000000000, -1.765856845898779112E-18 ) ) ;
#6129=VERTEX_POINT ( 'NONE', #5792 ) ;
#6133=CARTESIAN_POINT ( 'NONE',  ( 1.718945942447514764E-16, -6.144721277337255927, 1.085069813372578838E-17 ) ) ;
#6136=CARTESIAN_POINT ( 'NONE',  ( -5.865056423939742913, -109.1014366316559290, 2.931634662963101157 ) ) ;
#6137=EDGE_CURVE ( 'NONE', #430, #1472, #8562, .T. ) ;
#6139=FACE_OUTER_BOUND ( 'NONE', #9682, .T. ) ;
#6140=DIRECTION ( 'NONE',  ( 0.4545454545454531425, 0.8907235428302472391, 0.000000000000000000 ) ) ;
#6144=CARTESIAN_POINT ( 'NONE',  ( 15.29705854078138927, 29.09759144140119957, 3.746698755667522411E-15 ) ) ;
#6145=CIRCLE ( 'NONE', #558, 24.99999999999998934 ) ;
#6147=AXIS2_PLACEMENT_3D ( 'NONE', #10830, #10899, #7752 ) ;
#6148=ORIENTED_EDGE ( 'NONE', *, *, #99, .F. ) ;
#6149=CARTESIAN_POINT ( 'NONE',  ( 15.29705854078140348, -29.33764382806072746, 1.923489752901241150E-15 ) ) ;
#6150=CARTESIAN_POINT ( 'NONE',  ( -4.242345193642410806, -72.18181818157590612, -0.3889582016414882548 ) ) ;
#6158=CARTESIAN_POINT ( 'NONE',  ( -3.784192700541099352, -60.99999999999985789, -1.982393907671068822 ) ) ;
#6166=AXIS2_PLACEMENT_3D ( 'NONE', #10411, #4020, #5210 ) ;
#6167=CARTESIAN_POINT ( 'NONE',  ( -7.205014192377404036, -85.42868670995821390, 6.118711583836721424 ) ) ;
#6173=AXIS2_PLACEMENT_3D ( 'NONE', #13884, #959, #3186 ) ;
#6175=CARTESIAN_POINT ( 'NONE',  ( 0.7725026565705566117, -151.5832121717045311, 1.650885043546370001 ) ) ;
#6176=ADVANCED_FACE ( 'NONE', ( #3230 ), #12403, .T. ) ;
#6177=DIRECTION ( 'NONE',  ( -1.000000000000000000, 0.000000000000000000, -0.000000000000000000 ) ) ;
#6180=ORIENTED_EDGE ( 'NONE', *, *, #11890, .F. ) ;
#6182=FACE_OUTER_BOUND ( 'NONE', #2585, .T. ) ;
#6188=ORIENTED_EDGE ( 'NONE', *, *, #2950, .F. ) ;
#6189=FACE_OUTER_BOUND ( 'NONE', #12860, .T. ) ;
#6190=CARTESIAN_POINT ( 'NONE',  ( -9.844122869686341204, -91.60173160181895469, -1.011447867193920658 ) ) ;
#6192=CIRCLE ( 'NONE', #146, 2.000000000000003997 ) ;
#6196=CARTESIAN_POINT ( 'NONE',  ( 4.861079856844285452, -110.7705047426206306, -4.116395442951102268 ) ) ;
#6197=CARTESIAN_POINT ( 'NONE',  ( -9.115242551282449313, -73.26725378407866174, -4.373789832702658309 ) ) ;
#6200=ORIENTED_EDGE ( 'NONE', *, *, #11349, .T. ) ;
#6201=ORIENTED_EDGE ( 'NONE', *, *, #4372, .F. ) ;
#6207=CARTESIAN_POINT ( 'NONE',  ( 3.178328602730291941, -98.49082012759913596, 7.173849163080390667 ) ) ;
#6208=CARTESIAN_POINT ( 'NONE',  ( 0.5048931899926654143, -158.0606060600380829, 1.721373026807350604 ) ) ;
#6209=DIRECTION ( 'NONE',  ( -0.8907235428302473501, -0.4545454545454531425, 0.000000000000000000 ) ) ;
#6210=CARTESIAN_POINT ( 'NONE',  ( -10.69346802281033959, 21.32451227372186864, -21.38693604562068984 ) ) ;
#6211=CARTESIAN_POINT ( 'NONE',  ( -32.72727272727271952, 135.1423002281142089, -2.500000000000000000 ) ) ;
#6212=EDGE_CURVE ( 'NONE', #13265, #4522, #3367, .T. ) ;
#6215=LINE ( 'NONE', #879, #12380 ) ;
#6216=EDGE_CURVE ( 'NONE', #13042, #7777, #5672, .T. ) ;
#6217=EDGE_LOOP ( 'NONE', ( #5919, #4489, #12888, #8746 ) ) ;
#6220=CARTESIAN_POINT ( 'NONE',  ( -4.246087656249755149, -68.90909090942406579, 1.771789674518133184 ) ) ;
#6225=CARTESIAN_POINT ( 'NONE',  ( 10.82460162405762460, -71.99999999999998579, 2.658570984654982539 ) ) ;
#6226=CARTESIAN_POINT ( 'NONE',  ( 1.916816365364574892, -124.8181818181859057, 4.196942880910825124 ) ) ;
#6228=CARTESIAN_POINT ( 'NONE',  ( -10.69346802281035025, 49.59884612375012125, -1.484741062544533711E-15 ) ) ;
#6229=LINE ( 'NONE', #8255, #5902 ) ;
#6230=CARTESIAN_POINT ( 'NONE',  ( 8.385254915620292238, 50.40394642271930792, 9.355740606675297531E-16 ) ) ;
#6233=CARTESIAN_POINT ( 'NONE',  ( 8.385254915620294014, -12.94488700934118341, 1.052073721316228892E-15 ) ) ;
#6234=CARTESIAN_POINT ( 'NONE',  ( 12.99553232110413781, 67.62342244460847951, 3.182987412051231379E-15 ) ) ;
#6235=CARTESIAN_POINT ( 'NONE',  ( 10.69346802281035025, 30.74929022373127196, -21.38693604562068984 ) ) ;
#6237=CARTESIAN_POINT ( 'NONE',  ( 1.055520991492275407, -150.0189090233429567, 1.640041038016263331 ) ) ;
#6238=VECTOR ( 'NONE', #1764, 1000.000000000000000 ) ;
#6241=VERTEX_POINT ( 'NONE', #11856 ) ;
#6244=FACE_OUTER_BOUND ( 'NONE', #8092, .T. ) ;
#6246=ORIENTED_EDGE ( 'NONE', *, *, #802, .T. ) ;
#6248=CARTESIAN_POINT ( 'NONE',  ( -10.69346802281035202, 77.87317997377837742, -2.801244458071077041E-15 ) ) ;
#6249=EDGE_LOOP ( 'NONE', ( #1265, #6415, #4530, #7921 ) ) ;
#6251=CARTESIAN_POINT ( 'NONE',  ( -8.385254915620292238, 43.60378069071538221, -1.180893628524435759E-15 ) ) ;
#6252=LINE ( 'NONE', #3087, #13715 ) ;
#6254=CARTESIAN_POINT ( 'NONE',  ( -1.392812481782718104, -130.7247055227911972, 3.705400635335541537 ) ) ;
#6258=CARTESIAN_POINT ( 'NONE',  ( 0.8861126034330837342, -145.6297630941380987, -2.175407028858133085 ) ) ;
#6259=CARTESIAN_POINT ( 'NONE',  ( -2.517691654963332357E-15, 90.00000000000000000, -1.589271161308885878E-16 ) ) ;
#6260=EDGE_CURVE ( 'NONE', #4145, #3627, #9262, .T. ) ;
#6261=CARTESIAN_POINT ( 'NONE',  ( 15.29705854078137861, 38.52236939141059935, 30.59411708156277498 ) ) ;
#6263=FACE_OUTER_BOUND ( 'NONE', #10320, .T. ) ;
#6264=CARTESIAN_POINT ( 'NONE',  ( -4.736736781129390117, -106.7560981827712965, 4.922394428301823943 ) ) ;
#6265=AXIS2_PLACEMENT_3D ( 'NONE', #7313, #12522, #6140 ) ;
#6266=CARTESIAN_POINT ( 'NONE',  ( -32.72727272727271952, 135.1423002281142089, 0.5000000000000000000 ) ) ;
#6268=DIRECTION ( 'NONE',  ( -2.797435172181481150E-17, 1.000000000000000000, -1.765856845898762549E-18 ) ) ;
#6269=EDGE_CURVE ( 'NONE', #9012, #3902, #9933, .T. ) ;
#6270=CARTESIAN_POINT ( 'NONE',  ( 15.29705854078139637, 0.8232575913729167638, 1.873561326908939829E-15 ) ) ;
#6271=AXIS2_PLACEMENT_3D ( 'NONE', #244, #3445, #5484 ) ;
#6272=DIRECTION ( 'NONE',  ( 0.8000000000000008216, 0.5999999999999988676, -4.163336342344329138E-15 ) ) ;
#6274=DIRECTION ( 'NONE',  ( 1.000000000000000000, 0.000000000000000000, 0.000000000000000000 ) ) ;
#6275=CARTESIAN_POINT ( 'NONE',  ( -8.385254915620294014, 12.70483462268159869, -2.243491919447391838E-17 ) ) ;
#6278=CARTESIAN_POINT ( 'NONE',  ( -11.42080557900780668, -157.8181818179944855, 3.873507862836679916 ) ) ;
#6280=ORIENTED_EDGE ( 'NONE', *, *, #11827, .T. ) ;
#6282=CARTESIAN_POINT ( 'NONE',  ( -12.99579180576517246, -11.31471392308272428, 25.99158361153033070 ) ) ;
#6284=CARTESIAN_POINT ( 'NONE',  ( -8.385254915620295790, 90.00000000000000000, -1.589271161308885878E-16 ) ) ;
#6287=CARTESIAN_POINT ( 'NONE',  ( 12.87330105402722680, -111.7272727272711705, -6.772701765862029433 ) ) ;
#6288=ADVANCED_FACE ( 'NONE', ( #1622 ), #13224, .T. ) ;
#6289=CARTESIAN_POINT ( 'NONE',  ( 0.6173387890061909911, 90.00000000000000000, -4.961742921553712549 ) ) ;
#6290=CARTESIAN_POINT ( 'NONE',  ( 8.385254915620290461, 50.40394642271930081, 16.77050983124059158 ) ) ;
#6292=CARTESIAN_POINT ( 'NONE',  ( -2.504065471750553911E-13, 90.00000000000000000, -3.100119530583082101E-14 ) ) ;
#6293=CARTESIAN_POINT ( 'NONE',  ( -11.81226048336476886, -40.00941361824966691, -1.305282905288380184E-15 ) ) ;
#6294=ORIENTED_EDGE ( 'NONE', *, *, #11295, .T. ) ;
#6295=CIRCLE ( 'NONE', #258, 2.000000000000007105 ) ;
#6297=CARTESIAN_POINT ( 'NONE',  ( -8.842511989038502662, -90.40394009946363951, -0.01791039437029070397 ) ) ;
#6301=FACE_OUTER_BOUND ( 'NONE', #4767, .T. ) ;
#6302=CARTESIAN_POINT ( 'NONE',  ( -36.36363636363635976, 142.2680885707561629, -0.5000000000000000000 ) ) ;
#6307=CARTESIAN_POINT ( 'NONE',  ( 4.330127018922191873, 90.00000000000000000, 0.5000000000000000000 ) ) ;
#6310=CARTESIAN_POINT ( 'NONE',  ( -2.010743657263654653E-15, 71.87811454074363837, -1.269264606320675724E-16 ) ) ;
#6313=CARTESIAN_POINT ( 'NONE',  ( 8.627629343136117512, -71.90909090909211443, 5.462837922541618596 ) ) ;
#6316=DIRECTION ( 'NONE',  ( -1.000000000000000000, 0.000000000000000000, 0.000000000000000000 ) ) ;
#6317=CARTESIAN_POINT ( 'NONE',  ( -10.35394582475455394, -72.00000000000014211, -3.762420212848085033 ) ) ;
#6319=CARTESIAN_POINT ( 'NONE',  ( 10.69346802281034492, 68.44840202376897764, 1.228280763400934348E-15 ) ) ;
#6320=CARTESIAN_POINT ( 'NONE',  ( -0.3211315587227348556, -154.7330882371165046, -1.606866635973652757 ) ) ;
#6321=CARTESIAN_POINT ( 'NONE',  ( 1.958204620527036497E-15, -70.00000000000000000, 1.236099792129133461E-16 ) ) ;
#6322=VERTEX_POINT ( 'NONE', #12287 ) ;
#6323=EDGE_CURVE ( 'NONE', #10942, #10921, #7090, .T. ) ;
#6325=VERTEX_POINT ( 'NONE', #2678 ) ;
#6329=VERTEX_POINT ( 'NONE', #11163 ) ;
#6331=CARTESIAN_POINT ( 'NONE',  ( -5.217808995651798121, -115.4128671718531223, -2.475508680495110525 ) ) ;
#6333=DIRECTION ( 'NONE',  ( 0.9923485843107423543, 2.797833471351478217E-17, 0.1234677578012386562 ) ) ;
#6334=CARTESIAN_POINT ( 'NONE',  ( 10.69381717166375267, 63.25855867215299355, 1.228320867585964984E-15 ) ) ;
#6335=CARTESIAN_POINT ( 'NONE',  ( 12.99553232110414491, 20.49953269456136695, -25.99106464220827561 ) ) ;
#6337=EDGE_CURVE ( 'NONE', #4279, #2222, #8292, .T. ) ;
#6339=CARTESIAN_POINT ( 'NONE',  ( 10.69346802281034492, 68.44840202376897764, 0.000000000000000000 ) ) ;
#6345=CARTESIAN_POINT ( 'NONE',  ( 2.318285725469618086, -147.1038961039384674, 4.595794441991605694 ) ) ;
#6346=ORIENTED_EDGE ( 'NONE', *, *, #1161, .T. ) ;
#6348=ORIENTED_EDGE ( 'NONE', *, *, #5490, .T. ) ;
#6349=DIRECTION ( 'NONE',  ( -0.000000000000000000, -0.000000000000000000, -1.000000000000000000 ) ) ;
#6351=CARTESIAN_POINT ( 'NONE',  ( 12.88103206736702511, -118.2727272727294121, 6.757986543075767294 ) ) ;
#6352=DIRECTION ( 'NONE',  ( 1.000000000000000000, -0.000000000000000000, 0.000000000000000000 ) ) ;
#6356=EDGE_CURVE ( 'NONE', #12845, #357, #5444, .T. ) ;
#6360=EDGE_CURVE ( 'NONE', #1890, #1745, #13582, .T. ) ;
#6365=CYLINDRICAL_SURFACE ( 'NONE', #7409, 15.29705854078139105 ) ;
#6367=CARTESIAN_POINT ( 'NONE',  ( -15.29705854078139105, 29.09759144140119957, -3.799746640842329186E-15 ) ) ;
#6369=CARTESIAN_POINT ( 'NONE',  ( 1.819477288719722585, -146.4205547847951152, 1.378398102139016368 ) ) ;
#6371=FACE_OUTER_BOUND ( 'NONE', #10804, .T. ) ;
#6372=ORIENTED_EDGE ( 'NONE', *, *, #5341, .F. ) ;
#6373=ORIENTED_EDGE ( 'NONE', *, *, #1444, .T. ) ;
#6374=ORIENTED_EDGE ( 'NONE', *, *, #43, .F. ) ;
#6375=EDGE_CURVE ( 'NONE', #6810, #2418, #724, .T. ) ;
#6377=CIRCLE ( 'NONE', #11539, 15.29705854078139282 ) ;
#6378=CYLINDRICAL_SURFACE ( 'NONE', #5023, 8.385254915620292238 ) ;
#6380=CARTESIAN_POINT ( 'NONE',  ( 4.840675591955164059, -75.54545454545383620, 8.982239580829949332 ) ) ;
#6385=FACE_OUTER_BOUND ( 'NONE', #4397, .T. ) ;
#6386=CARTESIAN_POINT ( 'NONE',  ( -2.504065471750553911E-13, 90.00000000000000000, -3.100119530583082101E-14 ) ) ;
#6388=CARTESIAN_POINT ( 'NONE',  ( 4.535930497296239317, -119.9429431484441722, 2.586521195913217053 ) ) ;
#6389=DIRECTION ( 'NONE',  ( -1.000000000000000000, 0.000000000000000000, 0.000000000000000000 ) ) ;
#6398=AXIS2_PLACEMENT_3D ( 'NONE', #12275, #6932, #6653 ) ;
#6400=CARTESIAN_POINT ( 'NONE',  ( -3.621723652282179629, -105.2179775488178137, 6.003010775146917943 ) ) ;
#6402=FACE_OUTER_BOUND ( 'NONE', #4423, .T. ) ;
#6404=DIRECTION ( 'NONE',  ( -2.797435172181481150E-17, 1.000000000000000000, -1.765856845898762549E-18 ) ) ;
#6406=CARTESIAN_POINT ( 'NONE',  ( -6.726204760714091790, -75.54545454545716154, -7.481082188384119647 ) ) ;
#6409=ORIENTED_EDGE ( 'NONE', *, *, #1814, .F. ) ;
#6415=ORIENTED_EDGE ( 'NONE', *, *, #2599, .T. ) ;
#6416=CARTESIAN_POINT ( 'NONE',  ( -2.517691654963332357E-15, 90.00000000000000000, -1.589271161308885878E-16 ) ) ;
#6417=ORIENTED_EDGE ( 'NONE', *, *, #13664, .F. ) ;
#6421=AXIS2_PLACEMENT_3D ( 'NONE', #5029, #9310, #12745 ) ;
#6422=CARTESIAN_POINT ( 'NONE',  ( -4.364119526982408459, -68.90909090871591047, -1.457038019223346526 ) ) ;
#6425=CARTESIAN_POINT ( 'NONE',  ( 38.79999999999999716, 101.5999999999999943, 2.500000000000000000 ) ) ;
#6427=FACE_OUTER_BOUND ( 'NONE', #983, .T. ) ;
#6433=EDGE_CURVE ( 'NONE', #11415, #5518, #4000, .T. ) ;
#6436=EDGE_CURVE ( 'NONE', #1633, #13463, #1114, .T. ) ;
#6437=CARTESIAN_POINT ( 'NONE',  ( -9.876538000534836215, -71.62961015872004111, -2.126563546433114738 ) ) ;
#6438=EDGE_CURVE ( 'NONE', #6908, #8462, #11639, .T. ) ;
#6439=CARTESIAN_POINT ( 'NONE',  ( 0.000000000000000000, 71.01020514433645303, -2.500000000000000000 ) ) ;
#6440=DIRECTION ( 'NONE',  ( -1.000000000000000000, 0.000000000000000000, 0.000000000000000000 ) ) ;
#6441=VERTEX_POINT ( 'NONE', #4135 ) ;
#6444=ADVANCED_FACE ( 'NONE', ( #6189 ), #7157, .T. ) ;
#6446=DIRECTION ( 'NONE',  ( -1.000000000000000000, 0.000000000000000000, 0.000000000000000000 ) ) ;
#6447=ORIENTED_EDGE ( 'NONE', *, *, #2410, .T. ) ;
#6450=CARTESIAN_POINT ( 'NONE',  ( -2.255225165641619345, -77.73185736634954424, -9.851628698357723479 ) ) ;
#6454=CARTESIAN_POINT ( 'NONE',  ( -6.633121150698165991, -97.20333181108198062, -4.463170841960692137 ) ) ;
#6458=EDGE_LOOP ( 'NONE', ( #11269, #13201 ) ) ;
#6459=AXIS2_PLACEMENT_3D ( 'NONE', #6109, #10376, #9328 ) ;
#6460=TOROIDAL_SURFACE ( 'NONE', #9595, 42.00000000000001421, 2.000000000000000000 ) ;
#6461=DIRECTION ( 'NONE',  ( -2.797435172181481150E-17, 1.000000000000000000, -1.765856845898762549E-18 ) ) ;
#6462=LINE ( 'NONE', #166, #9192 ) ;
#6465=CARTESIAN_POINT ( 'NONE',  ( 12.99553232110413958, 39.34908859458022334, -25.99106464220826851 ) ) ;
#6469=CARTESIAN_POINT ( 'NONE',  ( -9.860966656292097454, -69.99999999999948841, -1.730751479146293903 ) ) ;
#6470=EDGE_CURVE ( 'NONE', #3638, #13779, #5784, .T. ) ;
#6471=CARTESIAN_POINT ( 'NONE',  ( 2.680497156733089970, -80.99999999999992895, -9.800765866881897992 ) ) ;
#6473=CARTESIAN_POINT ( 'NONE',  ( -8.385254915620295790, -15.56949922734665748, 16.77050983124058448 ) ) ;
#6483=VERTEX_POINT ( 'NONE', #12710 ) ;
#6485=ORIENTED_EDGE ( 'NONE', *, *, #2691, .T. ) ;
#6487=AXIS2_PLACEMENT_3D ( 'NONE', #11253, #8854, #4724 ) ;
#6488=CARTESIAN_POINT ( 'NONE',  ( -15.29705854078139815, 0.8232575913729157646, 30.59411708156277854 ) ) ;
#6489=CARTESIAN_POINT ( 'NONE',  ( 15.29705854078139282, 74.33491362204294717, 1.740418857596141236E-15 ) ) ;
#6491=FACE_OUTER_BOUND ( 'NONE', #7383, .T. ) ;
#6495=CARTESIAN_POINT ( 'NONE',  ( 15.29705854078138749, 17.78624592198638155, 3.746698755667521623E-15 ) ) ;
#6496=CIRCLE ( 'NONE', #1575, 8.385254915620294014 ) ;
#6498=CIRCLE ( 'NONE', #12571, 2.000000000000003109 ) ;
#6499=EDGE_LOOP ( 'NONE', ( #5721, #9937, #70, #9960, #13512 ) ) ;
#6500=AXIS2_PLACEMENT_3D ( 'NONE', #9253, #710, #13774 ) ;
#6503=CARTESIAN_POINT ( 'NONE',  ( -12.99553232110414314, 67.62342244460847951, 25.99106464220826496 ) ) ;
#6504=CIRCLE ( 'NONE', #5845, 15.29705854078138749 ) ;
#6505=CARTESIAN_POINT ( 'NONE',  ( 0.000000000000000000, 71.01020514433645303, 0.5000000000000000000 ) ) ;
#6506=DIRECTION ( 'NONE',  ( -0.000000000000000000, -0.000000000000000000, -1.000000000000000000 ) ) ;
#6508=CARTESIAN_POINT ( 'NONE',  ( 15.29705854078138749, 10.24803554138234496, 3.746698755667521623E-15 ) ) ;
#6512=EDGE_CURVE ( 'NONE', #11768, #11894, #103, .T. ) ;
#6513=CIRCLE ( 'NONE', #8313, 15.29705854078139637 ) ;
#6516=ORIENTED_EDGE ( 'NONE', *, *, #13419, .T. ) ;
#6518=ORIENTED_EDGE ( 'NONE', *, *, #8155, .F. ) ;
#6521=CARTESIAN_POINT ( 'NONE',  ( -3.108119021657300696, -77.10324913307979955, -9.630131037565234919 ) ) ;
#6524=CARTESIAN_POINT ( 'NONE',  ( 4.230699918504775781, 91.18539124371000071, -2.666380740812164696 ) ) ;
#6525=CARTESIAN_POINT ( 'NONE',  ( 1.140958104747115343, -80.62156175248728118, 9.984774867419227817 ) ) ;
#6527=ORIENTED_EDGE ( 'NONE', *, *, #211, .F. ) ;
#6529=EDGE_CURVE ( 'NONE', #11270, #9012, #384, .T. ) ;
#6534=CARTESIAN_POINT ( 'NONE',  ( 15.29705854078138927, 29.09759144140119957, 1.823632900916640086E-15 ) ) ;
#6536=ORIENTED_EDGE ( 'NONE', *, *, #11349, .F. ) ;
#6538=CARTESIAN_POINT ( 'NONE',  ( -10.69346802281034137, 59.02362407375952102, -21.38693604562068984 ) ) ;
#6539=CARTESIAN_POINT ( 'NONE',  ( 10.69381717166375623, 6.709890972096427042, 1.299272810468638199E-15 ) ) ;
#6540=CARTESIAN_POINT ( 'NONE',  ( -39.99999999999999289, 100.0000000000000000, -0.5000000000000000000 ) ) ;
#6541=CARTESIAN_POINT ( 'NONE',  ( -0.3668613529521884686, -160.9696969702431488, 1.703459722496312612 ) ) ;
#6542=CARTESIAN_POINT ( 'NONE',  ( -9.807291687911792621, -69.33333333333621340, -2.012068907120004635 ) ) ;
#6543=CARTESIAN_POINT ( 'NONE',  ( 10.69346802281034314, -16.37459952631584059, 21.38693604562069694 ) ) ;
#6544=CARTESIAN_POINT ( 'NONE',  ( -2.517691654963332357E-15, 90.00000000000000000, -1.589271161308885878E-16 ) ) ;
#6545=VERTEX_POINT ( 'NONE', #11165 ) ;
#6549=EDGE_CURVE ( 'NONE', #297, #13779, #5689, .T. ) ;
#6550=DIRECTION ( 'NONE',  ( 1.000000000000000000, 0.000000000000000000, 0.000000000000000000 ) ) ;
#6551=DIRECTION ( 'NONE',  ( -1.000000000000000000, 0.000000000000000000, 0.000000000000000000 ) ) ;
#6553=CIRCLE ( 'NONE', #1404, 1.999999999999998890 ) ;
#6554=CARTESIAN_POINT ( 'NONE',  ( 8.385254915620292238, -12.94488700934118341, 1.052073721316228694E-15 ) ) ;
#6556=CARTESIAN_POINT ( 'NONE',  ( -10.69381717166375623, 72.68333662216238622, -1.566311632108520979E-15 ) ) ;
#6557=CARTESIAN_POINT ( 'NONE',  ( -12.99579180576516535, 54.65873172698324112, -25.99158361153033425 ) ) ;
#6560=CARTESIAN_POINT ( 'NONE',  ( 15.29705854078138749, 10.24803554138234496, 1.856918518244839783E-15 ) ) ;
#6561=CARTESIAN_POINT ( 'NONE',  ( 12.99579180576517423, -20.73949187309215247, 0.000000000000000000 ) ) ;
#6562=CARTESIAN_POINT ( 'NONE',  ( -2.517691654963332357E-15, 90.00000000000000000, -1.589271161308885878E-16 ) ) ;
#6565=EDGE_LOOP ( 'NONE', ( #5904, #8896, #5184, #12859, #523, #13500, #5174, #12286, #4861 ) ) ;
#6569=DIRECTION ( 'NONE',  ( -1.000000000000000000, 0.000000000000000000, 0.000000000000000000 ) ) ;
#6571=CARTESIAN_POINT ( 'NONE',  ( -0.6173387890061953209, 79.99058638175036151, 4.961742921553712549 ) ) ;
#6573=ORIENTED_EDGE ( 'NONE', *, *, #6438, .T. ) ;
#6574=ORIENTED_EDGE ( 'NONE', *, *, #4372, .T. ) ;
#6575=AXIS2_PLACEMENT_3D ( 'NONE', #12470, #2854, #9309 ) ;
#6577=VERTEX_POINT ( 'NONE', #2537 ) ;
#6581=DIRECTION ( 'NONE',  ( 1.000000000000000000, 0.000000000000000000, 0.000000000000000000 ) ) ;
#6584=CARTESIAN_POINT ( 'NONE',  ( -2.434338757227561434, -101.9345656283768022, -7.012440599860332746 ) ) ;
#6585=CARTESIAN_POINT ( 'NONE',  ( -10.00000000000000711, 139.9999999999999716, -2.500000000000000000 ) ) ;
#6591=CIRCLE ( 'NONE', #580, 22.99999999999999645 ) ;
#6593=ORIENTED_EDGE ( 'NONE', *, *, #1914, .F. ) ;
#6596=CARTESIAN_POINT ( 'NONE',  ( -8.385254915620290461, 59.82872437272870769, -16.77050983124058448 ) ) ;
#6601=CARTESIAN_POINT ( 'NONE',  ( -0.6121604151423207796, -166.5454546257185768, -9.081467143786552398 ) ) ;
#6602=EDGE_CURVE ( 'NONE', #1315, #10942, #7247, .T. ) ;
#6603=CARTESIAN_POINT ( 'NONE',  ( -3.385241169372517955, -79.21212121212087709, -9.605957155564929906 ) ) ;
#6616=ORIENTED_EDGE ( 'NONE', *, *, #12552, .T. ) ;
#6619=CARTESIAN_POINT ( 'NONE',  ( -1.219787497442949287E-15, 43.60378069071538221, -7.699803463976802609E-17 ) ) ;
#6620=FACE_OUTER_BOUND ( 'NONE', #732, .T. ) ;
#6623=( BOUNDED_SURFACE ( )  B_SPLINE_SURFACE ( 3, 3, ( 
 ( #9391, #2868, #11352, #2016 ),
 ( #5105, #12691, #974, #3068 ),
 ( #7142, #11419, #3982, #9521 ),
 ( #6233, #10571, #6031, #11559 ) ),
 .UNSPECIFIED., .F., .F., .T. ) 
 B_SPLINE_SURFACE_WITH_KNOTS ( ( 4, 4 ),
 ( 4, 4 ),
 ( 0.000000000000000000, 1.000000000000000000 ),
 ( 0.000000000000000000, 1.000000000000000000 ),
 .UNSPECIFIED. ) 
 GEOMETRIC_REPRESENTATION_ITEM ( )  RATIONAL_B_SPLINE_SURFACE ( (
 ( 1.000000000000000000, 0.3333333333333334259, 0.3333333333333334259, 1.000000000000000000),
 ( 1.000000000000000000, 0.3333333333333334259, 0.3333333333333334259, 1.000000000000000000),
 ( 1.000000000000000000, 0.3333333333333334259, 0.3333333333333334259, 1.000000000000000000),
 ( 1.000000000000000000, 0.3333333333333334259, 0.3333333333333334259, 1.000000000000000000) ) ) 
 REPRESENTATION_ITEM ( '' )  SURFACE ( )  );
#6624=CARTESIAN_POINT ( 'NONE',  ( 15.29705854078138749, 90.00000000000000000, 1.714422261702872371E-15 ) ) ;
#6626=CARTESIAN_POINT ( 'NONE',  ( -12.99579180576517423, -30.16426982310158067, -1.484993918994249462E-15 ) ) ;
#6627=AXIS2_PLACEMENT_3D ( 'NONE', #11424, #9580, #3193 ) ;
#6628=EDGE_CURVE ( 'NONE', #6322, #6577, #525, .T. ) ;
#6629=CARTESIAN_POINT ( 'NONE',  ( -2.517691654963332357E-15, 90.00000000000000000, -1.589271161308885878E-16 ) ) ;
#6630=CARTESIAN_POINT ( 'NONE',  ( 12.99579180576516357, 16.95961992694555676, 3.183050967463141802E-15 ) ) ;
#6632=ORIENTED_EDGE ( 'NONE', *, *, #3340, .T. ) ;
#6637=ORIENTED_EDGE ( 'NONE', *, *, #6216, .F. ) ;
#6639=CARTESIAN_POINT ( 'NONE',  ( -10.69381717166375800, 53.83378072214353693, -1.499740397452121781E-15 ) ) ;
#6640=LINE ( 'NONE', #10981, #3639 ) ;
#6643=ORIENTED_EDGE ( 'NONE', *, *, #6360, .T. ) ;
#6644=EDGE_CURVE ( 'NONE', #8513, #4067, #11963, .T. ) ;
#6647=ORIENTED_EDGE ( 'NONE', *, *, #9619, .T. ) ;
#6648=FACE_OUTER_BOUND ( 'NONE', #7117, .T. ) ;
#6649=ORIENTED_EDGE ( 'NONE', *, *, #6098, .F. ) ;
#6650=CARTESIAN_POINT ( 'NONE',  ( -8.385254915620292238, 71.87811454074363837, -1.280750480509034654E-15 ) ) ;
#6653=DIRECTION ( 'NONE',  ( 1.000000000000000000, 0.000000000000000000, 0.000000000000000000 ) ) ;
#6654=CARTESIAN_POINT ( 'NONE',  ( 2.766098618134335663, 90.01525736159537416, -4.178197917109232051 ) ) ;
#6655=CARTESIAN_POINT ( 'NONE',  ( -7.746655750637584603, -88.96548976718894153, 4.603499224255631184 ) ) ;
#6658=ORIENTED_EDGE ( 'NONE', *, *, #1654, .T. ) ;
#6660=CARTESIAN_POINT ( 'NONE',  ( -4.066030946031339077, 90.77438413795603367, 2.912544222229247470 ) ) ;
#6663=CARTESIAN_POINT ( 'NONE',  ( -12.99579180576517068, 35.80917582696438473, 25.99158361153032359 ) ) ;
#6664=CARTESIAN_POINT ( 'NONE',  ( 15.29705854078139282, 8.361467971976955127, -30.59411708156277498 ) ) ;
#6667=CARTESIAN_POINT ( 'NONE',  ( 10.69381717166375445, 44.40900277213413716, 0.000000000000000000 ) ) ;
#6668=DIRECTION ( 'NONE',  ( -0.4545454545454558626, 0.8907235428302457958, 0.000000000000000000 ) ) ;
#6671=ORIENTED_EDGE ( 'NONE', *, *, #13131, .F. ) ;
#6676=ORIENTED_EDGE ( 'NONE', *, *, #5736, .T. ) ;
#6679=FACE_OUTER_BOUND ( 'NONE', #12268, .T. ) ;
#6681=ADVANCED_FACE ( 'NONE', ( #9524 ), #1449, .T. ) ;
#6684=CARTESIAN_POINT ( 'NONE',  ( -15.29705854078139105, 8.361467971976981772, -1.476515546007874940E-17 ) ) ;
#6686=CARTESIAN_POINT ( 'NONE',  ( -8.385254915620292238, 71.87811454074363837, -1.269264606320675724E-16 ) ) ;
#6687=AXIS2_PLACEMENT_3D ( 'NONE', #10761, #11685, #12960 ) ;
#6688=FACE_OUTER_BOUND ( 'NONE', #3994, .T. ) ;
#6689=CARTESIAN_POINT ( 'NONE',  ( -10.69381717166375623, 44.40900277213413716, -2.718044847157924077E-15 ) ) ;
#6691=DIRECTION ( 'NONE',  ( -1.000000000000000000, 0.000000000000000000, 0.000000000000000000 ) ) ;
#6694=DIRECTION ( 'NONE',  ( -1.000000000000000000, 0.000000000000000000, 0.000000000000000000 ) ) ;
#6704=CARTESIAN_POINT ( 'NONE',  ( 10.69346802281034670, 49.59884612375012125, 0.000000000000000000 ) ) ;
#6705=ORIENTED_EDGE ( 'NONE', *, *, #8673, .F. ) ;
#6707=CIRCLE ( 'NONE', #5362, 5.000000000000000000 ) ;
#6708=EDGE_CURVE ( 'NONE', #10788, #11146, #11495, .T. ) ;
#6709=CARTESIAN_POINT ( 'NONE',  ( 25.00000000000000355, 120.0000000000000284, -2.500000000000000000 ) ) ;
#6714=ORIENTED_EDGE ( 'NONE', *, *, #2669, .F. ) ;
#6725=DIRECTION ( 'NONE',  ( 0.000000000000000000, 0.000000000000000000, 1.000000000000000000 ) ) ;
#6728=CARTESIAN_POINT ( 'NONE',  ( -8.308237197123997220, -90.29822314243337189, 3.067701055007814759 ) ) ;
#6730=AXIS2_PLACEMENT_3D ( 'NONE', #1128, #10845, #10777 ) ;
#6732=EDGE_LOOP ( 'NONE', ( #5990, #7051, #285, #8116, #487, #1936 ) ) ;
#6736=ORIENTED_EDGE ( 'NONE', *, *, #12391, .F. ) ;
#6737=CARTESIAN_POINT ( 'NONE',  ( -8.385254915620294014, -3.520109059331755663, 16.77050983124058092 ) ) ;
#6738=( NAMED_UNIT ( * ) PLANE_ANGLE_UNIT ( ) SI_UNIT ( $, .RADIAN. ) );
#6739=CARTESIAN_POINT ( 'NONE',  ( -10.69346802281034670, 59.02362407375952102, -2.757941663132658262E-15 ) ) ;
#6742=CIRCLE ( 'NONE', #5173, 14.99999999999999112 ) ;
#6743=CARTESIAN_POINT ( 'NONE',  ( 3.341303593453228693, -106.9090909090940187, -6.231874970757119492 ) ) ;
#6744=CARTESIAN_POINT ( 'NONE',  ( 10.00000000000000000, 90.00000000000000000, -0.5000000000000000000 ) ) ;
#6748=CARTESIAN_POINT ( 'NONE',  ( -8.385254915620292238, 34.17900274070598243, -6.035522597566817733E-17 ) ) ;
#6750=ORIENTED_EDGE ( 'NONE', *, *, #2223, .T. ) ;
#6755=LINE ( 'NONE', #11023, #7607 ) ;
#6756=DIRECTION ( 'NONE',  ( -1.000000000000000000, 0.000000000000000000, 0.000000000000000000 ) ) ;
#6761=CARTESIAN_POINT ( 'NONE',  ( 4.696430422119469483, 90.40949893945196436, -1.719416569030751685 ) ) ;
#6762=CARTESIAN_POINT ( 'NONE',  ( 15.29705854078138749, 17.78624592198638155, 1.840275709580739737E-15 ) ) ;
#6767=DIRECTION ( 'NONE',  ( -0.1234677578012386562, -1.701584941912606716E-18, 0.9923485843107423543 ) ) ;
#6773=CARTESIAN_POINT ( 'NONE',  ( 3.828914887500465269, 90.45818551217382719, 3.218881588266133686 ) ) ;
#6774=ORIENTED_EDGE ( 'NONE', *, *, #9671, .T. ) ;
#6775=CARTESIAN_POINT ( 'NONE',  ( -15.29705854078139105, 47.94714734142005597, -8.466779837416320124E-17 ) ) ;
#6777=DIRECTION ( 'NONE',  ( -2.797435172181481150E-17, 1.000000000000000000, -1.765856845898762549E-18 ) ) ;
#6779=VERTEX_POINT ( 'NONE', #6302 ) ;
#6782=CIRCLE ( 'NONE', #11488, 15.29705854078139460 ) ;
#6786=CARTESIAN_POINT ( 'NONE',  ( 10.07809618175545552, -70.83793457269361227, 0.9291402596207405384 ) ) ;
#6788=ORIENTED_EDGE ( 'NONE', *, *, #10887, .T. ) ;
#6793=DIRECTION ( 'NONE',  ( 1.000000000000000000, 0.000000000000000000, 0.000000000000000000 ) ) ;
#6794=ORIENTED_EDGE ( 'NONE', *, *, #6644, .T. ) ;
#6795=VERTEX_POINT ( 'NONE', #4678 ) ;
#6802=CARTESIAN_POINT ( 'NONE',  ( 15.29705854078138927, 66.79670324143890525, -30.59411708156276788 ) ) ;
#6803=CARTESIAN_POINT ( 'NONE',  ( -8.385254915620294014, -31.79444290936001138, -1.999968028543267754E-15 ) ) ;
#6808=FACE_OUTER_BOUND ( 'NONE', #9540, .T. ) ;
#6809=CARTESIAN_POINT ( 'NONE',  ( -0.2617580721752758022, -80.12121212121192571, 10.03731802028323727 ) ) ;
#6810=VERTEX_POINT ( 'NONE', #13272 ) ;
#6816=CARTESIAN_POINT ( 'NONE',  ( 10.69346802281035202, -16.37459952631584059, -21.38693604562069339 ) ) ;
#6817=CARTESIAN_POINT ( 'NONE',  ( 6.635975953253233861, -85.78354978353411298, -7.919939413331956501 ) ) ;
#6818=DIRECTION ( 'NONE',  ( -0.000000000000000000, -0.000000000000000000, -1.000000000000000000 ) ) ;
#6824=EDGE_LOOP ( 'NONE', ( #4395, #9407, #200, #3443 ) ) ;
#6826=CIRCLE ( 'NONE', #6166, 8.385254915620292238 ) ;
#6828=CARTESIAN_POINT ( 'NONE',  ( -1.339511369751129832, -125.0784420352225368, 4.454679473787292565 ) ) ;
#6834=ORIENTED_EDGE ( 'NONE', *, *, #9279, .T. ) ;
#6835=LINE ( 'NONE', #11877, #4584 ) ;
#6837=CARTESIAN_POINT ( 'NONE',  ( 32.72727272727274084, 135.1423002281142089, 2.500000000000000000 ) ) ;
#6841=CARTESIAN_POINT ( 'NONE',  ( -10.69346802281034847, 68.44840202376897764, -1.551312297200932909E-15 ) ) ;
#6844=DIRECTION ( 'NONE',  ( -1.000000000000000000, 0.000000000000000000, 0.000000000000000000 ) ) ;
#6845=CARTESIAN_POINT ( 'NONE',  ( 12.99553232110414491, -7.774801155466914970, 1.605812573171299022E-15 ) ) ;
#6847=ORIENTED_EDGE ( 'NONE', *, *, #9699, .T. ) ;
#6849=CARTESIAN_POINT ( 'NONE',  ( 3.784192700541063825, -168.9999999999998010, 1.982393907671174960 ) ) ;
#6852=ORIENTED_EDGE ( 'NONE', *, *, #8185, .T. ) ;
#6853=CARTESIAN_POINT ( 'NONE',  ( 12.99553232110413958, 48.77386654458962312, 0.000000000000000000 ) ) ;
#6854=VERTEX_POINT ( 'NONE', #2507 ) ;
#6855=AXIS2_PLACEMENT_3D ( 'NONE', #6386, #2168, #8551 ) ;
#6856=CARTESIAN_POINT ( 'NONE',  ( -15.29705854078138749, 36.63580182200524149, -30.59411708156277854 ) ) ;
#6860=CARTESIAN_POINT ( 'NONE',  ( -12.99553232110414314, 20.49953269456136695, -1.663892186318449368E-15 ) ) ;
#6862=CARTESIAN_POINT ( 'NONE',  ( -15.29705854078139282, -38.76242177807012723, 30.59411708156277854 ) ) ;
#6866=CARTESIAN_POINT ( 'NONE',  ( -15.29705854078138927, -27.45107625865536960, -30.59411708156278564 ) ) ;
#6867=EDGE_CURVE ( 'NONE', #11197, #6577, #111, .T. ) ;
#6869=ORIENTED_EDGE ( 'NONE', *, *, #6899, .F. ) ;
#6870=EDGE_CURVE ( 'NONE', #8621, #2743, #1894, .T. ) ;
#6871=DIRECTION ( 'NONE',  ( 2.797435172181480534E-17, -1.000000000000000000, 1.765856845898762164E-18 ) ) ;
#6872=ADVANCED_FACE ( 'NONE', ( #5440 ), #2330, .T. ) ;
#6873=CIRCLE ( 'NONE', #10235, 11.81226048336476886 ) ;
#6874=CARTESIAN_POINT ( 'NONE',  ( -10.69346802281035202, 77.87317997377837742, -1.584597914529132607E-15 ) ) ;
#6877=CARTESIAN_POINT ( 'NONE',  ( 2.209461285238361494, -83.12085171535194661, -9.413399924858527612 ) ) ;
#6880=ORIENTED_EDGE ( 'NONE', *, *, #8589, .F. ) ;
#6882=CARTESIAN_POINT ( 'NONE',  ( -2.680497156732949637, -80.99999999999998579, 9.800765866881983257 ) ) ;
#6884=CARTESIAN_POINT ( 'NONE',  ( 6.850226906711063712, -73.90543882657019026, 7.468286908571726279 ) ) ;
#6888=CARTESIAN_POINT ( 'NONE',  ( -1.174765158626910777, -79.03030303034420001, -10.44010582246512264 ) ) ;
#6893=CARTESIAN_POINT ( 'NONE',  ( 1.896508640845344207, -103.2776239719436120, -7.000734796588814035 ) ) ;
#6895=CARTESIAN_POINT ( 'NONE',  ( -4.975586992323414874E-16, 17.78624592198638155, -3.140796412417860432E-17 ) ) ;
#6898=CARTESIAN_POINT ( 'NONE',  ( -1.759686353460360175, -152.7490567289512171, -0.2786442552020600982 ) ) ;
#6899=EDGE_CURVE ( 'NONE', #575, #10661, #10186, .T. ) ;
#6901=DIRECTION ( 'NONE',  ( -2.797435172181481150E-17, 1.000000000000000000, -1.765856845898762549E-18 ) ) ;
#6903=CARTESIAN_POINT ( 'NONE',  ( 0.6173387890061953209, -69.99999999999998579, -4.961742921553712549 ) ) ;
#6905=CARTESIAN_POINT ( 'NONE',  ( 15.29705854078139460, -27.45107625865536605, 1.923489752901240361E-15 ) ) ;
#6906=AXIS2_PLACEMENT_3D ( 'NONE', #9344, #13654, #7227 ) ;
#6908=VERTEX_POINT ( 'NONE', #4451 ) ;
#6911=CARTESIAN_POINT ( 'NONE',  ( 11.72298137502698623, -169.0000000000001137, 2.970135970081305921 ) ) ;
#6913=VERTEX_POINT ( 'NONE', #2287 ) ;
#6916=CARTESIAN_POINT ( 'NONE',  ( 10.91573825926023922, -140.5584415584475835, 8.453432789889285814 ) ) ;
#6917=CARTESIAN_POINT ( 'NONE',  ( 50.00000000000000000, 120.0000000000000284, 0.5000000000000000000 ) ) ;
#6918=CARTESIAN_POINT ( 'NONE',  ( 15.29705854078139282, -19.91286587805129926, 30.59411708156279630 ) ) ;
#6921=CARTESIAN_POINT ( 'NONE',  ( -12.97449437267217576, -39.59556244224027211, -1.449077110393148750E-15 ) ) ;
#6924=FACE_OUTER_BOUND ( 'NONE', #13574, .T. ) ;
#6927=ORIENTED_EDGE ( 'NONE', *, *, #6356, .T. ) ;
#6928=CARTESIAN_POINT ( 'NONE',  ( -8.385254915620294014, -24.99427717735608212, 4.413631546192547049E-17 ) ) ;
#6929=AXIS2_PLACEMENT_3D ( 'NONE', #680, #5878, #4819 ) ;
#6932=DIRECTION ( 'NONE',  ( -0.000000000000000000, -0.000000000000000000, -1.000000000000000000 ) ) ;
#6933=CARTESIAN_POINT ( 'NONE',  ( -4.832052475181153106, -110.7096548574291575, 4.160198837937846505 ) ) ;
#6935=EDGE_CURVE ( 'NONE', #6241, #13463, #3643, .T. ) ;
#6936=ORIENTED_EDGE ( 'NONE', *, *, #10643, .F. ) ;
#6939=ORIENTED_EDGE ( 'NONE', *, *, #6549, .F. ) ;
#6941=EDGE_CURVE ( 'NONE', #149, #1460, #12495, .T. ) ;
#6942=CIRCLE ( 'NONE', #12768, 8.385254915620292238 ) ;
#6944=CARTESIAN_POINT ( 'NONE',  ( -8.385254915620294014, -24.99427717735608212, -9.386249283210493447E-16 ) ) ;
#6945=DIRECTION ( 'NONE',  ( -1.000000000000000000, 0.000000000000000000, 0.000000000000000000 ) ) ;
#6947=CARTESIAN_POINT ( 'NONE',  ( 4.974937185533097050, 90.00000000000000000, 0.5000000000000000000 ) ) ;
#6948=SHAPE_REPRESENTATION_RELATIONSHIP ( 'NONE' , 'NONE' ,  #1365, #7406 ) ;
#6952=CARTESIAN_POINT ( 'NONE',  ( -15.29705854078139282, -1.063309978032473291, 1.877653204021102445E-18 ) ) ;
#6953=CARTESIAN_POINT ( 'NONE',  ( -2.491129965232259824, -148.3982683983499271, 1.520867222960083032 ) ) ;
#6955=CARTESIAN_POINT ( 'NONE',  ( 48.00000000000000000, 120.0000000000000284, 2.500000000000000000 ) ) ;
#6956=EDGE_CURVE ( 'NONE', #3001, #2418, #5926, .T. ) ;
#6957=AXIS2_PLACEMENT_3D ( 'NONE', #1286, #9706, #2555 ) ;
#6959=EDGE_CURVE ( 'NONE', #7666, #849, #1208, .T. ) ;
#6960=CYLINDRICAL_SURFACE ( 'NONE', #11977, 8.385254915620292238 ) ;
#6962=EDGE_LOOP ( 'NONE', ( #3510, #8158, #3788, #3670 ) ) ;
#6964=DIRECTION ( 'NONE',  ( -2.797435172181481150E-17, 1.000000000000000000, -1.765856845898762549E-18 ) ) ;
#6965=EDGE_LOOP ( 'NONE', ( #6714, #7030, #8667, #6658 ) ) ;
#6968=CARTESIAN_POINT ( 'NONE',  ( 4.479841886641914961, -106.3258580997496239, -5.265075680640510569 ) ) ;
#6970=CIRCLE ( 'NONE', #9878, 48.00000000000001421 ) ;
#6978=CARTESIAN_POINT ( 'NONE',  ( -1.495153876773553492, -154.2876702219585070, -0.7369765331111527429 ) ) ;
#6979=CARTESIAN_POINT ( 'NONE',  ( 4.545390705139091381, 90.76307318580400363, -2.092381513276356575 ) ) ;
#6982=CARTESIAN_POINT ( 'NONE',  ( 8.385254915620295790, -6.144721277337255927, 1.035430912652129043E-15 ) ) ;
#6985=DIRECTION ( 'NONE',  ( -0.9923485843107423543, -2.797833471351478217E-17, -0.1234677578012386562 ) ) ;
#6987=AXIS2_PLACEMENT_3D ( 'NONE', #9087, #3675, #12521 ) ;
#6988=EDGE_CURVE ( 'NONE', #11311, #9709, #4802, .T. ) ;
#6990=CARTESIAN_POINT ( 'NONE',  ( 10.69381717166375800, 53.83378072214353693, -21.38763434332750890 ) ) ;
#6991=CARTESIAN_POINT ( 'NONE',  ( 6.139211203634872049, -76.35064935069615899, 12.15884065890582555 ) ) ;
#6992=ORIENTED_EDGE ( 'NONE', *, *, #3718, .F. ) ;
#6993=ORIENTED_EDGE ( 'NONE', *, *, #10858, .T. ) ;
#6999=CARTESIAN_POINT ( 'NONE',  ( 10.69346802281034314, -35.22415542633469698, 21.38693604562069339 ) ) ;
#7000=VERTEX_POINT ( 'NONE', #13628 ) ;
#7002=ORIENTED_EDGE ( 'NONE', *, *, #13430, .F. ) ;
#7004=CARTESIAN_POINT ( 'NONE',  ( -15.29705854078138927, -36.87585420866476227, -3.723114491148376223E-15 ) ) ;
#7008=CARTESIAN_POINT ( 'NONE',  ( -1.483439550716517611E-15, 53.02855864072483882, -9.364084330386787485E-17 ) ) ;
#7009=CARTESIAN_POINT ( 'NONE',  ( 7.333588550536464190, -88.25569648369631182, -5.386745576991591733 ) ) ;
#7011=CARTESIAN_POINT ( 'NONE',  ( -10.69381717166375090, 16.13466892210585257, -21.38763434332751245 ) ) ;
#7012=ORIENTED_EDGE ( 'NONE', *, *, #8487, .F. ) ;
#7014=ORIENTED_EDGE ( 'NONE', *, *, #26, .F. ) ;
#7016=ADVANCED_FACE ( 'NONE', ( #1520 ), #11841, .T. ) ;
#7018=AXIS2_PLACEMENT_3D ( 'NONE', #12999, #2251, #5615 ) ;
#7019=CARTESIAN_POINT ( 'NONE',  ( 10.13852281052238702, -69.87878787878717901, -0.9720347947262335531 ) ) ;
#7021=CARTESIAN_POINT ( 'NONE',  ( 9.357262991920059392, -70.83714848844999779, 3.840749680622386641 ) ) ;
#7022=TOROIDAL_SURFACE ( 'NONE', #11048, 42.00000000000001421, 2.000000000000000000 ) ;
#7024=CARTESIAN_POINT ( 'NONE',  ( 3.510313888878266120, -133.0909090909286476, -1.034921094667353270 ) ) ;
#7026=CYLINDRICAL_SURFACE ( 'NONE', #4209, 8.385254915620295790 ) ;
#7030=ORIENTED_EDGE ( 'NONE', *, *, #4440, .F. ) ;
#7031=DIRECTION ( 'NONE',  ( 1.000000000000000000, 0.000000000000000000, 0.000000000000000000 ) ) ;
#7034=CARTESIAN_POINT ( 'NONE',  ( -3.251529939683060366, -129.1726566844749016, 2.555676826061363816 ) ) ;
#7037=ADVANCED_FACE ( 'NONE', ( #13420 ), #2159, .F. ) ;
#7041=CARTESIAN_POINT ( 'NONE',  ( 2.376601423472834540, -126.9250422869104540, -3.721977556539412202 ) ) ;
#7046=ADVANCED_FACE ( 'NONE', ( #7598, #408 ), #7806, .F. ) ;
#7047=CARTESIAN_POINT ( 'NONE',  ( 10.00000000000000000, 90.00000000000000000, -0.5000000000000000000 ) ) ;
#7049=CARTESIAN_POINT ( 'NONE',  ( -10.69346802281035025, 49.59884612375012125, -1.484741062544533711E-15 ) ) ;
#7051=ORIENTED_EDGE ( 'NONE', *, *, #3542, .T. ) ;
#7052=CARTESIAN_POINT ( 'NONE',  ( 12.02287503512517297, -157.8181818181245433, -0.9430477860670277712 ) ) ;
#7053=ORIENTED_EDGE ( 'NONE', *, *, #3542, .F. ) ;
#7054=CIRCLE ( 'NONE', #1014, 8.385254915620292238 ) ;
#7056=DIRECTION ( 'NONE',  ( 2.797435172181480534E-17, -1.000000000000000000, 1.765856845898762164E-18 ) ) ;
#7057=CARTESIAN_POINT ( 'NONE',  ( 10.00000000000000000, 92.00000000000000000, 0.5000000000000000000 ) ) ;
#7058=CARTESIAN_POINT ( 'NONE',  ( 4.607646589139954507, -134.6363636363662408, 0.3820433400543247759 ) ) ;
#7062=VECTOR ( 'NONE', #8449, 1000.000000000000000 ) ;
#7063=CARTESIAN_POINT ( 'NONE',  ( 8.385254915620292238, 22.12961257269105531, 2.053795118489800399E-15 ) ) ;
#7066=AXIS2_PLACEMENT_3D ( 'NONE', #13388, #11098, #4644 ) ;
#7068=CARTESIAN_POINT ( 'NONE',  ( -8.872490591736925225, -90.06604609259215977, 0.4070912038452756398 ) ) ;
#7069=TOROIDAL_SURFACE ( 'NONE', #11985, 22.99999999999999289, 2.000000000000000000 ) ;
#7071=CARTESIAN_POINT ( 'NONE',  ( 8.385254915620288685, 43.60378069071538221, 9.522168693316292075E-16 ) ) ;
#7072=EDGE_LOOP ( 'NONE', ( #13411, #9945, #5550, #10257 ) ) ;
#7074=CIRCLE ( 'NONE', #9295, 24.99999999999998934 ) ;
#7076=CARTESIAN_POINT ( 'NONE',  ( -15.29705854078139282, 76.22148119144830503, 30.59411708156276788 ) ) ;
#7079=CARTESIAN_POINT ( 'NONE',  ( -5.469814954756211378, -117.2912297489314710, -0.9484627639890558237 ) ) ;
#7081=AXIS2_PLACEMENT_3D ( 'NONE', #4475, #156, #79 ) ;
#7083=ORIENTED_EDGE ( 'NONE', *, *, #776, .F. ) ;
#7087=AXIS2_PLACEMENT_3D ( 'NONE', #6505, #10769, #4454 ) ;
#7088=CARTESIAN_POINT ( 'NONE',  ( 9.536547895815731479, -71.90909090909467238, 3.228601540706608208 ) ) ;
#7089=ORIENTED_EDGE ( 'NONE', *, *, #8259, .F. ) ;
#7090=LINE ( 'NONE', #1479, #8142 ) ;
#7091=CARTESIAN_POINT ( 'NONE',  ( -0.8583871962692122271, -102.5454545454458355, -7.611802117353696495 ) ) ;
#7092=CARTESIAN_POINT ( 'NONE',  ( -15.29705854078139105, 76.22148119144830503, -1.345962243664627229E-16 ) ) ;
#7096=CARTESIAN_POINT ( 'NONE',  ( 0.1852016367012860043, -160.0000000000003126, -1.488522876466233713 ) ) ;
#7098=ORIENTED_EDGE ( 'NONE', *, *, #9361, .T. ) ;
#7099=ORIENTED_EDGE ( 'NONE', *, *, #8331, .T. ) ;
#7101=CARTESIAN_POINT ( 'NONE',  ( 1.958204620527036497E-15, -70.00000000000000000, 1.236099792129133461E-16 ) ) ;
#7102=ORIENTED_EDGE ( 'NONE', *, *, #3141, .F. ) ;
#7103=CARTESIAN_POINT ( 'NONE',  ( -2.887522863561023723, -136.7361086070154954, -1.558166837788810932 ) ) ;
#7104=CARTESIAN_POINT ( 'NONE',  ( 6.257768754720297677E-16, -22.36966495935058319, 3.950162600893091522E-17 ) ) ;
#7105=( BOUNDED_SURFACE ( )  B_SPLINE_SURFACE ( 3, 3, ( 
 ( #4058, #3072, #2946, #3986 ),
 ( #2805, #7278, #842, #8132 ),
 ( #773, #9465, #5108, #11624 ),
 ( #3922, #8269, #13569, #2021 ) ),
 .UNSPECIFIED., .F., .F., .T. ) 
 B_SPLINE_SURFACE_WITH_KNOTS ( ( 4, 4 ),
 ( 4, 4 ),
 ( 0.000000000000000000, 1.000000000000000000 ),
 ( 0.000000000000000000, 1.000000000000000000 ),
 .UNSPECIFIED. ) 
 GEOMETRIC_REPRESENTATION_ITEM ( )  RATIONAL_B_SPLINE_SURFACE ( (
 ( 1.000000000000000000, 0.3333333333333334259, 0.3333333333333334259, 1.000000000000000000),
 ( 1.000000000000000000, 0.3333333333333334259, 0.3333333333333334259, 1.000000000000000000),
 ( 1.000000000000000000, 0.3333333333333334259, 0.3333333333333334259, 1.000000000000000000),
 ( 1.000000000000000000, 0.3333333333333334259, 0.3333333333333334259, 1.000000000000000000) ) ) 
 REPRESENTATION_ITEM ( '' )  SURFACE ( )  );
#7108=DIRECTION ( 'NONE',  ( -2.797435172181481150E-17, 1.000000000000000000, -1.765856845898762549E-18 ) ) ;
#7109=CARTESIAN_POINT ( 'NONE',  ( -1.659392250802589341, -148.6675893744416896, 1.251955227480716193 ) ) ;
#7111=LINE ( 'NONE', #8169, #7373 ) ;
#7113=DIRECTION ( 'NONE',  ( -2.797435172181481150E-17, 1.000000000000000000, -1.765856845898762549E-18 ) ) ;
#7114=CARTESIAN_POINT ( 'NONE',  ( -12.99553232110414314, 48.77386654458962312, -1.763749038303048460E-15 ) ) ;
#7115=EDGE_CURVE ( 'NONE', #11396, #11894, #2699, .T. ) ;
#7116=EDGE_CURVE ( 'NONE', #2454, #283, #11955, .T. ) ;
#7117=EDGE_LOOP ( 'NONE', ( #6374, #1709, #1571, #12818 ) ) ;
#7126=DIRECTION ( 'NONE',  ( -2.797435172181481150E-17, 1.000000000000000000, -1.765856845898762549E-18 ) ) ;
#7127=DIRECTION ( 'NONE',  ( 1.000000000000000000, 0.000000000000000000, 0.000000000000000000 ) ) ;
#7128=CARTESIAN_POINT ( 'NONE',  ( 12.93801431150394521, -134.6363636363615797, -1.977757875720894898 ) ) ;
#7129=CARTESIAN_POINT ( 'NONE',  ( 25.00000000000000355, 120.0000000000000284, 0.5000000000000000000 ) ) ;
#7130=CARTESIAN_POINT ( 'NONE',  ( -10.69381717166375800, -21.56444287793185310, 21.38763434332750890 ) ) ;
#7131=CARTESIAN_POINT ( 'NONE',  ( 15.29705854078140348, -29.33764382806072746, 1.923489752901241150E-15 ) ) ;
#7132=EDGE_CURVE ( 'NONE', #11767, #13355, #3256, .T. ) ;
#7133=UNCERTAINTY_MEASURE_WITH_UNIT (LENGTH_MEASURE( 1.000000000000000082E-05 ), #2760, 'distance_accuracy_value', 'NONE');
#7134=CARTESIAN_POINT ( 'NONE',  ( -11.81226048336477064, -40.00941361824966691, 23.62452096672953061 ) ) ;
#7137=ORIENTED_EDGE ( 'NONE', *, *, #13115, .T. ) ;
#7142=CARTESIAN_POINT ( 'NONE',  ( 10.69381717166375800, -12.13966492792242846, 1.341722361464477482E-15 ) ) ;
#7143=CIRCLE ( 'NONE', #4220, 8.385254915620294014 ) ;
#7145=CARTESIAN_POINT ( 'NONE',  ( -0.1852015970780942489, -159.9999997928953235, 1.488522644435750886 ) ) ;
#7147=CARTESIAN_POINT ( 'NONE',  ( 6.692989812469433808, -97.14474235384638234, 4.437126219143910255 ) ) ;
#7148=EDGE_CURVE ( 'NONE', #6779, #6795, #2449, .T. ) ;
#7155=CARTESIAN_POINT ( 'NONE',  ( 14.13596196814457784, -39.17949320881311337, -28.27192393628913436 ) ) ;
#7157=CYLINDRICAL_SURFACE ( 'NONE', #978, 24.99999999999998934 ) ;
#7162=CARTESIAN_POINT ( 'NONE',  ( -1.375500123858559354, -148.4763468619591151, -1.574495689507027896 ) ) ;
#7163=DIRECTION ( 'NONE',  ( 0.000000000000000000, 0.000000000000000000, 1.000000000000000000 ) ) ;
#7165=CIRCLE ( 'NONE', #1125, 8.385254915620294014 ) ;
#7166=ORIENTED_EDGE ( 'NONE', *, *, #11337, .F. ) ;
#7168=CARTESIAN_POINT ( 'NONE',  ( -1.705970724789718451, -139.6653734298945722, -2.453391655664824089 ) ) ;
#7169=CARTESIAN_POINT ( 'NONE',  ( -12.99553232110413958, 39.34908859458022334, 25.99106464220826496 ) ) ;
#7171=CARTESIAN_POINT ( 'NONE',  ( 0.8657135605078067897, -80.00115760430779233, 9.969076801623804940 ) ) ;
#7173=DIRECTION ( 'NONE',  ( -2.797435172181481150E-17, 1.000000000000000000, -1.765856845898762549E-18 ) ) ;
#7176=LINE ( 'NONE', #10343, #6037 ) ;
#7177=CARTESIAN_POINT ( 'NONE',  ( -15.29705854078139637, 74.33491362204294717, -1.312648161087776599E-16 ) ) ;
#7178=CARTESIAN_POINT ( 'NONE',  ( 0.9875500501441598633, -80.00464164738322381, -10.06307372056550342 ) ) ;
#7182=CARTESIAN_POINT ( 'NONE',  ( 8.385254915620292238, 31.55439052270045508, 16.77050983124059513 ) ) ;
#7183=AXIS2_PLACEMENT_3D ( 'NONE', #12730, #6272, #5212 ) ;
#7184=( BOUNDED_SURFACE ( )  B_SPLINE_SURFACE ( 3, 3, ( 
 ( #11358, #8906, #10103, #4694 ),
 ( #2602, #9052, #2742, #9959 ),
 ( #514, #12355, #2808, #5680 ),
 ( #11078, #11153, #8002, #366 ) ),
 .UNSPECIFIED., .F., .F., .T. ) 
 B_SPLINE_SURFACE_WITH_KNOTS ( ( 4, 4 ),
 ( 4, 4 ),
 ( 0.000000000000000000, 1.000000000000000000 ),
 ( 0.000000000000000000, 1.000000000000000000 ),
 .UNSPECIFIED. ) 
 GEOMETRIC_REPRESENTATION_ITEM ( )  RATIONAL_B_SPLINE_SURFACE ( (
 ( 1.000000000000000000, 0.3333333333333334259, 0.3333333333333334259, 1.000000000000000000),
 ( 1.000000000000000000, 0.3333333333333334259, 0.3333333333333334259, 1.000000000000000000),
 ( 1.000000000000000000, 0.3333333333333334259, 0.3333333333333334259, 1.000000000000000000),
 ( 1.000000000000000000, 0.3333333333333334259, 0.3333333333333334259, 1.000000000000000000) ) ) 
 REPRESENTATION_ITEM ( '' )  SURFACE ( )  );
#7185=CARTESIAN_POINT ( 'NONE',  ( -10.00000000000000711, 139.9999999999999716, 0.5000000000000000000 ) ) ;
#7188=AXIS2_PLACEMENT_3D ( 'NONE', #7838, #9389, #12479 ) ;
#7191=CYLINDRICAL_SURFACE ( 'NONE', #8844, 15.29705854078139105 ) ;
#7193=CARTESIAN_POINT ( 'NONE',  ( -4.363680981163685857, 91.46147893603955481, -2.443653808501017544 ) ) ;
#7197=CARTESIAN_POINT ( 'NONE',  ( 4.154595973944828380, -61.00000000000013500, -0.9946518452611575745 ) ) ;
#7200=CARTESIAN_POINT ( 'NONE',  ( -15.29705854078139282, 47.94714734142005597, -2.042684974582087312E-15 ) ) ;
#7202=CARTESIAN_POINT ( 'NONE',  ( 10.69346802281034670, 77.87317997377837742, 0.000000000000000000 ) ) ;
#7203=AXIS2_PLACEMENT_3D ( 'NONE', #13616, #3965, #13679 ) ;
#7204=CARTESIAN_POINT ( 'NONE',  ( -3.918572219198208639, -82.19108314072666133, 8.951287372965479605 ) ) ;
#7207=CARTESIAN_POINT ( 'NONE',  ( -8.385254915620286909, -22.36966495935058319, -16.77050983124058092 ) ) ;
#7211=EDGE_CURVE ( 'NONE', #11499, #9709, #7111, .T. ) ;
#7214=CARTESIAN_POINT ( 'NONE',  ( 2.824482778608038647, -140.8717184737295440, 0.1012005756595079214 ) ) ;
#7215=CARTESIAN_POINT ( 'NONE',  ( 10.00000000000000711, 139.9999999999999716, 2.500000000000000000 ) ) ;
#7218=ORIENTED_EDGE ( 'NONE', *, *, #11733, .F. ) ;
#7220=ORIENTED_EDGE ( 'NONE', *, *, #13589, .T. ) ;
#7223=ORIENTED_EDGE ( 'NONE', *, *, #10268, .T. ) ;
#7224=FACE_OUTER_BOUND ( 'NONE', #11689, .T. ) ;
#7226=DIRECTION ( 'NONE',  ( -2.797435172181481150E-17, 1.000000000000000000, -1.765856845898762549E-18 ) ) ;
#7227=DIRECTION ( 'NONE',  ( -1.000000000000000000, 0.000000000000000000, 0.000000000000000000 ) ) ;
#7230=ADVANCED_FACE ( 'NONE', ( #5786 ), #2776, .T. ) ;
#7231=CARTESIAN_POINT ( 'NONE',  ( 15.29705854078139105, 27.21102387199583816, 1.823632900916640874E-15 ) ) ;
#7233=CARTESIAN_POINT ( 'NONE',  ( 5.702026264667728661, -116.1006108127829606, 0.07857520267129523839 ) ) ;
#7234=DIRECTION ( 'NONE',  ( -0.8000000000000008216, -0.5999999999999988676, 0.000000000000000000 ) ) ;
#7236=EDGE_LOOP ( 'NONE', ( #4862, #12346, #2013, #12919 ) ) ;
#7237=ORIENTED_EDGE ( 'NONE', *, *, #1948, .F. ) ;
#7241=DIRECTION ( 'NONE',  ( 1.000000000000000000, 4.625929269271489266E-15, 0.000000000000000000 ) ) ;
#7242=CARTESIAN_POINT ( 'NONE',  ( 6.017021975735540984, -95.62437285806116449, 5.547819245424533641 ) ) ;
#7243=CARTESIAN_POINT ( 'NONE',  ( -0.03865624730777729445, -158.0606060610036820, -1.868422726202614959 ) ) ;
#7245=DIRECTION ( 'NONE',  ( -1.000000000000000000, 0.000000000000000000, 0.000000000000000000 ) ) ;
#7247=CIRCLE ( 'NONE', #4797, 8.385254915620292238 ) ;
#7249=CARTESIAN_POINT ( 'NONE',  ( -2.517691654963332357E-15, 90.00000000000000000, -1.589271161308885878E-16 ) ) ;
#7253=CARTESIAN_POINT ( 'NONE',  ( 25.00000000000000355, 120.0000000000000284, -2.500000000000000000 ) ) ;
#7254=CARTESIAN_POINT ( 'NONE',  ( -3.606245374342868626, -157.8181818183407756, 2.267989313195203138 ) ) ;
#7256=CARTESIAN_POINT ( 'NONE',  ( -10.69381717166375800, -12.13966492792242846, 21.38763434332751245 ) ) ;
#7258=AXIS2_PLACEMENT_3D ( 'NONE', #13110, #5577, #341 ) ;
#7259=CARTESIAN_POINT ( 'NONE',  ( -4.330127018922195425, 92.00000000000000000, -2.500000000000000000 ) ) ;
#7260=CARTESIAN_POINT ( 'NONE',  ( -15.29705854078140170, -29.33764382806072746, 5.180607919632063331E-17 ) ) ;
#7262=CARTESIAN_POINT ( 'NONE',  ( -6.062451257354288359, -129.7272727272762154, 11.56901651898807160 ) ) ;
#7263=B_SPLINE_CURVE_WITH_KNOTS ( 'NONE', 3,
 ( #10888, #259, #1171, #8793 ),
 .UNSPECIFIED., .F., .F.,
 ( 4, 4 ),
 ( 0.000000000000000000, 1.000000000000000000 ),
 .UNSPECIFIED. ) ;
#7264=CARTESIAN_POINT ( 'NONE',  ( 8.385254915620292238, 59.82872437272870769, 9.189312520034297072E-16 ) ) ;
#7269=CIRCLE ( 'NONE', #5033, 15.29705854078139105 ) ;
#7270=EDGE_CURVE ( 'NONE', #10317, #4734, #4453, .T. ) ;
#7271=VERTEX_POINT ( 'NONE', #2839 ) ;
#7274=CARTESIAN_POINT ( 'NONE',  ( 15.29705854078140348, -19.91286587805129926, -30.59411708156278920 ) ) ;
#7275=CIRCLE ( 'NONE', #9964, 40.00000000000001421 ) ;
#7276=DIRECTION ( 'NONE',  ( -0.000000000000000000, -0.000000000000000000, -1.000000000000000000 ) ) ;
#7278=CARTESIAN_POINT ( 'NONE',  ( 12.99579180576517068, -1.889935973073298081, -25.99158361153033070 ) ) ;
#7279=FACE_OUTER_BOUND ( 'NONE', #13188, .T. ) ;
#7280=DIRECTION ( 'NONE',  ( -0.000000000000000000, -0.000000000000000000, -1.000000000000000000 ) ) ;
#7283=EDGE_LOOP ( 'NONE', ( #1105, #11294, #13573, #912 ) ) ;
#7286=CARTESIAN_POINT ( 'NONE',  ( -2.517691654963332357E-15, 90.00000000000000000, -1.589271161308885878E-16 ) ) ;
#7289=CIRCLE ( 'NONE', #4371, 2.000000000000003109 ) ;
#7293=CARTESIAN_POINT ( 'NONE',  ( 1.416598489609834699, -78.09090909090815558, 10.12631592825928273 ) ) ;
#7295=DIRECTION ( 'NONE',  ( -1.000000000000000000, 0.000000000000000000, -0.000000000000000000 ) ) ;
#7296=CARTESIAN_POINT ( 'NONE',  ( 4.974937185533097050, 90.00000000000000000, 0.5000000000000000000 ) ) ;
#7297=AXIS2_PLACEMENT_3D ( 'NONE', #9270, #10460, #13587 ) ;
#7300=CARTESIAN_POINT ( 'NONE',  ( -15.29705854078139460, -18.02629830864596627, 3.183186227453577089E-17 ) ) ;
#7301=CARTESIAN_POINT ( 'NONE',  ( 5.749669232646114736, -115.6779247526754091, -0.2475080363690762286 ) ) ;
#7304=ORIENTED_EDGE ( 'NONE', *, *, #5573, .F. ) ;
#7306=ADVANCED_FACE ( 'NONE', ( #12389 ), #11487, .T. ) ;
#7309=FACE_OUTER_BOUND ( 'NONE', #11802, .T. ) ;
#7310=CARTESIAN_POINT ( 'NONE',  ( 2.082709946752197006, -80.78332142495241897, -9.792949010885818595 ) ) ;
#7312=CARTESIAN_POINT ( 'NONE',  ( -15.29705854078139282, 46.06057977201469100, -8.133639011647813827E-17 ) ) ;
#7313=CARTESIAN_POINT ( 'NONE',  ( 35.45454545454547457, 140.4866414850956744, 0.5000000000000000000 ) ) ;
#7320=CARTESIAN_POINT ( 'NONE',  ( 1.133743435585240489, -129.7272727272670352, -4.472427317383721679 ) ) ;
#7322=ORIENTED_EDGE ( 'NONE', *, *, #4539, .T. ) ;
#7323=CARTESIAN_POINT ( 'NONE',  ( 8.385254915620294014, -12.94488700934118341, 2.053795118489800793E-15 ) ) ;
#7324=ORIENTED_EDGE ( 'NONE', *, *, #7477, .T. ) ;
#7327=CARTESIAN_POINT ( 'NONE',  ( 8.355259928129500580, -76.12121212035069107, 3.018973157362855986 ) ) ;
#7328=CARTESIAN_POINT ( 'NONE',  ( 11.42080557901028293, -157.8181818180634366, -3.873507862844141947 ) ) ;
#7331=DIRECTION ( 'NONE',  ( 2.797435172181480534E-17, -1.000000000000000000, 1.765856845898762164E-18 ) ) ;
#7333=ORIENTED_EDGE ( 'NONE', *, *, #11295, .F. ) ;
#7336=EDGE_CURVE ( 'NONE', #2480, #12324, #12992, .T. ) ;
#7338=CARTESIAN_POINT ( 'NONE',  ( -2.200973885217364349E-15, 78.67828027274755698, -1.389345798431728350E-16 ) ) ;
#7341=DIRECTION ( 'NONE',  ( -0.5999999999999989786, -0.8000000000000008216, 0.000000000000000000 ) ) ;
#7344=ORIENTED_EDGE ( 'NONE', *, *, #12547, .T. ) ;
#7346=VECTOR ( 'NONE', #349, 1000.000000000000000 ) ;
#7349=ORIENTED_EDGE ( 'NONE', *, *, #8743, .F. ) ;
#7352=CARTESIAN_POINT ( 'NONE',  ( -7.616846500253796393, -85.78354978338798276, 7.024694013272235971 ) ) ;
#7354=ADVANCED_FACE ( 'NONE', ( #12728 ), #7590, .T. ) ;
#7356=CARTESIAN_POINT ( 'NONE',  ( 10.69346802281034314, 21.32451227372186864, 0.000000000000000000 ) ) ;
#7359=CARTESIAN_POINT ( 'NONE',  ( -1.327769271380126570, -103.0493006173539641, -7.164857848410852270 ) ) ;
#7361=FACE_OUTER_BOUND ( 'NONE', #2693, .T. ) ;
#7362=ORIENTED_EDGE ( 'NONE', *, *, #13614, .F. ) ;
#7366=AXIS2_PLACEMENT_3D ( 'NONE', #4039, #2073, #6083 ) ;
#7369=EDGE_LOOP ( 'NONE', ( #1491, #11567, #11249, #10871 ) ) ;
#7370=DIRECTION ( 'NONE',  ( -0.000000000000000000, -0.000000000000000000, -1.000000000000000000 ) ) ;
#7371=CARTESIAN_POINT ( 'NONE',  ( -5.489740287354453407, -114.7850684598158892, -2.013460231478539253 ) ) ;
#7373=VECTOR ( 'NONE', #1718, 1000.000000000000000 ) ;
#7374=CARTESIAN_POINT ( 'NONE',  ( 11.81226048336477064, -40.00941361824963849, 0.000000000000000000 ) ) ;
#7376=CARTESIAN_POINT ( 'NONE',  ( 15.29705854078139282, 19.67281349139177138, -30.59411708156276788 ) ) ;
#7377=CARTESIAN_POINT ( 'NONE',  ( 8.385254915620294014, 3.280056672672171381, 1.027013741517443780E-15 ) ) ;
#7381=CARTESIAN_POINT ( 'NONE',  ( -15.29705854078139105, 29.09759144140119957, -1.976113739925688312E-15 ) ) ;
#7383=EDGE_LOOP ( 'NONE', ( #982, #11186, #7102, #9756 ) ) ;
#7387=CARTESIAN_POINT ( 'NONE',  ( 4.801896836370951327, -140.5584415584236240, 0.8531065430110326142 ) ) ;
#7391=DIRECTION ( 'NONE',  ( -0.000000000000000000, -0.000000000000000000, -1.000000000000000000 ) ) ;
#7392=ORIENTED_EDGE ( 'NONE', *, *, #2528, .F. ) ;
#7396=EDGE_CURVE ( 'NONE', #1501, #8022, #1324, .T. ) ;
#7397=CARTESIAN_POINT ( 'NONE',  ( 4.242345193634528222, -72.18181818161869501, 0.3889582016326292302 ) ) ;
#7400=CARTESIAN_POINT ( 'NONE',  ( -10.69381717166375267, 25.55944687211528787, -21.38763434332751601 ) ) ;
#7401=DIRECTION ( 'NONE',  ( -2.797435172181481150E-17, 1.000000000000000000, -1.765856845898762549E-18 ) ) ;
#7402=EDGE_CURVE ( 'NONE', #10681, #9187, #9841, .T. ) ;
#7404=CARTESIAN_POINT ( 'NONE',  ( 15.29705854078138216, 17.78624592198638155, 30.59411708156277498 ) ) ;
#7406=ADVANCED_BREP_SHAPE_REPRESENTATION ( '', ( #12476, #8193 ), #11552 ) ;
#7409=AXIS2_PLACEMENT_3D ( 'NONE', #2149, #7886, #10957 ) ;
#7413=CARTESIAN_POINT ( 'NONE',  ( -2.517691654963332357E-15, 90.00000000000000000, -1.589271161308885878E-16 ) ) ;
#7414=CARTESIAN_POINT ( 'NONE',  ( 10.69346802281034492, 68.44840202376897764, 2.619144277183853160E-15 ) ) ;
#7415=B_SPLINE_CURVE_WITH_KNOTS ( 'NONE', 3,
 ( #8535, #11034, #64, #3130 ),
 .UNSPECIFIED., .F., .F.,
 ( 4, 4 ),
 ( 0.000000000000000000, 1.000000000000000000 ),
 .UNSPECIFIED. ) ;
#7418=CARTESIAN_POINT ( 'NONE',  ( 2.385373235779478573, -133.5189184999073007, -2.750077259266392460 ) ) ;
#7420=EDGE_LOOP ( 'NONE', ( #3446, #8975, #1127, #7949 ) ) ;
#7425=VERTEX_POINT ( 'NONE', #873 ) ;
#7430=CARTESIAN_POINT ( 'NONE',  ( 25.00000000000000355, 120.0000000000000284, 0.5000000000000000000 ) ) ;
#7433=CARTESIAN_POINT ( 'NONE',  ( 0.7638352155348442363, -126.5711838444371296, 4.383014990228201846 ) ) ;
#7434=DIRECTION ( 'NONE',  ( -2.797435172181481150E-17, 1.000000000000000000, -1.765856845898762549E-18 ) ) ;
#7437=ADVANCED_FACE ( 'NONE', ( #13742 ), #5141, .T. ) ;
#7438=CARTESIAN_POINT ( 'NONE',  ( 8.385254915620294014, 40.97916847270985130, 2.053795118489800793E-15 ) ) ;
#7439=EDGE_LOOP ( 'NONE', ( #6852, #7705, #1166, #11822 ) ) ;
#7441=CARTESIAN_POINT ( 'NONE',  ( -1.444477056741696464, -121.1523416466594654, -4.889642476594785236 ) ) ;
#7442=FACE_OUTER_BOUND ( 'NONE', #9818, .T. ) ;
#7444=CARTESIAN_POINT ( 'NONE',  ( -2.966263562846015667, -142.5800865800325994, -0.5601050917294461140 ) ) ;
#7446=CIRCLE ( 'NONE', #2289, 8.385254915620290461 ) ;
#7448=CARTESIAN_POINT ( 'NONE',  ( -2.142312913383871198, -80.12121212121239466, -9.955895698471787014 ) ) ;
#7449=CARTESIAN_POINT ( 'NONE',  ( 1.119237408740483274E-15, -40.00941361824966691, 7.065089693818133469E-17 ) ) ;
#7455=EDGE_CURVE ( 'NONE', #5860, #11418, #13482, .T. ) ;
#7456=CARTESIAN_POINT ( 'NONE',  ( -57.42269783611796186, -167.3636363826522881, 5.376878112289413814 ) ) ;
#7460=DIRECTION ( 'NONE',  ( -2.797435172181481150E-17, 1.000000000000000000, -1.765856845898762549E-18 ) ) ;
#7461=EDGE_CURVE ( 'NONE', #7855, #283, #9905, .T. ) ;
#7465=DIRECTION ( 'NONE',  ( -1.000000000000000000, 0.000000000000000000, 0.000000000000000000 ) ) ;
#7466=CARTESIAN_POINT ( 'NONE',  ( 10.69381717166375623, 25.55944687211528077, 2.619229793989004345E-15 ) ) ;
#7469=CARTESIAN_POINT ( 'NONE',  ( 3.373786045844536563, -82.89610389618431441, -3.887588323741812957 ) ) ;
#7471=CARTESIAN_POINT ( 'NONE',  ( -12.99553232110413248, 11.07475474455194053, -25.99106464220827561 ) ) ;
#7473=DIRECTION ( 'NONE',  ( -2.797435172181481150E-17, 1.000000000000000000, -1.765856845898762549E-18 ) ) ;
#7475=VERTEX_POINT ( 'NONE', #4291 ) ;
#7477=EDGE_CURVE ( 'NONE', #1890, #5237, #6707, .T. ) ;
#7479=CYLINDRICAL_SURFACE ( 'NONE', #5875, 8.385254915620295790 ) ;
#7480=DIRECTION ( 'NONE',  ( 1.000000000000000000, 6.938893903907226405E-16, 0.000000000000000000 ) ) ;
#7481=CARTESIAN_POINT ( 'NONE',  ( -12.99579180576517068, 54.65873172698324112, -1.784564474948045950E-15 ) ) ;
#7483=CARTESIAN_POINT ( 'NONE',  ( -9.636121577330632348, -72.23759218051375797, -2.995460436795389647 ) ) ;
#7484=CARTESIAN_POINT ( 'NONE',  ( -2.517691654963332357E-15, 90.00000000000000000, -1.589271161308885878E-16 ) ) ;
#7489=ORIENTED_EDGE ( 'NONE', *, *, #7455, .T. ) ;
#7492=CARTESIAN_POINT ( 'NONE',  ( 7.679260624019852705E-16, -27.45107625865536605, 4.847467093863555185E-17 ) ) ;
#7493=AXIS2_PLACEMENT_3D ( 'NONE', #6001, #3672, #2630 ) ;
#7497=DIRECTION ( 'NONE',  ( -1.000000000000000000, 0.000000000000000000, 0.000000000000000000 ) ) ;
#7499=CARTESIAN_POINT ( 'NONE',  ( -6.370414618488270619, -97.56321138151314187, -4.760973744585681011 ) ) ;
#7500=DIRECTION ( 'NONE',  ( 0.000000000000000000, 0.000000000000000000, 1.000000000000000000 ) ) ;
#7501=ORIENTED_EDGE ( 'NONE', *, *, #1543, .F. ) ;
#7503=COLOUR_RGB ( '', 0.72549020, 0.75294118, 0.79215686) ;
#7507=ORIENTED_EDGE ( 'NONE', *, *, #6529, .F. ) ;
#7508=CARTESIAN_POINT ( 'NONE',  ( 15.29705854078138749, -1.063309978032445091, 30.59411708156277854 ) ) ;
#7509=AXIS2_PLACEMENT_3D ( 'NONE', #8979, #6725, #5600 ) ;
#7510=DIRECTION ( 'NONE',  ( 1.000000000000000000, 0.000000000000000000, 0.000000000000000000 ) ) ;
#7511=CARTESIAN_POINT ( 'NONE',  ( -4.184759487138673961, -117.2897403752749312, -3.654242507195469170 ) ) ;
#7513=CARTESIAN_POINT ( 'NONE',  ( -2.517691654963332357E-15, 90.00000000000000000, -1.589271161308885878E-16 ) ) ;
#7514=CARTESIAN_POINT ( 'NONE',  ( -2.517691654963332357E-15, 90.00000000000000000, -1.589271161308885878E-16 ) ) ;
#7516=CARTESIAN_POINT ( 'NONE',  ( -9.977514653935900313, -69.33333333333061432, -0.8249805266091697620 ) ) ;
#7517=EDGE_CURVE ( 'NONE', #3806, #9883, #9773, .T. ) ;
#7520=AXIS2_PLACEMENT_3D ( 'NONE', #7008, #3987, #2077 ) ;
#7521=FACE_OUTER_BOUND ( 'NONE', #9751, .T. ) ;
#7523=ORIENTED_EDGE ( 'NONE', *, *, #2379, .T. ) ;
#7527=EDGE_LOOP ( 'NONE', ( #10368, #2417, #12041, #10107 ) ) ;
#7528=CARTESIAN_POINT ( 'NONE',  ( 1.084353620409068652E-15, -38.76242177807012723, 6.844888786042043893E-17 ) ) ;
#7529=CARTESIAN_POINT ( 'NONE',  ( 12.99579180576516890, 26.38439787695498495, 3.183050967463142985E-15 ) ) ;
#7530=CARTESIAN_POINT ( 'NONE',  ( -8.385254915620297567, 90.00000000000000000, -1.589271161308885878E-16 ) ) ;
#7533=CARTESIAN_POINT ( 'NONE',  ( -15.29705854078138749, 27.21102387199583461, -30.59411708156277854 ) ) ;
#7534=EDGE_CURVE ( 'NONE', #11046, #10478, #9828, .T. ) ;
#7535=CARTESIAN_POINT ( 'NONE',  ( 15.29705854078140170, -19.91286587805129926, 1.906846944237140710E-15 ) ) ;
#7537=FACE_OUTER_BOUND ( 'NONE', #9390, .T. ) ;
#7539=ADVANCED_FACE ( 'NONE', ( #12073 ), #519, .F. ) ;
#7542=ORIENTED_EDGE ( 'NONE', *, *, #255, .T. ) ;
#7543=CARTESIAN_POINT ( 'NONE',  ( -12.99553232110413958, 67.62342244460847951, -1.830320272959447658E-15 ) ) ;
#7545=DIRECTION ( 'NONE',  ( 1.000000000000000000, 0.000000000000000000, 0.000000000000000000 ) ) ;
#7546=EDGE_CURVE ( 'NONE', #5181, #8931, #6252, .T. ) ;
#7548=CARTESIAN_POINT ( 'NONE',  ( 8.385254915620290461, 12.70483462268160046, 16.77050983124058803 ) ) ;
#7551=EDGE_CURVE ( 'NONE', #10942, #2744, #11614, .T. ) ;
#7553=EDGE_LOOP ( 'NONE', ( #6094, #8853, #7542, #12201 ) ) ;
#7555=CARTESIAN_POINT ( 'NONE',  ( 15.29705854078138927, 76.22148119144830503, -30.59411708156276788 ) ) ;
#7556=ORIENTED_EDGE ( 'NONE', *, *, #1889, .F. ) ;
#7560=CARTESIAN_POINT ( 'NONE',  ( -6.629834750586161896, -74.11811805074310655, -7.660853594987535153 ) ) ;
#7562=DIRECTION ( 'NONE',  ( -2.797435172181481150E-17, 1.000000000000000000, -1.765856845898762549E-18 ) ) ;
#7563=CARTESIAN_POINT ( 'NONE',  ( 3.159504973698678221, 90.09612598291144536, -3.878748273749980768 ) ) ;
#7564=CARTESIAN_POINT ( 'NONE',  ( -4.875680159242816281, -85.38011053856008914, 8.109980874214908653 ) ) ;
#7566=ORIENTED_EDGE ( 'NONE', *, *, #9224, .T. ) ;
#7570=AXIS2_PLACEMENT_3D ( 'NONE', #11344, #5032, #10295 ) ;
#7572=CARTESIAN_POINT ( 'NONE',  ( -8.385254915620294014, 90.00000000000000000, -1.589271161308885878E-16 ) ) ;
#7574=VERTEX_POINT ( 'NONE', #8482 ) ;
#7576=FILL_AREA_STYLE ('',( #7779 ) ) ;
#7578=CARTESIAN_POINT ( 'NONE',  ( -12.99579180576516535, 7.534841976936128560, -3.197093525192043264E-15 ) ) ;
#7579=CARTESIAN_POINT ( 'NONE',  ( -10.11144051725924520, -69.99977036137985920, 0.2534939247371171822 ) ) ;
#7580=CARTESIAN_POINT ( 'NONE',  ( -0.1425268984646445858, -158.0606060616233606, 0.6718241418580294111 ) ) ;
#7581=CARTESIAN_POINT ( 'NONE',  ( -8.804495088766199018, -73.18181818181871279, -4.925729831870038211 ) ) ;
#7583=DIRECTION ( 'NONE',  ( -2.797435172181481150E-17, 1.000000000000000000, -1.765856845898762549E-18 ) ) ;
#7584=FACE_OUTER_BOUND ( 'NONE', #5464, .T. ) ;
#7585=EDGE_LOOP ( 'NONE', ( #8628, #11741, #12983, #11286, #6676, #1957, #10133, #12297, #4036, #9076 ) ) ;
#7588=LINE ( 'NONE', #10875, #13032 ) ;
#7590=TOROIDAL_SURFACE ( 'NONE', #12321, 71.99999999999998579, 2.000000000000000000 ) ;
#7591=DIRECTION ( 'NONE',  ( 0.5999999999999989786, -0.8000000000000008216, 0.000000000000000000 ) ) ;
#7596=CIRCLE ( 'NONE', #2909, 16.99999999999998934 ) ;
#7597=CARTESIAN_POINT ( 'NONE',  ( -8.385254915620294014, 3.280056672672170937, -1.038481780305648437E-15 ) ) ;
#7598=FACE_BOUND ( 'NONE', #10447, .T. ) ;
#7599=CARTESIAN_POINT ( 'NONE',  ( -10.69381717166375623, -21.56444287793185666, -1.233455458826524398E-15 ) ) ;
#7604=CARTESIAN_POINT ( 'NONE',  ( 10.00000000000000711, 139.9999999999999716, -0.5000000000000000000 ) ) ;
#7607=VECTOR ( 'NONE', #1425, 1000.000000000000000 ) ;
#7611=TOROIDAL_SURFACE ( 'NONE', #2462, 22.99999999999999289, 2.000000000000000000 ) ;
#7613=DIRECTION ( 'NONE',  ( 1.000000000000000000, 9.637352644315596722E-16, 0.000000000000000000 ) ) ;
#7615=CARTESIAN_POINT ( 'NONE',  ( -8.385254915620292238, 53.02855864072483882, -1.214179245852635653E-15 ) ) ;
#7617=DIRECTION ( 'NONE',  ( -1.000000000000000000, 0.000000000000000000, 0.000000000000000000 ) ) ;
#7618=ORIENTED_EDGE ( 'NONE', *, *, #3497, .T. ) ;
#7620=EDGE_LOOP ( 'NONE', ( #9867, #920, #7322, #9129 ) ) ;
#7622=EDGE_LOOP ( 'NONE', ( #11114, #5535, #8003, #8944 ) ) ;
#7625=EDGE_CURVE ( 'NONE', #3627, #4145, #5589, .T. ) ;
#7629=ADVANCED_FACE ( 'NONE', ( #11578 ), #11205, .T. ) ;
#7630=FACE_OUTER_BOUND ( 'NONE', #6732, .T. ) ;
#7633=DIRECTION ( 'NONE',  ( 0.000000000000000000, 0.000000000000000000, 1.000000000000000000 ) ) ;
#7637=CARTESIAN_POINT ( 'NONE',  ( -7.144831932706865452, -87.96976810164353822, 5.694097463405904058 ) ) ;
#7640=ORIENTED_EDGE ( 'NONE', *, *, #1161, .F. ) ;
#7644=LINE ( 'NONE', #7572, #9831 ) ;
#7648=SURFACE_STYLE_USAGE ( .BOTH. , #13000 ) ;
#7649=CARTESIAN_POINT ( 'NONE',  ( 8.385254915620292238, 59.82872437272870769, 9.722760835075757558E-16 ) ) ;
#7650=EDGE_CURVE ( 'NONE', #10190, #297, #10745, .T. ) ;
#7651=CARTESIAN_POINT ( 'NONE',  ( 10.69381717166375800, 6.709890972096426154, -21.38763434332750890 ) ) ;
#7653=CARTESIAN_POINT ( 'NONE',  ( 8.385254915620292238, 90.00000000000000000, 8.679704431140114636E-16 ) ) ;
#7654=CARTESIAN_POINT ( 'NONE',  ( 8.385254915620288685, 43.60378069071538221, 9.522168693316292075E-16 ) ) ;
#7655=CARTESIAN_POINT ( 'NONE',  ( -2.010743657263654653E-15, 71.87811454074363837, -1.269264606320675724E-16 ) ) ;
#7658=DIRECTION ( 'NONE',  ( -2.797435172181481150E-17, 1.000000000000000000, -1.765856845898762549E-18 ) ) ;
#7660=ORIENTED_EDGE ( 'NONE', *, *, #7455, .F. ) ;
#7661=LINE ( 'NONE', #4573, #8609 ) ;
#7663=ORIENTED_EDGE ( 'NONE', *, *, #12190, .F. ) ;
#7665=CARTESIAN_POINT ( 'NONE',  ( -10.69381717166375623, 6.709890972096426154, -1.333312310811123490E-15 ) ) ;
#7666=VERTEX_POINT ( 'NONE', #5326 ) ;
#7668=DIRECTION ( 'NONE',  ( -2.797435172181481150E-17, 1.000000000000000000, -1.765856845898762549E-18 ) ) ;
#7671=CARTESIAN_POINT ( 'NONE',  ( 10.69381717166375800, 25.55944687211528787, -21.38763434332750890 ) ) ;
#7672=DIRECTION ( 'NONE',  ( -2.797435172181481150E-17, 1.000000000000000000, -1.765856845898762549E-18 ) ) ;
#7673=FACE_OUTER_BOUND ( 'NONE', #7620, .T. ) ;
#7674=CARTESIAN_POINT ( 'NONE',  ( -15.29705854078138927, 17.78624592198638155, -1.936165306082118094E-15 ) ) ;
#7678=CARTESIAN_POINT ( 'NONE',  ( 15.29705854078138749, 47.94714734142005597, 1.790347283588440388E-15 ) ) ;
#7681=CARTESIAN_POINT ( 'NONE',  ( -12.99579180576517068, 26.38439787695498495, -1.684707622963446858E-15 ) ) ;
#7684=EDGE_CURVE ( 'NONE', #6329, #7425, #8298, .T. ) ;
#7689=ORIENTED_EDGE ( 'NONE', *, *, #1948, .T. ) ;
#7691=ORIENTED_EDGE ( 'NONE', *, *, #7211, .T. ) ;
#7692=CARTESIAN_POINT ( 'NONE',  ( 1.958204620527036102E-15, -69.99999999999998579, 1.236099792129133461E-16 ) ) ;
#7694=CARTESIAN_POINT ( 'NONE',  ( -10.69381717166375800, 72.68333662216240043, 21.38763434332750535 ) ) ;
#7697=DIRECTION ( 'NONE',  ( 0.000000000000000000, -1.000000000000000000, 0.000000000000000000 ) ) ;
#7699=CARTESIAN_POINT ( 'NONE',  ( 2.482863863605449417, 90.00000000000002842, -4.353049703108322177 ) ) ;
#7701=CARTESIAN_POINT ( 'NONE',  ( 12.99579180576518134, -30.16426982310158422, -25.99158361153034491 ) ) ;
#7703=ADVANCED_FACE ( 'NONE', ( #6385 ), #7611, .T. ) ;
#7705=ORIENTED_EDGE ( 'NONE', *, *, #12778, .F. ) ;
#7707=EDGE_CURVE ( 'NONE', #6483, #9883, #12798, .T. ) ;
#7714=CARTESIAN_POINT ( 'NONE',  ( -15.29705854078139105, 8.361467971976955127, -3.761435144035948792E-15 ) ) ;
#7715=LINE ( 'NONE', #11997, #2051 ) ;
#7718=CARTESIAN_POINT ( 'NONE',  ( 15.29705854078138572, 90.00000000000000000, 1.714422261702872371E-15 ) ) ;
#7720=CARTESIAN_POINT ( 'NONE',  ( -15.29705854078139637, 90.00000000000000000, -1.589271161308885878E-16 ) ) ;
#7724=EDGE_CURVE ( 'NONE', #3535, #6779, #12051, .T. ) ;
#7729=FACE_OUTER_BOUND ( 'NONE', #12848, .T. ) ;
#7731=CARTESIAN_POINT ( 'NONE',  ( 12.99553232110414669, -17.19957910547634228, 0.000000000000000000 ) ) ;
#7732=ORIENTED_EDGE ( 'NONE', *, *, #9894, .T. ) ;
#7735=CARTESIAN_POINT ( 'NONE',  ( -8.385254915620295790, 24.75422479069652582, -1.114322393868036955E-15 ) ) ;
#7736=CARTESIAN_POINT ( 'NONE',  ( -8.385254915620286909, 43.60378069071538221, -16.77050983124057737 ) ) ;
#7737=DIRECTION ( 'NONE',  ( 1.000000000000000000, 0.000000000000000000, -0.000000000000000000 ) ) ;
#7738=CARTESIAN_POINT ( 'NONE',  ( 10.00000000000000000, 97.99999999999994316, -2.500000000000000000 ) ) ;
#7741=CARTESIAN_POINT ( 'NONE',  ( -8.385254915620297567, 78.67828027274755698, -1.389345798431728350E-16 ) ) ;
#7749=CYLINDRICAL_SURFACE ( 'NONE', #2563, 15.29705854078138749 ) ;
#7752=DIRECTION ( 'NONE',  ( -1.000000000000000000, 0.000000000000000000, 0.000000000000000000 ) ) ;
#7755=DIRECTION ( 'NONE',  ( -0.5999999999999989786, -0.8000000000000008216, 0.000000000000000000 ) ) ;
#7757=CARTESIAN_POINT ( 'NONE',  ( -8.385254915620294014, -24.99427717735608212, -2.007341458301378282E-15 ) ) ;
#7761=DIRECTION ( 'NONE',  ( -2.797435172181481150E-17, 1.000000000000000000, -1.765856845898762549E-18 ) ) ;
#7762=VERTEX_POINT ( 'NONE', #13435 ) ;
#7768=CARTESIAN_POINT ( 'NONE',  ( 10.69381717166376511, -30.98922082794128485, -21.38763434332751956 ) ) ;
#7772=CARTESIAN_POINT ( 'NONE',  ( 0.6173387890061948768, -40.00941361824966691, -4.961742921553712549 ) ) ;
#7774=CARTESIAN_POINT ( 'NONE',  ( -3.521437233922030785, 90.23421079890158580, 3.553194557407191922 ) ) ;
#7777=VERTEX_POINT ( 'NONE', #13128 ) ;
#7778=CARTESIAN_POINT ( 'NONE',  ( 8.385254915620292238, -3.520109059331755219, 2.053795118489800004E-15 ) ) ;
#7779=FILL_AREA_STYLE_COLOUR ( '', #7503 ) ;
#7780=AXIS2_PLACEMENT_3D ( 'NONE', #1317, #5598, #8753 ) ;
#7781=CARTESIAN_POINT ( 'NONE',  ( 0.1852016367020528076, -70.00000000000000000, -1.488522876466090272 ) ) ;
#7782=CARTESIAN_POINT ( 'NONE',  ( -2.557893175568157318, -128.7272727272848272, 3.337007314118914714 ) ) ;
#7783=DIRECTION ( 'NONE',  ( -0.000000000000000000, -0.000000000000000000, -1.000000000000000000 ) ) ;
#7784=EDGE_CURVE ( 'NONE', #8545, #8344, #6087, .T. ) ;
#7789=VECTOR ( 'NONE', #3137, 1000.000000000000000 ) ;
#7793=CARTESIAN_POINT ( 'NONE',  ( -2.339066459587731637E-16, 8.361467971976981772, -1.476515546007874940E-17 ) ) ;
#7795=CARTESIAN_POINT ( 'NONE',  ( -10.00000000000000711, 139.9999999999999716, -0.5000000000000000000 ) ) ;
#7806=PLANE ( 'NONE',  #2224 ) ;
#7808=VECTOR ( 'NONE', #3820, 1000.000000000000000 ) ;
#7813=CARTESIAN_POINT ( 'NONE',  ( -2.517691654963332357E-15, 90.00000000000000000, -1.589271161308885878E-16 ) ) ;
#7814=CARTESIAN_POINT ( 'NONE',  ( 8.385254915620299343, -6.144721277337255039, -16.77050983124059158 ) ) ;
#7815=EDGE_LOOP ( 'NONE', ( #9387, #8829, #11296, #6201 ) ) ;
#7816=DIRECTION ( 'NONE',  ( -1.000000000000000000, 0.000000000000000000, 0.000000000000000000 ) ) ;
#7821=ORIENTED_EDGE ( 'NONE', *, *, #7396, .T. ) ;
#7822=CARTESIAN_POINT ( 'NONE',  ( 9.628507540654561270E-16, -34.41905512736551032, 6.077912412602530076E-17 ) ) ;
#7823=ORIENTED_EDGE ( 'NONE', *, *, #8419, .T. ) ;
#7824=DIRECTION ( 'NONE',  ( -2.797435172181481150E-17, 1.000000000000000000, -1.765856845898762549E-18 ) ) ;
#7827=CARTESIAN_POINT ( 'NONE',  ( 8.894289287455980914E-16, -31.79444290936001138, 5.614443467303076398E-17 ) ) ;
#7829=CIRCLE ( 'NONE', #1788, 8.385254915620297567 ) ;
#7833=CARTESIAN_POINT ( 'NONE',  ( 9.723082553384461590, -72.03366436399431905, 2.708544018860256308 ) ) ;
#7837=AXIS2_PLACEMENT_3D ( 'NONE', #6122, #10394, #790 ) ;
#7838=CARTESIAN_POINT ( 'NONE',  ( 1.084353620409068652E-15, -38.76242177807012723, 6.844888786042043893E-17 ) ) ;
#7839=AXIS2_PLACEMENT_3D ( 'NONE', #11095, #10345, #12727 ) ;
#7840=CIRCLE ( 'NONE', #6957, 2.000000000000000000 ) ;
#7842=VERTEX_POINT ( 'NONE', #3849 ) ;
#7844=CARTESIAN_POINT ( 'NONE',  ( 15.29705854078138216, 76.22148119144830503, 30.59411708156277854 ) ) ;
#7846=CARTESIAN_POINT ( 'NONE',  ( -10.00000000000000711, 92.00000000000000000, -2.500000000000000000 ) ) ;
#7847=CARTESIAN_POINT ( 'NONE',  ( -2.008006351130390499, -80.00378950643924725, -9.910921267331605833 ) ) ;
#7848=VECTOR ( 'NONE', #7113, 1000.000000000000000 ) ;
#7849=ADVANCED_FACE ( 'NONE', ( #13640 ), #12416, .T. ) ;
#7853=CIRCLE ( 'NONE', #7188, 15.29705854078139105 ) ;
#7855=VERTEX_POINT ( 'NONE', #8339 ) ;
#7857=CARTESIAN_POINT ( 'NONE',  ( 8.804495088766337574, -73.18181818181338372, 4.925729831870250486 ) ) ;
#7859=CARTESIAN_POINT ( 'NONE',  ( 4.804172150869134406, 90.20479154739604155, 1.391179344134541473 ) ) ;
#7861=DIRECTION ( 'NONE',  ( 1.000000000000000000, 0.000000000000000000, 0.000000000000000000 ) ) ;
#7865=CARTESIAN_POINT ( 'NONE',  ( 4.547999443521274721, -70.00000000000000000, 2.077426547854386296 ) ) ;
#7867=CARTESIAN_POINT ( 'NONE',  ( 0.05313321603437554802, -142.5800865800495671, 3.258060136338194468 ) ) ;
#7868=DIRECTION ( 'NONE',  ( -0.000000000000000000, -0.000000000000000000, -1.000000000000000000 ) ) ;
#7870=DIRECTION ( 'NONE',  ( 2.797435172181480534E-17, -1.000000000000000000, 1.765856845898762164E-18 ) ) ;
#7872=EDGE_LOOP ( 'NONE', ( #2714, #5266, #2878, #3926 ) ) ;
#7873=EDGE_CURVE ( 'NONE', #11146, #11917, #10574, .T. ) ;
#7874=VERTEX_POINT ( 'NONE', #7145 ) ;
#7875=CARTESIAN_POINT ( 'NONE',  ( -8.385254915620295790, 90.00000000000000000, -1.589271161308885878E-16 ) ) ;
#7876=ORIENTED_EDGE ( 'NONE', *, *, #2597, .T. ) ;
#7883=DIRECTION ( 'NONE',  ( -0.9923485843107423543, -2.797833471351478217E-17, -0.1234677578012386562 ) ) ;
#7884=ORIENTED_EDGE ( 'NONE', *, *, #2697, .F. ) ;
#7885=DIRECTION ( 'NONE',  ( 1.000000000000000000, 0.000000000000000000, 0.000000000000000000 ) ) ;
#7886=DIRECTION ( 'NONE',  ( -2.797435172181481150E-17, 1.000000000000000000, -1.765856845898762549E-18 ) ) ;
#7887=CARTESIAN_POINT ( 'NONE',  ( 8.385254915620292238, 22.12961257269105531, 1.008767855514154504E-15 ) ) ;
#7888=B_SPLINE_CURVE_WITH_KNOTS ( 'NONE', 3,
 ( #7131, #11408, #4045, #4109 ),
 .UNSPECIFIED., .F., .F.,
 ( 4, 4 ),
 ( 0.000000000000000000, 1.000000000000000000 ),
 .UNSPECIFIED. ) ;
#7890=CARTESIAN_POINT ( 'NONE',  ( -8.385254915620295790, 69.25350232273815720, -1.222917711790730109E-16 ) ) ;
#7891=CARTESIAN_POINT ( 'NONE',  ( -2.595029975318955628, -79.59366873198513304, -9.795567015018859180 ) ) ;
#7892=CARTESIAN_POINT ( 'NONE',  ( 10.69381717166375267, 63.25855867215299355, 2.619229793989003951E-15 ) ) ;
#7896=EDGE_CURVE ( 'NONE', #12324, #4849, #11275, .T. ) ;
#7897=DIRECTION ( 'NONE',  ( -1.000000000000000000, 0.000000000000000000, 0.000000000000000000 ) ) ;
#7899=FACE_OUTER_BOUND ( 'NONE', #11970, .T. ) ;
#7904=SHAPE_DEFINITION_REPRESENTATION ( #8005, #1365 ) ;
#7905=ORIENTED_EDGE ( 'NONE', *, *, #8075, .T. ) ;
#7906=DIRECTION ( 'NONE',  ( -2.797435172181481150E-17, 1.000000000000000000, -1.765856845898762549E-18 ) ) ;
#7908=CARTESIAN_POINT ( 'NONE',  ( -15.29705854078138749, 38.52236939141059935, -6.802498971006334016E-17 ) ) ;
#7909=AXIS2_PLACEMENT_3D ( 'NONE', #2010, #11481, #12684 ) ;
#7910=CARTESIAN_POINT ( 'NONE',  ( -8.385254915620295790, 22.12961257269105531, 16.77050983124058448 ) ) ;
#7911=EDGE_CURVE ( 'NONE', #11359, #12557, #482, .T. ) ;
#7916=ORIENTED_EDGE ( 'NONE', *, *, #10213, .F. ) ;
#7919=CARTESIAN_POINT ( 'NONE',  ( 12.99553232110414669, -26.62435705548577047, 1.656305067313535556E-15 ) ) ;
#7921=ORIENTED_EDGE ( 'NONE', *, *, #707, .F. ) ;
#7923=CARTESIAN_POINT ( 'NONE',  ( -12.99553232110414491, -7.774801155466915858, -1.564035334333850472E-15 ) ) ;
#7927=CARTESIAN_POINT ( 'NONE',  ( 7.162946923110105502, -96.44493861733469942, 3.807625378222109003 ) ) ;
#7928=CARTESIAN_POINT ( 'NONE',  ( -8.385254915620288685, 15.32944684068712782, -16.77050983124058448 ) ) ;
#7932=ADVANCED_FACE ( 'NONE', ( #1885 ), #7105, .T. ) ;
#7934=EDGE_LOOP ( 'NONE', ( #4553, #6643, #10304, #336 ) ) ;
#7936=CARTESIAN_POINT ( 'NONE',  ( 9.940250983052006717, -69.87878787878412368, 1.425521750854503722 ) ) ;
#7938=CARTESIAN_POINT ( 'NONE',  ( 4.895853646792283520, 90.06529264441493865, 1.023585852534436347 ) ) ;
#7939=LINE ( 'NONE', #11090, #4001 ) ;
#7940=CARTESIAN_POINT ( 'NONE',  ( 15.29705854078139637, -18.02629830864593785, 1.919277763901059081E-15 ) ) ;
#7941=CARTESIAN_POINT ( 'NONE',  ( 0.3728392436379902586, -81.93939393934687132, -10.00978956350897064 ) ) ;
#7942=CARTESIAN_POINT ( 'NONE',  ( -8.385254915620297567, 78.67828027274755698, -1.389345798431728350E-16 ) ) ;
#7943=AXIS2_PLACEMENT_3D ( 'NONE', #5727, #7824, #2578 ) ;
#7945=CARTESIAN_POINT ( 'NONE',  ( -10.00000000000000711, 139.9999999999999716, -2.500000000000000000 ) ) ;
#7948=CIRCLE ( 'NONE', #8865, 8.385254915620294014 ) ;
#7949=ORIENTED_EDGE ( 'NONE', *, *, #9040, .F. ) ;
#7950=CARTESIAN_POINT ( 'NONE',  ( -4.340256562281096464, -97.38225965448614829, -6.691037544056555042 ) ) ;
#7951=CARTESIAN_POINT ( 'NONE',  ( -25.00000000000000355, 120.0000000000000284, 0.5000000000000000000 ) ) ;
#7955=DIRECTION ( 'NONE',  ( 1.000000000000000000, 0.000000000000000000, 0.000000000000000000 ) ) ;
#7957=CARTESIAN_POINT ( 'NONE',  ( 1.912509855227740641, -139.1821000271621926, 2.327450852377690005 ) ) ;
#7959=CARTESIAN_POINT ( 'NONE',  ( 4.471182088707192470, 90.98125128669738615, -2.240943909473569473 ) ) ;
#7963=DIRECTION ( 'NONE',  ( -1.000000000000000000, 0.000000000000000000, 0.000000000000000000 ) ) ;
#7965=DIRECTION ( 'NONE',  ( -2.797435172181481150E-17, 1.000000000000000000, -1.765856845898762549E-18 ) ) ;
#7967=CARTESIAN_POINT ( 'NONE',  ( -8.385254915620294014, 15.32944684068712782, 16.77050983124058092 ) ) ;
#7968=CIRCLE ( 'NONE', #9536, 5.000000000000000000 ) ;
#7969=VERTEX_POINT ( 'NONE', #5044 ) ;
#7970=CARTESIAN_POINT ( 'NONE',  ( 2.771542151761392070, 90.01585036846415733, 4.174539845741942479 ) ) ;
#7971=ORIENTED_EDGE ( 'NONE', *, *, #8397, .T. ) ;
#7973=CARTESIAN_POINT ( 'NONE',  ( 1.111721538977011203, -76.35064935050891677, 4.681383094373183340 ) ) ;
#7975=ORIENTED_EDGE ( 'NONE', *, *, #11073, .F. ) ;
#7979=ADVANCED_FACE ( 'NONE', ( #11826 ), #3274, .F. ) ;
#7981=CARTESIAN_POINT ( 'NONE',  ( 10.43546891138484511, -95.36363636363113017, 7.899666394170035133 ) ) ;
#7982=CARTESIAN_POINT ( 'NONE',  ( 12.99579180576516002, 7.534841976936129448, 25.99158361153033070 ) ) ;
#7985=CARTESIAN_POINT ( 'NONE',  ( -2.517691654963332357E-15, 90.00000000000000000, -1.589271161308885878E-16 ) ) ;
#7987=DIRECTION ( 'NONE',  ( -0.8000000000000008216, 0.5999999999999988676, 0.000000000000000000 ) ) ;
#7988=VERTEX_POINT ( 'NONE', #5373 ) ;
#7990=EDGE_CURVE ( 'NONE', #13685, #3535, #3826, .T. ) ;
#7991=ORIENTED_EDGE ( 'NONE', *, *, #8677, .F. ) ;
#7993=CARTESIAN_POINT ( 'NONE',  ( -8.385254915620297567, -34.41905512736551032, -1.990698649637279025E-15 ) ) ;
#7999=EDGE_CURVE ( 'NONE', #7762, #3806, #10759, .T. ) ;
#8001=CARTESIAN_POINT ( 'NONE',  ( 0.9785323935166234666, -82.17131360862762790, -9.727322450732026837 ) ) ;
#8002=CARTESIAN_POINT ( 'NONE',  ( 15.29705854078138216, 57.37192529142944863, 30.59411708156277854 ) ) ;
#8003=ORIENTED_EDGE ( 'NONE', *, *, #2420, .T. ) ;
#8004=ORIENTED_EDGE ( 'NONE', *, *, #1457, .T. ) ;
#8005=PRODUCT_DEFINITION_SHAPE ( 'NONE', 'NONE',  #2214 ) ;
#8006=EDGE_LOOP ( 'NONE', ( #1646, #11501, #8160, #2439 ) ) ;
#8008=LINE ( 'NONE', #11232, #106 ) ;
#8009=CARTESIAN_POINT ( 'NONE',  ( 2.142312913383998207, -80.12121212121218150, 9.955895698471858069 ) ) ;
#8010=( BOUNDED_SURFACE ( )  B_SPLINE_SURFACE ( 3, 3, ( 
 ( #4159, #6473, #5480, #9765 ),
 ( #10740, #11932, #6543, #2323 ),
 ( #10869, #4566, #11798, #9832 ),
 ( #311, #5696, #1417, #9980 ) ),
 .UNSPECIFIED., .F., .F., .T. ) 
 B_SPLINE_SURFACE_WITH_KNOTS ( ( 4, 4 ),
 ( 4, 4 ),
 ( 0.000000000000000000, 1.000000000000000000 ),
 ( 0.000000000000000000, 1.000000000000000000 ),
 .UNSPECIFIED. ) 
 GEOMETRIC_REPRESENTATION_ITEM ( )  RATIONAL_B_SPLINE_SURFACE ( (
 ( 1.000000000000000000, 0.3333333333333334259, 0.3333333333333334259, 1.000000000000000000),
 ( 1.000000000000000000, 0.3333333333333334259, 0.3333333333333334259, 1.000000000000000000),
 ( 1.000000000000000000, 0.3333333333333334259, 0.3333333333333334259, 1.000000000000000000),
 ( 1.000000000000000000, 0.3333333333333334259, 0.3333333333333334259, 1.000000000000000000) ) ) 
 REPRESENTATION_ITEM ( '' )  SURFACE ( )  );
#8011=ORIENTED_EDGE ( 'NONE', *, *, #9381, .T. ) ;
#8012=CARTESIAN_POINT ( 'NONE',  ( 1.964926810246274247, -77.94210575524361673, 9.914063055205920350 ) ) ;
#8014=CARTESIAN_POINT ( 'NONE',  ( 5.925229457222553897, -117.0909090909068482, 2.047657493157430952 ) ) ;
#8016=CARTESIAN_POINT ( 'NONE',  ( -6.764234067550082941, -111.2727272727269821, 0.6609924544552703285 ) ) ;
#8017=EDGE_CURVE ( 'NONE', #3902, #4278, #4477, .T. ) ;
#8018=FACE_OUTER_BOUND ( 'NONE', #9596, .T. ) ;
#8020=DIRECTION ( 'NONE',  ( -1.000000000000000000, 0.000000000000000000, 0.000000000000000000 ) ) ;
#8022=VERTEX_POINT ( 'NONE', #13408 ) ;
#8023=ORIENTED_EDGE ( 'NONE', *, *, #8185, .F. ) ;
#8024=CARTESIAN_POINT ( 'NONE',  ( -3.661863250968810046, -131.0369695719847982, 1.478767330369552768 ) ) ;
#8025=DIRECTION ( 'NONE',  ( -5.551115123125776539E-17, 1.000000000000000000, 3.944304526105059027E-31 ) ) ;
#8028=DIRECTION ( 'NONE',  ( -0.000000000000000000, -0.000000000000000000, -1.000000000000000000 ) ) ;
#8029=ORIENTED_EDGE ( 'NONE', *, *, #13514, .F. ) ;
#8033=CARTESIAN_POINT ( 'NONE',  ( -31.81818181818181657, 133.3608531424536920, 2.500000000000000000 ) ) ;
#8036=CARTESIAN_POINT ( 'NONE',  ( 1.947606478028208261E-13, -70.00000000000000000, 2.411204079342396664E-14 ) ) ;
#8037=LINE ( 'NONE', #2709, #10323 ) ;
#8039=AXIS2_PLACEMENT_3D ( 'NONE', #1967, #3148, #10652 ) ;
#8041=CARTESIAN_POINT ( 'NONE',  ( 3.523137085080620956, 90.23509738553477177, 3.551515709300293366 ) ) ;
#8042=CARTESIAN_POINT ( 'NONE',  ( 18.84535726572642034, -167.3636363553120532, 7.741214183180429309 ) ) ;
#8047=CARTESIAN_POINT ( 'NONE',  ( -3.784192700541033183, -169.0000000000003126, -1.982393907671172961 ) ) ;
#8051=CARTESIAN_POINT ( 'NONE',  ( 6.266477192377021943, -76.69310173738496417, 7.966230643697302938 ) ) ;
#8052=ORIENTED_EDGE ( 'NONE', *, *, #7896, .F. ) ;
#8053=ORIENTED_EDGE ( 'NONE', *, *, #4702, .F. ) ;
#8058=CARTESIAN_POINT ( 'NONE',  ( -10.69346802281034670, -25.79937747632526879, -1.218456123918935934E-15 ) ) ;
#8060=CARTESIAN_POINT ( 'NONE',  ( -8.385254915620301119, 78.67828027274755698, 16.77050983124059158 ) ) ;
#8061=DIRECTION ( 'NONE',  ( -0.000000000000000000, -0.000000000000000000, -1.000000000000000000 ) ) ;
#8062=( BOUNDED_SURFACE ( )  B_SPLINE_SURFACE ( 3, 3, ( 
 ( #4320, #474, #8599, #13251 ),
 ( #1358, #12903, #2407, #5638 ),
 ( #3457, #3523, #12168, #6689 ),
 ( #12753, #11690, #7736, #2084 ) ),
 .UNSPECIFIED., .F., .F., .T. ) 
 B_SPLINE_SURFACE_WITH_KNOTS ( ( 4, 4 ),
 ( 4, 4 ),
 ( 0.000000000000000000, 1.000000000000000000 ),
 ( 0.000000000000000000, 1.000000000000000000 ),
 .UNSPECIFIED. ) 
 GEOMETRIC_REPRESENTATION_ITEM ( )  RATIONAL_B_SPLINE_SURFACE ( (
 ( 1.000000000000000000, 0.3333333333333334259, 0.3333333333333334259, 1.000000000000000000),
 ( 1.000000000000000000, 0.3333333333333334259, 0.3333333333333334259, 1.000000000000000000),
 ( 1.000000000000000000, 0.3333333333333334259, 0.3333333333333334259, 1.000000000000000000),
 ( 1.000000000000000000, 0.3333333333333334259, 0.3333333333333334259, 1.000000000000000000) ) ) 
 REPRESENTATION_ITEM ( '' )  SURFACE ( )  );
#8064=CARTESIAN_POINT ( 'NONE',  ( -1.147385087825261607, -80.61700017096171678, -9.985132701286346446 ) ) ;
#8065=CARTESIAN_POINT ( 'NONE',  ( -15.29705854078138394, 17.78624592198638155, -30.59411708156277854 ) ) ;
#8069=EDGE_LOOP ( 'NONE', ( #4166, #9876, #9421, #12139 ) ) ;
#8071=EDGE_CURVE ( 'NONE', #1714, #11917, #5789, .T. ) ;
#8072=CARTESIAN_POINT ( 'NONE',  ( -8.256647985966802494, -92.46527916421074167, -2.505673630511644934 ) ) ;
#8074=CARTESIAN_POINT ( 'NONE',  ( -10.69346802281035025, -6.949821576306441706, 21.38693604562069339 ) ) ;
#8075=EDGE_CURVE ( 'NONE', #6545, #7000, #616, .T. ) ;
#8077=ORIENTED_EDGE ( 'NONE', *, *, #5940, .T. ) ;
#8079=CARTESIAN_POINT ( 'NONE',  ( 4.858750903448073366, -78.09090909090949140, 8.996753037508748108 ) ) ;
#8080=ORIENTED_EDGE ( 'NONE', *, *, #9857, .F. ) ;
#8081=CARTESIAN_POINT ( 'NONE',  ( 4.471144793536856454, 90.98178511618806397, 2.240986362385854580 ) ) ;
#8083=VECTOR ( 'NONE', #2779, 1000.000000000000000 ) ;
#8085=CARTESIAN_POINT ( 'NONE',  ( -15.29705854078138749, 10.24803554138234496, -1.809656371776380929E-17 ) ) ;
#8086=CARTESIAN_POINT ( 'NONE',  ( -5.494716852924834249, -106.9090909090907502, 4.862358660864143367 ) ) ;
#8089=AXIS2_PLACEMENT_3D ( 'NONE', #7286, #9190, #9333 ) ;
#8090=FACE_OUTER_BOUND ( 'NONE', #8006, .T. ) ;
#8092=EDGE_LOOP ( 'NONE', ( #7501, #9555, #2472, #11945 ) ) ;
#8095=CARTESIAN_POINT ( 'NONE',  ( 6.191228697746712584, -110.8526145195744306, -1.341853914380320978 ) ) ;
#8097=ADVANCED_FACE ( 'NONE', ( #6071 ), #12525, .T. ) ;
#8100=CARTESIAN_POINT ( 'NONE',  ( 0.000000000000000000, 71.01020514433645303, 0.5000000000000000000 ) ) ;
#8101=CARTESIAN_POINT ( 'NONE',  ( -4.975586992323414874E-16, 17.78624592198638155, -3.140796412417860432E-17 ) ) ;
#8102=ORIENTED_EDGE ( 'NONE', *, *, #11827, .F. ) ;
#8103=CARTESIAN_POINT ( 'NONE',  ( -49.99999999999999289, 120.0000000000000284, 0.5000000000000000000 ) ) ;
#8104=CARTESIAN_POINT ( 'NONE',  ( 2.989041064089018374, -128.2926750340500917, -3.053002924880402702 ) ) ;
#8105=CARTESIAN_POINT ( 'NONE',  ( -36.36363636363635976, 142.2680885707561629, 0.5000000000000000000 ) ) ;
#8108=CARTESIAN_POINT ( 'NONE',  ( -10.00000000000000000, 99.99999999999994316, 2.500000000000000000 ) ) ;
#8109=CARTESIAN_POINT ( 'NONE',  ( -15.29705854078139105, 47.94714734142005597, -8.466779837416320124E-17 ) ) ;
#8110=AXIS2_PLACEMENT_3D ( 'NONE', #307, #9827, #5619 ) ;
#8111=ORIENTED_EDGE ( 'NONE', *, *, #2997, .F. ) ;
#8112=DIRECTION ( 'NONE',  ( -1.000000000000000000, 0.000000000000000000, 0.000000000000000000 ) ) ;
#8114=CARTESIAN_POINT ( 'NONE',  ( 11.95302590260997455, -161.0909090909845816, 5.173310689862941736 ) ) ;
#8116=ORIENTED_EDGE ( 'NONE', *, *, #6269, .F. ) ;
#8117=EDGE_LOOP ( 'NONE', ( #3377, #854, #6637, #8111 ) ) ;
#8120=VECTOR ( 'NONE', #951, 1000.000000000000000 ) ;
#8121=CARTESIAN_POINT ( 'NONE',  ( -6.139211203638544667, -76.35064935069904379, -12.15884065890355181 ) ) ;
#8122=DIRECTION ( 'NONE',  ( 0.000000000000000000, 0.000000000000000000, 1.000000000000000000 ) ) ;
#8126=DIRECTION ( 'NONE',  ( 1.000000000000000000, 0.000000000000000000, 0.000000000000000000 ) ) ;
#8128=ORIENTED_EDGE ( 'NONE', *, *, #12391, .T. ) ;
#8131=CARTESIAN_POINT ( 'NONE',  ( 8.385254915620288685, 78.67828027274755698, 16.77050983124059158 ) ) ;
#8132=CARTESIAN_POINT ( 'NONE',  ( -12.99579180576516713, -1.889935973073298525, -3.189601575276258806E-15 ) ) ;
#8134=CARTESIAN_POINT ( 'NONE',  ( -5.810149393362634918, -114.7767544601693430, 0.9592521923076761103 ) ) ;
#8135=CARTESIAN_POINT ( 'NONE',  ( -8.385254915620290461, -31.79444290936001494, -16.77050983124059158 ) ) ;
#8136=ORIENTED_EDGE ( 'NONE', *, *, #2761, .T. ) ;
#8137=AXIS2_PLACEMENT_3D ( 'NONE', #5329, #8552, #13543 ) ;
#8138=ORIENTED_EDGE ( 'NONE', *, *, #6870, .F. ) ;
#8139=ORIENTED_EDGE ( 'NONE', *, *, #12822, .F. ) ;
#8140=DIRECTION ( 'NONE',  ( -1.000000000000000000, 0.000000000000000000, 0.000000000000000000 ) ) ;
#8141=CARTESIAN_POINT ( 'NONE',  ( -12.99553232110414847, -26.62435705548576692, 25.99106464220827917 ) ) ;
#8142=VECTOR ( 'NONE', #3649, 1000.000000000000000 ) ;
#8143=DIRECTION ( 'NONE',  ( -2.797435172181481150E-17, 1.000000000000000000, -1.765856845898762549E-18 ) ) ;
#8146=( BOUNDED_SURFACE ( )  B_SPLINE_SURFACE ( 3, 3, ( 
 ( #356, #3774, #4614, #7757 ),
 ( #10018, #5892, #13428, #12343 ),
 ( #7919, #12199, #13119, #2517 ),
 ( #2733, #2588, #6866, #13203 ) ),
 .UNSPECIFIED., .F., .F., .T. ) 
 B_SPLINE_SURFACE_WITH_KNOTS ( ( 4, 4 ),
 ( 4, 4 ),
 ( 0.000000000000000000, 1.000000000000000000 ),
 ( 0.000000000000000000, 1.000000000000000000 ),
 .UNSPECIFIED. ) 
 GEOMETRIC_REPRESENTATION_ITEM ( )  RATIONAL_B_SPLINE_SURFACE ( (
 ( 1.000000000000000000, 0.3333333333333334259, 0.3333333333333334259, 1.000000000000000000),
 ( 1.000000000000000000, 0.3333333333333334259, 0.3333333333333334259, 1.000000000000000000),
 ( 1.000000000000000000, 0.3333333333333334259, 0.3333333333333334259, 1.000000000000000000),
 ( 1.000000000000000000, 0.3333333333333334259, 0.3333333333333334259, 1.000000000000000000) ) ) 
 REPRESENTATION_ITEM ( '' )  SURFACE ( )  );
#8148=FACE_OUTER_BOUND ( 'NONE', #4956, .T. ) ;
#8150=CARTESIAN_POINT ( 'NONE',  ( -5.925229457222161322, -117.0909090909115235, -2.047657493157731157 ) ) ;
#8152=DIRECTION ( 'NONE',  ( -1.000000000000000000, 0.000000000000000000, 0.000000000000000000 ) ) ;
#8155=EDGE_CURVE ( 'NONE', #357, #3902, #8037, .T. ) ;
#8158=ORIENTED_EDGE ( 'NONE', *, *, #7990, .T. ) ;
#8160=ORIENTED_EDGE ( 'NONE', *, *, #984, .F. ) ;
#8161=AXIS2_PLACEMENT_3D ( 'NONE', #3079, #5251, #9539 ) ;
#8162=CARTESIAN_POINT ( 'NONE',  ( -2.946076804534930815, -128.2487050844958674, 3.060050242327970071 ) ) ;
#8165=EDGE_LOOP ( 'NONE', ( #246, #10164, #10123, #13861 ) ) ;
#8167=CARTESIAN_POINT ( 'NONE',  ( -0.4690429436946310093, -122.4721769046603868, -4.906597864725500635 ) ) ;
#8169=CARTESIAN_POINT ( 'NONE',  ( 15.29705854078138927, 90.00000000000000000, 1.714422261702872766E-15 ) ) ;
#8170=CARTESIAN_POINT ( 'NONE',  ( 4.355466475183198247E-16, -15.56949922734665570, 2.749350679782564022E-17 ) ) ;
#8171=FACE_OUTER_BOUND ( 'NONE', #1459, .T. ) ;
#8173=CYLINDRICAL_SURFACE ( 'NONE', #911, 2.000000000000000000 ) ;
#8174=ADVANCED_FACE ( 'NONE', ( #2842 ), #8173, .T. ) ;
#8175=CARTESIAN_POINT ( 'NONE',  ( 15.29705854078138749, 64.91013567203349055, 30.59411708156278564 ) ) ;
#8178=CARTESIAN_POINT ( 'NONE',  ( -10.91573825925852859, -140.5584415584503404, -8.453432789889644638 ) ) ;
#8179=AXIS2_PLACEMENT_3D ( 'NONE', #180, #5703, #3381 ) ;
#8182=VERTEX_POINT ( 'NONE', #3894 ) ;
#8183=CARTESIAN_POINT ( 'NONE',  ( -4.471144793536862672, 90.98178511618806397, -2.240986362385854580 ) ) ;
#8184=FACE_OUTER_BOUND ( 'NONE', #4450, .T. ) ;
#8185=EDGE_CURVE ( 'NONE', #11917, #10214, #11442, .T. ) ;
#8186=CARTESIAN_POINT ( 'NONE',  ( -11.72298137502704840, -61.00000000000002842, -2.970135970080977739 ) ) ;
#8187=CARTESIAN_POINT ( 'NONE',  ( 8.385254915620292238, 5.904668890677672088, 2.053795118489800004E-15 ) ) ;
#8188=LINE ( 'NONE', #11342, #11785 ) ;
#8189=CIRCLE ( 'NONE', #2126, 8.385254915620294014 ) ;
#8191=FACE_OUTER_BOUND ( 'NONE', #7585, .T. ) ;
#8192=DIRECTION ( 'NONE',  ( -2.797435172181481150E-17, 1.000000000000000000, -1.765856845898762549E-18 ) ) ;
#8193=AXIS2_PLACEMENT_3D ( 'NONE', #1409, #10931, #382 ) ;
#8194=TOROIDAL_SURFACE ( 'NONE', #13609, 16.99999999999998934, 2.000000000000000000 ) ;
#8196=ORIENTED_EDGE ( 'NONE', *, *, #3710, .F. ) ;
#8201=CARTESIAN_POINT ( 'NONE',  ( -10.00000000000000711, 99.99999999999994316, 2.500000000000000000 ) ) ;
#8203=CARTESIAN_POINT ( 'NONE',  ( -12.99553232110414314, 29.92431064457076673, -3.246435148940206039E-15 ) ) ;
#8205=DIRECTION ( 'NONE',  ( -0.4545454545454531425, 0.8907235428302472391, 0.000000000000000000 ) ) ;
#8206=CARTESIAN_POINT ( 'NONE',  ( 2.607178694270818831, -83.43640819696341282, -9.281062047519146319 ) ) ;
#8207=CARTESIAN_POINT ( 'NONE',  ( 1.958204620527036102E-15, -69.99999999999998579, 1.236099792129133461E-16 ) ) ;
#8209=EDGE_LOOP ( 'NONE', ( #9819, #933, #3644, #7089 ) ) ;
#8216=CARTESIAN_POINT ( 'NONE',  ( -1.026257020618903670, -73.45454545136195179, -21.46608457335733178 ) ) ;
#8218=CARTESIAN_POINT ( 'NONE',  ( -0.03701750592458041833, -157.3626971396553529, -1.516132001818238706 ) ) ;
#8219=CARTESIAN_POINT ( 'NONE',  ( 10.00000000000000000, 90.00000000000000000, 2.500000000000000000 ) ) ;
#8222=ORIENTED_EDGE ( 'NONE', *, *, #2516, .F. ) ;
#8224=CARTESIAN_POINT ( 'NONE',  ( 3.364289002660265204, -118.5204725339004597, 4.219879093570879647 ) ) ;
#8226=CYLINDRICAL_SURFACE ( 'NONE', #263, 15.29705854078139105 ) ;
#8228=CARTESIAN_POINT ( 'NONE',  ( -8.385254915620292238, 22.12961257269105531, -3.907772785857374249E-17 ) ) ;
#8230=DIRECTION ( 'NONE',  ( -1.000000000000000000, 0.000000000000000000, 0.000000000000000000 ) ) ;
#8232=CARTESIAN_POINT ( 'NONE',  ( -1.066429238991507766, -167.9999999999998863, 0.4719413927851786594 ) ) ;
#8233=CARTESIAN_POINT ( 'NONE',  ( -8.385254915620292238, -22.36966495935058319, 3.950162600893091522E-17 ) ) ;
#8234=CARTESIAN_POINT ( 'NONE',  ( -12.99553232110413425, 20.49953269456136695, -25.99106464220827917 ) ) ;
#8236=CARTESIAN_POINT ( 'NONE',  ( 15.29705854078139282, 90.00000000000000000, 1.714422261702873160E-15 ) ) ;
#8237=CARTESIAN_POINT ( 'NONE',  ( -12.99553232110414314, 29.92431064457076673, -1.697177803646649065E-15 ) ) ;
#8238=EDGE_CURVE ( 'NONE', #2048, #1705, #13501, .T. ) ;
#8240=DIRECTION ( 'NONE',  ( 0.000000000000000000, 0.000000000000000000, 1.000000000000000000 ) ) ;
#8242=CARTESIAN_POINT ( 'NONE',  ( 12.05308885558885024, -134.6363636363533942, -5.101645771607613788 ) ) ;
#8244=ORIENTED_EDGE ( 'NONE', *, *, #950, .T. ) ;
#8247=CARTESIAN_POINT ( 'NONE',  ( -8.385254915620294014, 90.00000000000000000, -1.589271161308885878E-16 ) ) ;
#8249=CARTESIAN_POINT ( 'NONE',  ( 8.385254915620292238, 59.82872437272870769, 9.189312520034297072E-16 ) ) ;
#8251=CARTESIAN_POINT ( 'NONE',  ( -8.385254915620292238, 34.17900274070598243, -2.138129980707100895E-15 ) ) ;
#8252=AXIS2_PLACEMENT_3D ( 'NONE', #4621, #5456, #8902 ) ;
#8254=CARTESIAN_POINT ( 'NONE',  ( -12.99553232110414314, 48.77386654458962312, -1.763749038303048460E-15 ) ) ;
#8255=CARTESIAN_POINT ( 'NONE',  ( 15.29705854078138927, 90.00000000000000000, 1.714422261702872766E-15 ) ) ;
#8256=DIRECTION ( 'NONE',  ( -2.797435172181481150E-17, 1.000000000000000000, -1.765856845898762549E-18 ) ) ;
#8259=EDGE_CURVE ( 'NONE', #11738, #13355, #5378, .T. ) ;
#8260=AXIS2_PLACEMENT_3D ( 'NONE', #9132, #654, #12428 ) ;
#8264=ORIENTED_EDGE ( 'NONE', *, *, #5886, .F. ) ;
#8265=CARTESIAN_POINT ( 'NONE',  ( 8.385254915620292238, -22.36966495935058319, 1.068716529980328543E-15 ) ) ;
#8267=VECTOR ( 'NONE', #8595, 1000.000000000000000 ) ;
#8268=CARTESIAN_POINT ( 'NONE',  ( -10.69346802281034314, 30.74929022373127196, -21.38693604562069694 ) ) ;
#8269=CARTESIAN_POINT ( 'NONE',  ( 8.385254915620294014, -3.520109059331755219, -16.77050983124058092 ) ) ;
#8270=CARTESIAN_POINT ( 'NONE',  ( -0.005328072727578240381, -157.8884954289838447, 1.500081365927933508 ) ) ;
#8271=CLOSED_SHELL ( 'NONE', ( #5778, #12085, #9872, #4872, #8332, #10856, #1725, #6176, #193, #2387, #8851, #9336, #5754, #192, #12236, #10790, #9598, #4120, #4978, #4630, #8642, #12103, #6681, #3125, #4531, #9028, #3170, #3410, #8573, #13846, #10440, #1379, #5415, #3595, #1210, #1312, #12311, #10706, #10900, #9026, #7437, #11050, #3530, #11687, #12379, #1394, #12569, #11347, #5500, #176, #12060, #2758, #3697, #7629, #12880, #4626, #7703, #4481, #631, #5835, #503, #1048, #5849, #11656, #12686, #4286, #7046, #11428, #5304, #2068, #6444, #1360, #7849, #5874, #3332, #2007, #4396, #10384, #12633, #12806, #13607, #11157, #4735, #1838, #3600, #3395, #9030, #6872, #21, #13340, #1303, #5020, #955, #10157, #8560, #10307, #5487, #4008, #10782, #2426, #13680, #8174, #7354, #12206, #4967, #10029, #7979, #935, #9393, #949, #10032, #500, #6111, #5324, #10877, #3778, #11486, #10724, #8097, #198, #10152, #8665, #10326, #3448, #8920, #13850, #8814, #7016, #8869, #4541, #6024, #5041, #10403, #7306, #10033, #8661, #11654, #4982, #7230, #9458, #13054, #13037, #2503, #7932, #2302, #9443, #5921, #3339, #3427, #2826, #9768, #3353, #2667, #1796, #6288, #8601, #5960, #3268, #1648, #7539, #112, #850, #13133, #1523, #7037, #9180, #5156, #12651, #1136, #8812, #13156 ) ) ;
#8274=ORIENTED_EDGE ( 'NONE', *, *, #5316, .T. ) ;
#8276=CIRCLE ( 'NONE', #4018, 2.000000000000000000 ) ;
#8277=ORIENTED_EDGE ( 'NONE', *, *, #7116, .T. ) ;
#8280=ORIENTED_EDGE ( 'NONE', *, *, #776, .T. ) ;
#8281=CARTESIAN_POINT ( 'NONE',  ( 6.150798755069183166, -74.45454545454636275, 8.129532795066678474 ) ) ;
#8282=VERTEX_POINT ( 'NONE', #12874 ) ;
#8284=DIRECTION ( 'NONE',  ( 0.000000000000000000, 0.000000000000000000, 1.000000000000000000 ) ) ;
#8288=CARTESIAN_POINT ( 'NONE',  ( 4.126438786023406635, -120.8149455287847758, 3.030370511718414317 ) ) ;
#8289=CARTESIAN_POINT ( 'NONE',  ( 38.79999999999999716, 101.5999999999999943, 0.5000000000000000000 ) ) ;
#8290=ORIENTED_EDGE ( 'NONE', *, *, #12107, .F. ) ;
#8292=B_SPLINE_CURVE_WITH_KNOTS ( 'NONE', 3,
 ( #6947, #1759, #10181, #7938, #10321, #7859, #4785, #9062, #2534, #5760, #8081, #10038, #12145, #4705 ),
 .UNSPECIFIED., .F., .F.,
 ( 4, 2, 2, 2, 2, 2, 4 ),
 ( 0.000000000000000000, 0.0003997920717328745199, 0.0007995841434657493651, 0.001199376215198624156, 0.001599168286931499164, 0.002398752430397248312, 0.003198336573862998328 ),
 .UNSPECIFIED. ) ;
#8293=VECTOR ( 'NONE', #3492, 1000.000000000000000 ) ;
#8294=EDGE_LOOP ( 'NONE', ( #431, #6025, #13849, #1199 ) ) ;
#8298=CIRCLE ( 'NONE', #2239, 2.000000000000000000 ) ;
#8299=DIRECTION ( 'NONE',  ( 1.000000000000000000, 0.000000000000000000, 0.000000000000000000 ) ) ;
#8300=CARTESIAN_POINT ( 'NONE',  ( 6.383362303552328143, -84.46817857652109751, -7.102163859751367880 ) ) ;
#8303=VECTOR ( 'NONE', #5182, 1000.000000000000000 ) ;
#8307=DIRECTION ( 'NONE',  ( -2.797435172181481150E-17, 1.000000000000000000, -1.765856845898762549E-18 ) ) ;
#8308=EDGE_CURVE ( 'NONE', #5091, #4998, #3139, .T. ) ;
#8310=CARTESIAN_POINT ( 'NONE',  ( 8.385254915620292238, -3.520109059331727241, 1.035430912652128846E-15 ) ) ;
#8312=DIRECTION ( 'NONE',  ( -1.000000000000000000, 0.000000000000000000, 0.000000000000000000 ) ) ;
#8313=AXIS2_PLACEMENT_3D ( 'NONE', #4180, #770, #4971 ) ;
#8315=CIRCLE ( 'NONE', #5618, 8.385254915620292238 ) ;
#8317=VERTEX_POINT ( 'NONE', #11463 ) ;
#8322=CARTESIAN_POINT ( 'NONE',  ( 3.628753873946515718, -79.03030303033179393, 9.983370075670988442 ) ) ;
#8323=CARTESIAN_POINT ( 'NONE',  ( 20.16774360776483732, -62.63636365604191525, -2.887214122427654406 ) ) ;
#8324=CIRCLE ( 'NONE', #726, 8.385254915620294014 ) ;
#8327=EDGE_CURVE ( 'NONE', #2969, #11439, #10754, .T. ) ;
#8331=EDGE_CURVE ( 'NONE', #8182, #30, #6970, .T. ) ;
#8332=ADVANCED_FACE ( 'NONE', ( #9498 ), #8010, .T. ) ;
#8335=ORIENTED_EDGE ( 'NONE', *, *, #4187, .F. ) ;
#8336=DIRECTION ( 'NONE',  ( 0.000000000000000000, 0.000000000000000000, 1.000000000000000000 ) ) ;
#8337=CARTESIAN_POINT ( 'NONE',  ( -15.29705854078138927, 66.79670324143890525, -2.109256209238486313E-15 ) ) ;
#8338=CARTESIAN_POINT ( 'NONE',  ( 25.00000000000000355, 120.0000000000000284, -0.5000000000000000000 ) ) ;
#8339=CARTESIAN_POINT ( 'NONE',  ( 8.385254915620292238, 69.25350232273815720, 9.022884433393300556E-16 ) ) ;
#8340=CARTESIAN_POINT ( 'NONE',  ( -1.620286128678860127, -125.1459947693864194, -4.334625215706721768 ) ) ;
#8341=CARTESIAN_POINT ( 'NONE',  ( -12.99553232110413425, 48.77386654458962312, -25.99106464220827917 ) ) ;
#8342=ORIENTED_EDGE ( 'NONE', *, *, #10547, .T. ) ;
#8344=VERTEX_POINT ( 'NONE', #6748 ) ;
#8348=DIRECTION ( 'NONE',  ( 1.000000000000000000, 0.000000000000000000, 0.000000000000000000 ) ) ;
#8350=CARTESIAN_POINT ( 'NONE',  ( -12.97449437267216865, -39.59556244224027211, -25.94898874534435151 ) ) ;
#8351=ORIENTED_EDGE ( 'NONE', *, *, #6708, .F. ) ;
#8352=CARTESIAN_POINT ( 'NONE',  ( 10.69346802281034492, 11.89973432371241380, 0.000000000000000000 ) ) ;
#8356=AXIS2_PLACEMENT_3D ( 'NONE', #12759, #3073, #2022 ) ;
#8357=CARTESIAN_POINT ( 'NONE',  ( -2.861434295120944160, -135.9613303536295348, 1.766772280313772203 ) ) ;
#8358=LINE ( 'NONE', #4076, #3253 ) ;
#8362=EDGE_LOOP ( 'NONE', ( #4807, #3855, #622, #679 ) ) ;
#8363=VECTOR ( 'NONE', #7226, 1000.000000000000000 ) ;
#8364=CARTESIAN_POINT ( 'NONE',  ( 15.29705854078138572, 38.52236939141059935, 3.746698755667520834E-15 ) ) ;
#8367=CARTESIAN_POINT ( 'NONE',  ( 8.845718597664788518, -89.07293163041987327, -1.670562313001050292 ) ) ;
#8368=CARTESIAN_POINT ( 'NONE',  ( 12.97449437267217753, -39.59556244224027211, 0.000000000000000000 ) ) ;
#8369=CARTESIAN_POINT ( 'NONE',  ( -2.517691654963332357E-15, 90.00000000000000000, -1.589271161308885878E-16 ) ) ;
#8373=FACE_OUTER_BOUND ( 'NONE', #7439, .T. ) ;
#8374=VECTOR ( 'NONE', #312, 1000.000000000000000 ) ;
#8378=CARTESIAN_POINT ( 'NONE',  ( 0.1916457366472302803, -105.1818181818151317, 4.609965990740150232 ) ) ;
#8384=LINE ( 'NONE', #118, #5043 ) ;
#8388=CARTESIAN_POINT ( 'NONE',  ( 25.00000000000000355, 120.0000000000000284, 2.500000000000000000 ) ) ;
#8390=CYLINDRICAL_SURFACE ( 'NONE', #7909, 15.29705854078139460 ) ;
#8392=CARTESIAN_POINT ( 'NONE',  ( 11.81226048336477064, -40.00941361824966691, 2.893169398329486201E-15 ) ) ;
#8394=ORIENTED_EDGE ( 'NONE', *, *, #4368, .F. ) ;
#8397=EDGE_CURVE ( 'NONE', #9893, #6779, #6295, .T. ) ;
#8398=VERTEX_POINT ( 'NONE', #13231 ) ;
#8402=CARTESIAN_POINT ( 'NONE',  ( -15.29705854078139282, 66.79670324143890525, 30.59411708156276788 ) ) ;
#8403=AXIS2_PLACEMENT_3D ( 'NONE', #31, #7370, #7241 ) ;
#8404=DIRECTION ( 'NONE',  ( -1.000000000000000000, 0.000000000000000000, 0.000000000000000000 ) ) ;
#8405=CARTESIAN_POINT ( 'NONE',  ( 2.615685906363557134, -134.4805512794541187, -2.371495061727838305 ) ) ;
#8407=VERTEX_POINT ( 'NONE', #9695 ) ;
#8408=ORIENTED_EDGE ( 'NONE', *, *, #13664, .T. ) ;
#8409=CIRCLE ( 'NONE', #2819, 8.385254915620292238 ) ;
#8414=AXIS2_PLACEMENT_3D ( 'NONE', #1703, #7870, #4793 ) ;
#8419=EDGE_CURVE ( 'NONE', #13516, #283, #10984, .T. ) ;
#8420=CARTESIAN_POINT ( 'NONE',  ( 8.385254915620292238, 5.904668890677672088, 1.018788103988028800E-15 ) ) ;
#8426=CARTESIAN_POINT ( 'NONE',  ( -12.99553232110414491, -17.19957910547634228, -1.530749717005650972E-15 ) ) ;
#8427=CARTESIAN_POINT ( 'NONE',  ( 4.459053427763567612, -109.9755374418222829, -4.679063774435563872 ) ) ;
#8430=ORIENTED_EDGE ( 'NONE', *, *, #4296, .F. ) ;
#8432=B_SPLINE_CURVE_WITH_KNOTS ( 'NONE', 3,
 ( #238, #11931, #6667, #7654 ),
 .UNSPECIFIED., .F., .F.,
 ( 4, 4 ),
 ( 0.000000000000000000, 1.000000000000000000 ),
 .UNSPECIFIED. ) ;
#8433=CARTESIAN_POINT ( 'NONE',  ( -8.385254915620297567, 40.97916847270985841, 16.77050983124058448 ) ) ;
#8434=CARTESIAN_POINT ( 'NONE',  ( 1.493586498966360088, -80.00119264582536971, 9.937293197986129201 ) ) ;
#8435=CARTESIAN_POINT ( 'NONE',  ( 10.69346802281034847, 40.17406817374067174, -21.38693604562068984 ) ) ;
#8436=CARTESIAN_POINT ( 'NONE',  ( 8.747338040274810211, -91.10717937812032119, 0.8989578942604090628 ) ) ;
#8438=CARTESIAN_POINT ( 'NONE',  ( -8.385254915620292238, 62.45333659073423860, -2.210618003686766271E-15 ) ) ;
#8439=CARTESIAN_POINT ( 'NONE',  ( 12.99553232110414136, 20.49953269456136695, 1.563396152262992288E-15 ) ) ;
#8440=CARTESIAN_POINT ( 'NONE',  ( 15.29705854078139815, 0.8232575913729167638, -30.59411708156277854 ) ) ;
#8442=DIRECTION ( 'NONE',  ( -0.000000000000000000, -0.000000000000000000, -1.000000000000000000 ) ) ;
#8446=DIRECTION ( 'NONE',  ( 0.000000000000000000, 0.000000000000000000, 1.000000000000000000 ) ) ;
#8447=CARTESIAN_POINT ( 'NONE',  ( -8.943257790340283009, -76.35064935061960512, -10.27353203466038423 ) ) ;
#8448=ORIENTED_EDGE ( 'NONE', *, *, #2410, .F. ) ;
#8449=DIRECTION ( 'NONE',  ( -2.797435172181481150E-17, 1.000000000000000000, -1.765856845898762549E-18 ) ) ;
#8454=CARTESIAN_POINT ( 'NONE',  ( 2.937342332081942953, -95.36363636365133800, 3.570487953802512049 ) ) ;
#8455=LINE ( 'NONE', #11681, #2243 ) ;
#8458=CARTESIAN_POINT ( 'NONE',  ( -1.219787497442949287E-15, 43.60378069071538221, -7.699803463976802609E-17 ) ) ;
#8459=DIRECTION ( 'NONE',  ( -0.1234677578012386562, -1.701584941912606716E-18, 0.9923485843107423543 ) ) ;
#8461=CIRCLE ( 'NONE', #1302, 15.29705854078139993 ) ;
#8462=VERTEX_POINT ( 'NONE', #5989 ) ;
#8463=FACE_OUTER_BOUND ( 'NONE', #3033, .T. ) ;
#8464=CARTESIAN_POINT ( 'NONE',  ( 10.69346802281033959, 68.44840202376897764, 21.38693604562069339 ) ) ;
#8467=FACE_OUTER_BOUND ( 'NONE', #3200, .T. ) ;
#8469=FACE_OUTER_BOUND ( 'NONE', #4033, .T. ) ;
#8471=ORIENTED_EDGE ( 'NONE', *, *, #2528, .T. ) ;
#8472=ORIENTED_EDGE ( 'NONE', *, *, #2616, .F. ) ;
#8473=ORIENTED_EDGE ( 'NONE', *, *, #8155, .T. ) ;
#8474=CARTESIAN_POINT ( 'NONE',  ( 10.00000000000000000, 90.00000000000000000, 2.500000000000000000 ) ) ;
#8475=CARTESIAN_POINT ( 'NONE',  ( -2.179449471770338320, 90.00000000000000000, -4.500000000000000888 ) ) ;
#8476=AXIS2_PLACEMENT_3D ( 'NONE', #7604, #10627, #2141 ) ;
#8478=CARTESIAN_POINT ( 'NONE',  ( 12.97449437267218109, -39.59556244224027211, -25.94898874534434086 ) ) ;
#8479=ORIENTED_EDGE ( 'NONE', *, *, #7873, .T. ) ;
#8481=CARTESIAN_POINT ( 'NONE',  ( -1.341290363786561812E-15, 47.94714734142005597, -8.466779837416320124E-17 ) ) ;
#8482=CARTESIAN_POINT ( 'NONE',  ( -8.385254915620292238, 15.32944684068712782, -2.706960864746847057E-17 ) ) ;
#8483=DIRECTION ( 'NONE',  ( -1.000000000000000000, -2.835060530349835421E-17, 0.000000000000000000 ) ) ;
#8484=CARTESIAN_POINT ( 'NONE',  ( -8.385254915620294014, -15.56949922734665570, 2.749350679782564022E-17 ) ) ;
#8486=CARTESIAN_POINT ( 'NONE',  ( -0.7710117948378325536, -151.5922553772190895, -1.650848015692418569 ) ) ;
#8487=EDGE_CURVE ( 'NONE', #13048, #10681, #2654, .T. ) ;
#8489=EDGE_CURVE ( 'NONE', #4145, #4671, #2686, .T. ) ;
#8490=ORIENTED_EDGE ( 'NONE', *, *, #12699, .F. ) ;
#8495=CIRCLE ( 'NONE', #10723, 5.000000000000000000 ) ;
#8496=CARTESIAN_POINT ( 'NONE',  ( -10.69346802281034670, 40.17406817374066463, -1.451455445216333422E-15 ) ) ;
#8498=CARTESIAN_POINT ( 'NONE',  ( -3.034625339109073394, -118.9865377956984389, -4.388674898262355129 ) ) ;
#8499=CARTESIAN_POINT ( 'NONE',  ( -12.99553232110413781, -7.774801155466916747, -25.99106464220828627 ) ) ;
#8501=DIRECTION ( 'NONE',  ( -2.797435172181481150E-17, 1.000000000000000000, -1.765856845898762549E-18 ) ) ;
#8504=FACE_OUTER_BOUND ( 'NONE', #13415, .T. ) ;
#8505=AXIS2_PLACEMENT_3D ( 'NONE', #3414, #2438, #6446 ) ;
#8507=CARTESIAN_POINT ( 'NONE',  ( -10.00000000000000711, 139.9999999999999716, -0.5000000000000000000 ) ) ;
#8508=( BOUNDED_SURFACE ( )  B_SPLINE_SURFACE ( 3, 3, ( 
 ( #1484, #12501, #13381, #8997 ),
 ( #13526, #12292, #3731, #10324 ),
 ( #3865, #2682, #11367, #6050 ),
 ( #6251, #1904, #5121, #11443 ) ),
 .UNSPECIFIED., .F., .F., .T. ) 
 B_SPLINE_SURFACE_WITH_KNOTS ( ( 4, 4 ),
 ( 4, 4 ),
 ( 0.000000000000000000, 1.000000000000000000 ),
 ( 0.000000000000000000, 1.000000000000000000 ),
 .UNSPECIFIED. ) 
 GEOMETRIC_REPRESENTATION_ITEM ( )  RATIONAL_B_SPLINE_SURFACE ( (
 ( 1.000000000000000000, 0.3333333333333334259, 0.3333333333333334259, 1.000000000000000000),
 ( 1.000000000000000000, 0.3333333333333334259, 0.3333333333333334259, 1.000000000000000000),
 ( 1.000000000000000000, 0.3333333333333334259, 0.3333333333333334259, 1.000000000000000000),
 ( 1.000000000000000000, 0.3333333333333334259, 0.3333333333333334259, 1.000000000000000000) ) ) 
 REPRESENTATION_ITEM ( '' )  SURFACE ( )  );
#8510=EDGE_CURVE ( 'NONE', #1315, #10763, #4747, .T. ) ;
#8513=VERTEX_POINT ( 'NONE', #1701 ) ;
#8514=ORIENTED_EDGE ( 'NONE', *, *, #2211, .F. ) ;
#8515=VECTOR ( 'NONE', #11233, 1000.000000000000000 ) ;
#8516=CARTESIAN_POINT ( 'NONE',  ( 15.29705854078139282, -10.48808792804187284, 3.746698755667523200E-15 ) ) ;
#8520=CARTESIAN_POINT ( 'NONE',  ( 4.864544286455739552, -89.44155844152219004, 0.3495895964544955548 ) ) ;
#8523=FACE_OUTER_BOUND ( 'NONE', #862, .T. ) ;
#8525=AXIS2_PLACEMENT_3D ( 'NONE', #8613, #1316, #1190 ) ;
#8529=ORIENTED_EDGE ( 'NONE', *, *, #354, .T. ) ;
#8530=( BOUNDED_SURFACE ( )  B_SPLINE_SURFACE ( 3, 3, ( 
 ( #13001, #3368, #2383, #11926 ),
 ( #305, #6663, #9825, #4492 ),
 ( #10932, #4559, #1333, #5616 ),
 ( #8839, #13149, #4707, #8993 ) ),
 .UNSPECIFIED., .F., .F., .F. ) 
 B_SPLINE_SURFACE_WITH_KNOTS ( ( 4, 4 ),
 ( 4, 4 ),
 ( 0.000000000000000000, 1.000000000000000000 ),
 ( 0.000000000000000000, 1.000000000000000000 ),
 .UNSPECIFIED. ) 
 GEOMETRIC_REPRESENTATION_ITEM ( )  RATIONAL_B_SPLINE_SURFACE ( (
 ( 1.000000000000000000, 0.3333333333333334259, 0.3333333333333334259, 1.000000000000000000),
 ( 1.000000000000000000, 0.3333333333333334259, 0.3333333333333334259, 1.000000000000000000),
 ( 1.000000000000000000, 0.3333333333333334259, 0.3333333333333334259, 1.000000000000000000),
 ( 1.000000000000000000, 0.3333333333333334259, 0.3333333333333334259, 1.000000000000000000) ) ) 
 REPRESENTATION_ITEM ( '' )  SURFACE ( )  );
#8535=CARTESIAN_POINT ( 'NONE',  ( -15.29705854078139282, 55.48535772202409078, -9.797919878057798703E-17 ) ) ;
#8537=CARTESIAN_POINT ( 'NONE',  ( 10.69381717166375445, 53.83378072214353693, 2.619229793989003951E-15 ) ) ;
#8538=CARTESIAN_POINT ( 'NONE',  ( -0.7998255503467009975, -126.5099019064922743, -4.384466114569518957 ) ) ;
#8539=CYLINDRICAL_SURFACE ( 'NONE', #9386, 8.385254915620294014 ) ;
#8543=ORIENTED_EDGE ( 'NONE', *, *, #13758, .F. ) ;
#8545=VERTEX_POINT ( 'NONE', #2757 ) ;
#8547=CARTESIAN_POINT ( 'NONE',  ( 15.29705854078138749, 74.33491362204296138, 30.59411708156278564 ) ) ;
#8551=DIRECTION ( 'NONE',  ( 0.1234677578012386562, 1.701584941912606716E-18, -0.9923485843107423543 ) ) ;
#8552=DIRECTION ( 'NONE',  ( 0.000000000000000000, 1.000000000000000000, -0.000000000000000000 ) ) ;
#8553=CARTESIAN_POINT ( 'NONE',  ( -10.69381717166375623, 63.25855867215299355, -1.533026014780321478E-15 ) ) ;
#8555=EDGE_LOOP ( 'NONE', ( #940, #12556, #6847, #8598 ) ) ;
#8556=ORIENTED_EDGE ( 'NONE', *, *, #4364, .T. ) ;
#8558=EDGE_CURVE ( 'NONE', #7842, #4998, #2199, .T. ) ;
#8559=CARTESIAN_POINT ( 'NONE',  ( -2.179449471770338320, 90.00000000000000000, 4.500000000000000888 ) ) ;
#8560=ADVANCED_FACE ( 'NONE', ( #10187 ), #5109, .T. ) ;
#8562=LINE ( 'NONE', #10794, #754 ) ;
#8564=CARTESIAN_POINT ( 'NONE',  ( 6.895584828341370986, -94.56397396217489870, 4.654405414161209897 ) ) ;
#8566=AXIS2_PLACEMENT_3D ( 'NONE', #5178, #13775, #12695 ) ;
#8567=CARTESIAN_POINT ( 'NONE',  ( 0.3134609018104931866, -154.2164502171992240, -0.8036717672280221381 ) ) ;
#8571=AXIS2_PLACEMENT_3D ( 'NONE', #1875, #13631, #5100 ) ;
#8573=ADVANCED_FACE ( 'NONE', ( #8090 ), #7026, .T. ) ;
#8574=CARTESIAN_POINT ( 'NONE',  ( 1.024078386997840262, -80.66666666666725405, -9.976024522090996882 ) ) ;
#8575=DIRECTION ( 'NONE',  ( -1.000000000000000000, 0.000000000000000000, 0.000000000000000000 ) ) ;
#8576=CARTESIAN_POINT ( 'NONE',  ( 10.00000000000000000, 99.99999999999994316, 2.500000000000000000 ) ) ;
#8577=VECTOR ( 'NONE', #5256, 1000.000000000000000 ) ;
#8578=ORIENTED_EDGE ( 'NONE', *, *, #9954, .T. ) ;
#8583=EDGE_CURVE ( 'NONE', #12700, #1806, #41, .T. ) ;
#8584=CARTESIAN_POINT ( 'NONE',  ( -25.00000000000000355, 120.0000000000000284, -0.5000000000000000000 ) ) ;
#8586=ORIENTED_EDGE ( 'NONE', *, *, #13434, .T. ) ;
#8588=FACE_OUTER_BOUND ( 'NONE', #13668, .T. ) ;
#8589=EDGE_CURVE ( 'NONE', #6325, #6913, #12063, .T. ) ;
#8590=CARTESIAN_POINT ( 'NONE',  ( 12.09338464843078675, -169.0000000000000000, -0.006909782850910250844 ) ) ;
#8593=CARTESIAN_POINT ( 'NONE',  ( 10.69346802281034847, 11.89973432371241202, -21.38693604562068629 ) ) ;
#8595=DIRECTION ( 'NONE',  ( -0.000000000000000000, -0.000000000000000000, -1.000000000000000000 ) ) ;
#8596=VERTEX_POINT ( 'NONE', #19 ) ;
#8598=ORIENTED_EDGE ( 'NONE', *, *, #1741, .F. ) ;
#8599=CARTESIAN_POINT ( 'NONE',  ( -15.29705854078138749, 46.06057977201469100, -30.59411708156277854 ) ) ;
#8601=ADVANCED_FACE ( 'NONE', ( #10850 ), #5747, .T. ) ;
#8602=AXIS2_PLACEMENT_3D ( 'NONE', #9063, #13379, #3728 ) ;
#8603=DIRECTION ( 'NONE',  ( -0.000000000000000000, -0.000000000000000000, -1.000000000000000000 ) ) ;
#8606=CARTESIAN_POINT ( 'NONE',  ( 8.385254915620292238, 90.00000000000000000, 8.679704431140118580E-16 ) ) ;
#8607=ORIENTED_EDGE ( 'NONE', *, *, #9722, .F. ) ;
#8608=( BOUNDED_SURFACE ( )  B_SPLINE_SURFACE ( 3, 3, ( 
 ( #13866, #8433, #5135, #7438 ),
 ( #8496, #9354, #9558, #2110 ),
 ( #13737, #7169, #11592, #12723 ),
 ( #12591, #1846, #6261, #8364 ) ),
 .UNSPECIFIED., .F., .F., .T. ) 
 B_SPLINE_SURFACE_WITH_KNOTS ( ( 4, 4 ),
 ( 4, 4 ),
 ( 0.000000000000000000, 1.000000000000000000 ),
 ( 0.000000000000000000, 1.000000000000000000 ),
 .UNSPECIFIED. ) 
 GEOMETRIC_REPRESENTATION_ITEM ( )  RATIONAL_B_SPLINE_SURFACE ( (
 ( 1.000000000000000000, 0.3333333333333334259, 0.3333333333333334259, 1.000000000000000000),
 ( 1.000000000000000000, 0.3333333333333334259, 0.3333333333333334259, 1.000000000000000000),
 ( 1.000000000000000000, 0.3333333333333334259, 0.3333333333333334259, 1.000000000000000000),
 ( 1.000000000000000000, 0.3333333333333334259, 0.3333333333333334259, 1.000000000000000000) ) ) 
 REPRESENTATION_ITEM ( '' )  SURFACE ( )  );
#8609=VECTOR ( 'NONE', #1350, 1000.000000000000000 ) ;
#8610=ORIENTED_EDGE ( 'NONE', *, *, #13336, .F. ) ;
#8613=CARTESIAN_POINT ( 'NONE',  ( -6.924833908958124424E-16, 24.75422479069652582, -4.371241731156832241E-17 ) ) ;
#8615=CARTESIAN_POINT ( 'NONE',  ( -6.174202239351583188, -74.54647412380100491, -8.025911163902851087 ) ) ;
#8616=DIRECTION ( 'NONE',  ( -1.000000000000000000, 0.000000000000000000, 0.000000000000000000 ) ) ;
#8618=CARTESIAN_POINT ( 'NONE',  ( -2.799701502495941963, -101.5643811721427738, -6.922737930671543971 ) ) ;
#8619=CARTESIAN_POINT ( 'NONE',  ( -0.9875499244693202172, -80.00464164737402939, 10.06307371418729701 ) ) ;
#8621=VERTEX_POINT ( 'NONE', #13366 ) ;
#8624=ORIENTED_EDGE ( 'NONE', *, *, #190, .F. ) ;
#8625=AXIS2_PLACEMENT_3D ( 'NONE', #7945, #1418, #5915 ) ;
#8626=CARTESIAN_POINT ( 'NONE',  ( -3.629742700906668951, 90.29727615934677942, 3.441963681523289242 ) ) ;
#8627=LINE ( 'NONE', #12932, #5154 ) ;
#8628=ORIENTED_EDGE ( 'NONE', *, *, #11589, .T. ) ;
#8629=CARTESIAN_POINT ( 'NONE',  ( -38.80000000000001137, 101.5999999999999943, 0.5000000000000000000 ) ) ;
#8630=CIRCLE ( 'NONE', #7297, 5.000000000000000000 ) ;
#8632=CARTESIAN_POINT ( 'NONE',  ( -12.99553232110414491, 1.649976794542511893, -1.597320951662050367E-15 ) ) ;
#8633=CARTESIAN_POINT ( 'NONE',  ( -3.510313888878303423, -133.0909090908702126, 1.034921094667177410 ) ) ;
#8636=CARTESIAN_POINT ( 'NONE',  ( 0.2677229415529756018, -160.9696969707963774, -0.7106593571500791073 ) ) ;
#8637=CIRCLE ( 'NONE', #11771, 15.29705854078139105 ) ;
#8638=CARTESIAN_POINT ( 'NONE',  ( -7.500230552170997100, -73.18181818181757592, -6.960552780978341403 ) ) ;
#8642=ADVANCED_FACE ( 'NONE', ( #12137 ), #7184, .T. ) ;
#8643=EDGE_LOOP ( 'NONE', ( #6011, #9237, #11112, #5056 ) ) ;
#8644=CIRCLE ( 'NONE', #154, 2.000000000000000000 ) ;
#8645=CARTESIAN_POINT ( 'NONE',  ( -2.303009741871944172E-17, 0.8232575913728890082, -1.453755053663958216E-18 ) ) ;
#8649=FACE_OUTER_BOUND ( 'NONE', #1570, .T. ) ;
#8654=CARTESIAN_POINT ( 'NONE',  ( -15.29705854078138927, 55.48535772202409788, -30.59411708156277854 ) ) ;
#8656=CARTESIAN_POINT ( 'NONE',  ( 10.69381717166375623, 25.55944687211528077, 1.274859266482038215E-15 ) ) ;
#8661=ADVANCED_FACE ( 'NONE', ( #5746 ), #1277, .T. ) ;
#8662=CYLINDRICAL_SURFACE ( 'NONE', #13006, 40.00000000000001421 ) ;
#8665=ADVANCED_FACE ( 'NONE', ( #1687 ), #2809, .T. ) ;
#8667=ORIENTED_EDGE ( 'NONE', *, *, #12038, .T. ) ;
#8673=EDGE_CURVE ( 'NONE', #2108, #3901, #13443, .T. ) ;
#8674=CARTESIAN_POINT ( 'NONE',  ( 15.29705854078138216, 10.24803554138234318, 30.59411708156277498 ) ) ;
#8677=EDGE_CURVE ( 'NONE', #4998, #3518, #12962, .T. ) ;
#8680=DIRECTION ( 'NONE',  ( -1.000000000000000000, 0.000000000000000000, 0.000000000000000000 ) ) ;
#8681=ORIENTED_EDGE ( 'NONE', *, *, #6212, .F. ) ;
#8682=CARTESIAN_POINT ( 'NONE',  ( -2.237684797877294057E-15, 79.99058638175036151, -1.412519245696701404E-16 ) ) ;
#8684=FACE_OUTER_BOUND ( 'NONE', #10749, .T. ) ;
#8687=CARTESIAN_POINT ( 'NONE',  ( 3.828023344975119535, 90.45717703472961091, -3.219997411495246098 ) ) ;
#8688=CARTESIAN_POINT ( 'NONE',  ( 0.9252956712946845963, -80.77513221109299479, 9.969903607383971078 ) ) ;
#8690=ORIENTED_EDGE ( 'NONE', *, *, #13865, .F. ) ;
#8692=ORIENTED_EDGE ( 'NONE', *, *, #6118, .T. ) ;
#8695=ORIENTED_EDGE ( 'NONE', *, *, #13218, .F. ) ;
#8697=SURFACE_STYLE_FILL_AREA ( #7576 ) ;
#8702=CARTESIAN_POINT ( 'NONE',  ( -9.841115069317030617, -69.87878787878872799, -2.624300023644856150 ) ) ;
#8712=DIRECTION ( 'NONE',  ( -0.8000000000000008216, -0.5999999999999988676, -0.000000000000000000 ) ) ;
#8716=AXIS2_PLACEMENT_3D ( 'NONE', #7253, #751, #13618 ) ;
#8717=DIRECTION ( 'NONE',  ( 0.000000000000000000, 0.000000000000000000, -1.000000000000000000 ) ) ;
#8726=AXIS2_PLACEMENT_3D ( 'NONE', #8645, #7658, #9701 ) ;
#8729=ORIENTED_EDGE ( 'NONE', *, *, #11995, .F. ) ;
#8730=LINE ( 'NONE', #4596, #9207 ) ;
#8731=ORIENTED_EDGE ( 'NONE', *, *, #10531, .F. ) ;
#8736=EDGE_CURVE ( 'NONE', #2229, #4279, #13843, .T. ) ;
#8737=EDGE_LOOP ( 'NONE', ( #3197, #1220, #440, #8913, #2995 ) ) ;
#8738=CARTESIAN_POINT ( 'NONE',  ( -2.866821506922881722E-16, 10.24803554138234496, -1.809656371776380929E-17 ) ) ;
#8740=AXIS2_PLACEMENT_3D ( 'NONE', #2332, #8785, #1225 ) ;
#8743=EDGE_CURVE ( 'NONE', #7988, #13719, #10576, .T. ) ;
#8744=DIRECTION ( 'NONE',  ( -2.797435172181481150E-17, 1.000000000000000000, -1.765856845898762549E-18 ) ) ;
#8746=ORIENTED_EDGE ( 'NONE', *, *, #5929, .F. ) ;
#8747=AXIS2_PLACEMENT_3D ( 'NONE', #6310, #9193, #10839 ) ;
#8749=CARTESIAN_POINT ( 'NONE',  ( 8.385254915620288685, 53.02855864072483882, 9.355740606675293587E-16 ) ) ;
#8751=EDGE_LOOP ( 'NONE', ( #589, #12539, #1590, #4229 ) ) ;
#8753=DIRECTION ( 'NONE',  ( 0.000000000000000000, 0.000000000000000000, -1.000000000000000000 ) ) ;
#8754=CARTESIAN_POINT ( 'NONE',  ( 41.99999999999999289, 120.0000000000000284, -0.5000000000000000000 ) ) ;
#8759=CARTESIAN_POINT ( 'NONE',  ( -3.408847948936934547, -84.09052683291464803, 8.956775459301910658 ) ) ;
#8760=CARTESIAN_POINT ( 'NONE',  ( 15.29705854078139105, 27.21102387199583816, 1.823632900916640874E-15 ) ) ;
#8762=VERTEX_POINT ( 'NONE', #2948 ) ;
#8770=CARTESIAN_POINT ( 'NONE',  ( 15.29705854078138749, 57.37192529142945574, 1.773704474924340737E-15 ) ) ;
#8772=CARTESIAN_POINT ( 'NONE',  ( 1.956031471770903973, -154.2164502167725857, 1.283490743971270831 ) ) ;
#8776=CARTESIAN_POINT ( 'NONE',  ( -0.9402774206043360561, -80.12121212121206781, -9.996606859377621390 ) ) ;
#8781=CARTESIAN_POINT ( 'NONE',  ( 8.385254915620288685, 71.87811454074363837, -16.77050983124057382 ) ) ;
#8783=VECTOR ( 'NONE', #2201, 1000.000000000000000 ) ;
#8785=DIRECTION ( 'NONE',  ( -2.797435172181481150E-17, 1.000000000000000000, -1.765856845898762549E-18 ) ) ;
#8786=ORIENTED_EDGE ( 'NONE', *, *, #9317, .T. ) ;
#8787=AXIS2_PLACEMENT_3D ( 'NONE', #9926, #10069, #4746 ) ;
#8788=DIRECTION ( 'NONE',  ( 1.000000000000000000, 2.797435172181480534E-17, 0.000000000000000000 ) ) ;
#8790=DIRECTION ( 'NONE',  ( -2.797435172181481150E-17, 1.000000000000000000, -1.765856845898762549E-18 ) ) ;
#8791=CARTESIAN_POINT ( 'NONE',  ( -15.29705854078139637, 0.8232575913729158756, -1.876256887941090008E-15 ) ) ;
#8793=CARTESIAN_POINT ( 'NONE',  ( -8.385254915620292238, -3.520109059331727686, 6.216008680731233110E-18 ) ) ;
#8807=DIRECTION ( 'NONE',  ( 1.000000000000000000, 0.000000000000000000, 0.000000000000000000 ) ) ;
#8808=CARTESIAN_POINT ( 'NONE',  ( 8.385254915620290461, 53.02855864072483882, 2.053795118489800004E-15 ) ) ;
#8812=ADVANCED_FACE ( 'NONE', ( #8469 ), #6038, .T. ) ;
#8814=ADVANCED_FACE ( 'NONE', ( #13643 ), #3990, .T. ) ;
#8815=CARTESIAN_POINT ( 'NONE',  ( 15.29705854078138927, 29.09759144140119957, 1.823632900916640086E-15 ) ) ;
#8817=ORIENTED_EDGE ( 'NONE', *, *, #4700, .T. ) ;
#8819=CARTESIAN_POINT ( 'NONE',  ( 8.385254915620281579, 71.87811454074363837, 16.77050983124057737 ) ) ;
#8820=AXIS2_PLACEMENT_3D ( 'NONE', #9448, #13693, #7465 ) ;
#8823=CARTESIAN_POINT ( 'NONE',  ( 8.385254915620292238, -12.94488700934118341, 1.052073721316228694E-15 ) ) ;
#8825=CARTESIAN_POINT ( 'NONE',  ( -0.9919461901367589984, -82.18142821831455080, 9.724687322501905484 ) ) ;
#8829=ORIENTED_EDGE ( 'NONE', *, *, #6549, .T. ) ;
#8832=CIRCLE ( 'NONE', #5467, 2.000000000000003997 ) ;
#8833=EDGE_CURVE ( 'NONE', #1472, #7475, #6027, .T. ) ;
#8835=CARTESIAN_POINT ( 'NONE',  ( -4.230699918504780221, 91.18539124371005755, 2.666380740812165584 ) ) ;
#8839=CARTESIAN_POINT ( 'NONE',  ( -8.385254915620292238, 34.17900274070598243, -1.147608011196236061E-15 ) ) ;
#8840=CARTESIAN_POINT ( 'NONE',  ( -6.190615655759536180E-16, 22.12961257269105531, -3.907772785857374249E-17 ) ) ;
#8841=CARTESIAN_POINT ( 'NONE',  ( -0.2890385494233511099, -128.7272727272755048, 4.499839249777335404 ) ) ;
#8842=CARTESIAN_POINT ( 'NONE',  ( -2.079471018873752021E-15, 74.33491362204294717, -1.312648161087776599E-16 ) ) ;
#8843=CARTESIAN_POINT ( 'NONE',  ( 12.99553232110414669, -17.19957910547634228, 1.630511914918685592E-15 ) ) ;
#8844=AXIS2_PLACEMENT_3D ( 'NONE', #3114, #11740, #10421 ) ;
#8845=DIRECTION ( 'NONE',  ( -2.797435172181481150E-17, 1.000000000000000000, -1.765856845898762549E-18 ) ) ;
#8846=DIRECTION ( 'NONE',  ( -1.000000000000000000, 0.000000000000000000, 0.000000000000000000 ) ) ;
#8848=CIRCLE ( 'NONE', #9088, 5.000000000000000000 ) ;
#8850=AXIS2_PLACEMENT_3D ( 'NONE', #8219, #10594, #7163 ) ;
#8851=ADVANCED_FACE ( 'NONE', ( #4528 ), #5575, .T. ) ;
#8853=ORIENTED_EDGE ( 'NONE', *, *, #8510, .T. ) ;
#8854=DIRECTION ( 'NONE',  ( -0.000000000000000000, -0.000000000000000000, -1.000000000000000000 ) ) ;
#8862=ORIENTED_EDGE ( 'NONE', *, *, #5229, .F. ) ;
#8863=CARTESIAN_POINT ( 'NONE',  ( 8.385254915620294014, -15.56949922734665570, 1.052073721316228694E-15 ) ) ;
#8865=AXIS2_PLACEMENT_3D ( 'NONE', #8170, #8307, #748 ) ;
#8867=CARTESIAN_POINT ( 'NONE',  ( 8.385254915620294014, 24.75422479069652582, 2.053795118489800793E-15 ) ) ;
#8869=ADVANCED_FACE ( 'NONE', ( #6371 ), #8539, .T. ) ;
#8872=CARTESIAN_POINT ( 'NONE',  ( -9.943536534200680066, -71.42980831791368246, -1.832023084373848532 ) ) ;
#8874=CIRCLE ( 'NONE', #11339, 15.29705854078139282 ) ;
#8875=DIRECTION ( 'NONE',  ( -2.797435172181481150E-17, 1.000000000000000000, -1.765856845898762549E-18 ) ) ;
#8876=CARTESIAN_POINT ( 'NONE',  ( -10.69381717166375623, 16.13466892210585613, -1.366597928139322991E-15 ) ) ;
#8878=DIRECTION ( 'NONE',  ( -0.000000000000000000, -0.000000000000000000, -1.000000000000000000 ) ) ;
#8879=EDGE_LOOP ( 'NONE', ( #4825, #7392, #8023, #12106 ) ) ;
#8881=AXIS2_PLACEMENT_3D ( 'NONE', #4253, #8603, #11897 ) ;
#8882=B_SPLINE_CURVE_WITH_KNOTS ( 'NONE', 3,
 ( #150, #12046, #12982, #8749 ),
 .UNSPECIFIED., .F., .F.,
 ( 4, 4 ),
 ( 0.000000000000000000, 1.000000000000000000 ),
 .UNSPECIFIED. ) ;
#8896=ORIENTED_EDGE ( 'NONE', *, *, #11057, .T. ) ;
#8902=DIRECTION ( 'NONE',  ( -1.000000000000000000, 0.000000000000000000, 0.000000000000000000 ) ) ;
#8904=DIRECTION ( 'NONE',  ( -1.000000000000000000, 0.000000000000000000, 0.000000000000000000 ) ) ;
#8906=CARTESIAN_POINT ( 'NONE',  ( -8.385254915620295790, 59.82872437272870769, 16.77050983124058092 ) ) ;
#8912=CARTESIAN_POINT ( 'NONE',  ( -10.00000000000000000, 99.99999999999994316, 0.5000000000000000000 ) ) ;
#8913=ORIENTED_EDGE ( 'NONE', *, *, #4759, .F. ) ;
#8914=CARTESIAN_POINT ( 'NONE',  ( 8.385254915620292238, -24.99427717735608567, 16.77050983124059158 ) ) ;
#8915=DIRECTION ( 'NONE',  ( -2.797435172181481150E-17, 1.000000000000000000, -1.765856845898762549E-18 ) ) ;
#8916=EDGE_LOOP ( 'NONE', ( #8430, #12572, #13059, #5439 ) ) ;
#8917=CARTESIAN_POINT ( 'NONE',  ( 1.087924128445332483, -78.56626503148619634, 10.04922990102044622 ) ) ;
#8919=CARTESIAN_POINT ( 'NONE',  ( -12.99553232110413425, 58.19864449459908684, -25.99106464220827561 ) ) ;
#8920=ADVANCED_FACE ( 'NONE', ( #5376 ), #3343, .T. ) ;
#8923=DIRECTION ( 'NONE',  ( -2.797435172181481150E-17, 1.000000000000000000, -1.765856845898762549E-18 ) ) ;
#8924=CARTESIAN_POINT ( 'NONE',  ( -2.264596963716165146, -106.9090909090919013, 6.916633125701347140 ) ) ;
#8928=EDGE_CURVE ( 'NONE', #9797, #2621, #4325, .T. ) ;
#8931=VERTEX_POINT ( 'NONE', #6571 ) ;
#8933=VECTOR ( 'NONE', #6177, 1000.000000000000000 ) ;
#8937=DIRECTION ( 'NONE',  ( 1.000000000000000000, 0.000000000000000000, 0.000000000000000000 ) ) ;
#8941=LINE ( 'NONE', #5421, #2933 ) ;
#8943=CARTESIAN_POINT ( 'NONE',  ( 10.69346802281034847, -16.37459952631584059, 0.000000000000000000 ) ) ;
#8944=ORIENTED_EDGE ( 'NONE', *, *, #6118, .F. ) ;
#8951=CARTESIAN_POINT ( 'NONE',  ( -4.789632183893028028, -77.94522261687450282, -8.921723405160534526 ) ) ;
#8954=CARTESIAN_POINT ( 'NONE',  ( -15.29705854078138749, -36.87585420866476227, 6.511747960273540061E-17 ) ) ;
#8955=CARTESIAN_POINT ( 'NONE',  ( -10.69381717166375800, 16.13466892210585257, 21.38763434332750890 ) ) ;
#8956=DIRECTION ( 'NONE',  ( -1.000000000000000000, 0.000000000000000000, 0.000000000000000000 ) ) ;
#8957=CARTESIAN_POINT ( 'NONE',  ( 3.632360187558549836, 90.29910261214918421, 3.439149220787172556 ) ) ;
#8961=CIRCLE ( 'NONE', #3126, 15.29705854078138927 ) ;
#8962=ORIENTED_EDGE ( 'NONE', *, *, #13583, .T. ) ;
#8964=ORIENTED_EDGE ( 'NONE', *, *, #6269, .T. ) ;
#8965=CARTESIAN_POINT ( 'NONE',  ( 1.718945942447514764E-16, -6.144721277337255927, 1.085069813372578838E-17 ) ) ;
#8970=FACE_OUTER_BOUND ( 'NONE', #3946, .T. ) ;
#8971=ORIENTED_EDGE ( 'NONE', *, *, #10707, .T. ) ;
#8974=TOROIDAL_SURFACE ( 'NONE', #10747, 22.99999999999999289, 2.000000000000000000 ) ;
#8975=ORIENTED_EDGE ( 'NONE', *, *, #5951, .T. ) ;
#8976=CARTESIAN_POINT ( 'NONE',  ( -10.69346802281034137, -35.22415542633469698, -21.38693604562069694 ) ) ;
#8978=CARTESIAN_POINT ( 'NONE',  ( -9.515638016687521628, -70.53215316236570231, -3.421011903893942829 ) ) ;
#8979=CARTESIAN_POINT ( 'NONE',  ( 25.00000000000000355, 120.0000000000000284, 2.500000000000000000 ) ) ;
#8980=CARTESIAN_POINT ( 'NONE',  ( -1.798319979498498977, -80.15852057206338088, -9.967197727661469386 ) ) ;
#8982=CARTESIAN_POINT ( 'NONE',  ( 12.99579180576516713, 16.95961992694555676, -25.99158361153032004 ) ) ;
#8985=EDGE_CURVE ( 'NONE', #12700, #7874, #13425, .T. ) ;
#8986=CARTESIAN_POINT ( 'NONE',  ( 8.385254915620294014, -6.144721277337255039, 16.77050983124059513 ) ) ;
#8990=( BOUNDED_SURFACE ( )  B_SPLINE_SURFACE ( 3, 3, ( 
 ( #11605, #4100, #10553, #8516 ),
 ( #13817, #6282, #13882, #5351 ),
 ( #1091, #7256, #12675, #4165 ),
 ( #9373, #1864, #11672, #7323 ) ),
 .UNSPECIFIED., .F., .F., .T. ) 
 B_SPLINE_SURFACE_WITH_KNOTS ( ( 4, 4 ),
 ( 4, 4 ),
 ( 0.000000000000000000, 1.000000000000000000 ),
 ( 0.000000000000000000, 1.000000000000000000 ),
 .UNSPECIFIED. ) 
 GEOMETRIC_REPRESENTATION_ITEM ( )  RATIONAL_B_SPLINE_SURFACE ( (
 ( 1.000000000000000000, 0.3333333333333334259, 0.3333333333333334259, 1.000000000000000000),
 ( 1.000000000000000000, 0.3333333333333334259, 0.3333333333333334259, 1.000000000000000000),
 ( 1.000000000000000000, 0.3333333333333334259, 0.3333333333333334259, 1.000000000000000000),
 ( 1.000000000000000000, 0.3333333333333334259, 0.3333333333333334259, 1.000000000000000000) ) ) 
 REPRESENTATION_ITEM ( '' )  SURFACE ( )  );
#8992=CARTESIAN_POINT ( 'NONE',  ( 5.215657008045057275, -75.40994149440513183, 8.686150177547775186 ) ) ;
#8993=CARTESIAN_POINT ( 'NONE',  ( 8.385254915620290461, 34.17900274070598243, 2.053795118489799610E-15 ) ) ;
#8994=AXIS2_PLACEMENT_3D ( 'NONE', #11595, #8501, #12800 ) ;
#8997=CARTESIAN_POINT ( 'NONE',  ( 15.29705854078139105, 46.06057977201469100, 3.746698755667522411E-15 ) ) ;
#8998=CARTESIAN_POINT ( 'NONE',  ( -12.99553232110413781, -17.19957910547634228, -25.99106464220828627 ) ) ;
#8999=CARTESIAN_POINT ( 'NONE',  ( 2.733214920032663198, -81.93939393936486226, -9.473759075839289778 ) ) ;
#9001=CARTESIAN_POINT ( 'NONE',  ( -2.517691654963332357E-15, 90.00000000000000000, -1.589271161308885878E-16 ) ) ;
#9004=DIRECTION ( 'NONE',  ( -0.8000000000000008216, 0.5999999999999988676, 0.000000000000000000 ) ) ;
#9006=EDGE_CURVE ( 'NONE', #8407, #8282, #11397, .T. ) ;
#9007=CARTESIAN_POINT ( 'NONE',  ( -3.317295986488982162, -135.2979454323821358, -0.9176727334396277413 ) ) ;
#9008=EDGE_CURVE ( 'NONE', #4633, #11439, #2530, .T. ) ;
#9010=DIRECTION ( 'NONE',  ( -1.000000000000000000, 0.000000000000000000, 0.000000000000000000 ) ) ;
#9011=EDGE_CURVE ( 'NONE', #1806, #10192, #11401, .T. ) ;
#9012=VERTEX_POINT ( 'NONE', #5732 ) ;
#9014=ORIENTED_EDGE ( 'NONE', *, *, #8558, .F. ) ;
#9015=CARTESIAN_POINT ( 'NONE',  ( 1.692320366844926705, -139.6713384906986448, 2.426530036419475511 ) ) ;
#9016=DIRECTION ( 'NONE',  ( 1.000000000000000000, 0.000000000000000000, 0.000000000000000000 ) ) ;
#9022=CARTESIAN_POINT ( 'NONE',  ( 15.29705854078139282, 64.91013567203349055, 3.746698755667523989E-15 ) ) ;
#9023=DIRECTION ( 'NONE',  ( -2.797435172181481150E-17, 1.000000000000000000, -1.765856845898762549E-18 ) ) ;
#9024=ORIENTED_EDGE ( 'NONE', *, *, #4122, .F. ) ;
#9026=ADVANCED_FACE ( 'NONE', ( #4764 ), #634, .T. ) ;
#9027=CARTESIAN_POINT ( 'NONE',  ( -4.864544286455551259, -89.44155844152571433, -0.3495895964559158076 ) ) ;
#9028=ADVANCED_FACE ( 'NONE', ( #8970 ), #13330, .T. ) ;
#9029=ORIENTED_EDGE ( 'NONE', *, *, #4122, .T. ) ;
#9030=ADVANCED_FACE ( 'NONE', ( #12548 ), #11615, .T. ) ;
#9032=VERTEX_POINT ( 'NONE', #6230 ) ;
#9033=CARTESIAN_POINT ( 'NONE',  ( -0.2321914886085471308, -147.1038961038843524, 14.56966866480940226 ) ) ;
#9036=CARTESIAN_POINT ( 'NONE',  ( 8.385254915620299343, -34.41905512736551032, 2.053795118489801582E-15 ) ) ;
#9037=CARTESIAN_POINT ( 'NONE',  ( -2.517691654963332357E-15, 90.00000000000000000, -1.589271161308885878E-16 ) ) ;
#9040=EDGE_CURVE ( 'NONE', #12557, #8513, #3509, .T. ) ;
#9043=EDGE_CURVE ( 'NONE', #13719, #1890, #9566, .T. ) ;
#9047=MECHANICAL_DESIGN_GEOMETRIC_PRESENTATION_REPRESENTATION('',(#5015),#12182);
#9049=( BOUNDED_SURFACE ( )  B_SPLINE_SURFACE ( 3, 3, ( 
 ( #5816, #2736, #10234, #7993 ),
 ( #4770, #10097, #8976, #9952 ),
 ( #9116, #13432, #11219, #13505 ),
 ( #1609, #13360, #12272, #7004 ) ),
 .UNSPECIFIED., .F., .F., .F. ) 
 B_SPLINE_SURFACE_WITH_KNOTS ( ( 4, 4 ),
 ( 4, 4 ),
 ( 0.000000000000000000, 1.000000000000000000 ),
 ( 0.000000000000000000, 1.000000000000000000 ),
 .UNSPECIFIED. ) 
 GEOMETRIC_REPRESENTATION_ITEM ( )  RATIONAL_B_SPLINE_SURFACE ( (
 ( 1.000000000000000000, 0.3333333333333334259, 0.3333333333333334259, 1.000000000000000000),
 ( 1.000000000000000000, 0.3333333333333334259, 0.3333333333333334259, 1.000000000000000000),
 ( 1.000000000000000000, 0.3333333333333334259, 0.3333333333333334259, 1.000000000000000000),
 ( 1.000000000000000000, 0.3333333333333334259, 0.3333333333333334259, 1.000000000000000000) ) ) 
 REPRESENTATION_ITEM ( '' )  SURFACE ( )  );
#9051=CARTESIAN_POINT ( 'NONE',  ( 3.767919204793307220, -84.38294504924263606, -8.813286018183102755 ) ) ;
#9052=CARTESIAN_POINT ( 'NONE',  ( -10.69346802281035025, 59.02362407375952102, 21.38693604562068629 ) ) ;
#9055=ORIENTED_EDGE ( 'NONE', *, *, #6956, .T. ) ;
#9056=CARTESIAN_POINT ( 'NONE',  ( -8.621450369311798312, -91.42953101131953986, -1.276853297472915649 ) ) ;
#9062=CARTESIAN_POINT ( 'NONE',  ( 4.696484759529488962, 90.40938722714874132, 1.719265504264336109 ) ) ;
#9063=CARTESIAN_POINT ( 'NONE',  ( -2.132246523607266586E-15, 76.22148119144830503, -1.345962243664627229E-16 ) ) ;
#9064=CARTESIAN_POINT ( 'NONE',  ( 3.371721678969648917, -122.9090909090891728, 4.477688567679800613 ) ) ;
#9066=CARTESIAN_POINT ( 'NONE',  ( -1.693173457972974028, -102.5454545454559110, 7.725659299994978468 ) ) ;
#9075=CIRCLE ( 'NONE', #10194, 15.29705854078139105 ) ;
#9076=ORIENTED_EDGE ( 'NONE', *, *, #211, .T. ) ;
#9077=CARTESIAN_POINT ( 'NONE',  ( -2.816776700191196081, -98.83340855854847007, -7.314626998258005663 ) ) ;
#9081=EDGE_LOOP ( 'NONE', ( #7640, #7991, #3179, #6188 ) ) ;
#9083=VERTEX_POINT ( 'NONE', #13701 ) ;
#9084=DIRECTION ( 'NONE',  ( 1.000000000000000000, 0.000000000000000000, 0.000000000000000000 ) ) ;
#9086=CARTESIAN_POINT ( 'NONE',  ( 2.535732011270894759, -137.7254863561949492, 1.949617200014976071 ) ) ;
#9087=CARTESIAN_POINT ( 'NONE',  ( 10.00000000000000711, 139.9999999999999716, 0.5000000000000000000 ) ) ;
#9088=AXIS2_PLACEMENT_3D ( 'NONE', #5405, #4016, #8299 ) ;
#9093=CARTESIAN_POINT ( 'NONE',  ( 10.69381717166374735, 63.25855867215300066, 21.38763434332750890 ) ) ;
#9094=DIRECTION ( 'NONE',  ( -1.000000000000000000, 0.000000000000000000, 0.000000000000000000 ) ) ;
#9096=CARTESIAN_POINT ( 'NONE',  ( -10.43546891138450228, -95.36363636363145702, -7.899666394170180794 ) ) ;
#9097=CIRCLE ( 'NONE', #2357, 15.29705854078138749 ) ;
#9098=ORIENTED_EDGE ( 'NONE', *, *, #6026, .F. ) ;
#9102=AXIS2_PLACEMENT_3D ( 'NONE', #1613, #4545, #8904 ) ;
#9103=CARTESIAN_POINT ( 'NONE',  ( -12.99579180576516713, 35.80917582696438473, -3.253142430666311955E-15 ) ) ;
#9106=CARTESIAN_POINT ( 'NONE',  ( 12.99579180576516713, -20.73949187309215247, 25.99158361153034491 ) ) ;
#9112=EDGE_CURVE ( 'NONE', #8398, #4279, #876, .T. ) ;
#9116=CARTESIAN_POINT ( 'NONE',  ( 12.99553232110414314, -36.04913500549519512, 1.682098219708385520E-15 ) ) ;
#9117=FACE_OUTER_BOUND ( 'NONE', #7420, .T. ) ;
#9119=CARTESIAN_POINT ( 'NONE',  ( -8.558795028186576559, -72.03745728540356197, -5.439008160060279984 ) ) ;
#9121=CARTESIAN_POINT ( 'NONE',  ( -4.426053706385205899, -109.9138289782734432, 4.721619936386206362 ) ) ;
#9124=EDGE_CURVE ( 'NONE', #11499, #149, #9821, .T. ) ;
#9126=CARTESIAN_POINT ( 'NONE',  ( 8.385254915620297567, -6.144721277337255927, 2.053795118489801582E-15 ) ) ;
#9128=CARTESIAN_POINT ( 'NONE',  ( -0.1768551147989557704, -79.21212121212170132, 10.18346664538817770 ) ) ;
#9129=ORIENTED_EDGE ( 'NONE', *, *, #9671, .F. ) ;
#9130=CARTESIAN_POINT ( 'NONE',  ( 6.174202269517973463, -74.54647409589566109, 8.025911141045913411 ) ) ;
#9132=CARTESIAN_POINT ( 'NONE',  ( 10.00000000000000711, 139.9999999999999716, 2.500000000000000000 ) ) ;
#9134=CARTESIAN_POINT ( 'NONE',  ( 0.2714810715513833461, -148.3982683985791198, 1.717521498777542455 ) ) ;
#9140=CARTESIAN_POINT ( 'NONE',  ( 8.385254915620292238, 15.32944684068712782, 1.002145295323929148E-15 ) ) ;
#9142=CARTESIAN_POINT ( 'NONE',  ( -3.045952509441874678, -136.2549498598916671, -1.356822578832249215 ) ) ;
#9143=CARTESIAN_POINT ( 'NONE',  ( 1.119237408740483274E-15, -40.00941361824966691, 7.065089693818133469E-17 ) ) ;
#9145=CYLINDRICAL_SURFACE ( 'NONE', #4046, 15.29705854078139815 ) ;
#9147=ORIENTED_EDGE ( 'NONE', *, *, #9804, .F. ) ;
#9149=CARTESIAN_POINT ( 'NONE',  ( 3.311736046961211155, -135.3203766226484674, 0.9286747277042636250 ) ) ;
#9150=FACE_OUTER_BOUND ( 'NONE', #13368, .T. ) ;
#9157=CARTESIAN_POINT ( 'NONE',  ( 3.163850051431341015, 90.09728930184206774, 3.875191615614280494 ) ) ;
#9159=CARTESIAN_POINT ( 'NONE',  ( 15.29705854078139460, -27.45107625865536605, 1.923489752901240361E-15 ) ) ;
#9163=DIRECTION ( 'NONE',  ( 1.000000000000000000, 0.000000000000000000, 0.000000000000000000 ) ) ;
#9165=CARTESIAN_POINT ( 'NONE',  ( 10.69381717166375800, 34.98422482212468054, -21.38763434332750890 ) ) ;
#9173=EDGE_CURVE ( 'NONE', #9032, #3017, #7143, .T. ) ;
#9174=CARTESIAN_POINT ( 'NONE',  ( -6.361701577163668020, -84.44507371548807839, 7.124205211947466587 ) ) ;
#9175=EDGE_CURVE ( 'NONE', #11958, #10177, #13894, .T. ) ;
#9176=VECTOR ( 'NONE', #37, 1000.000000000000000 ) ;
#9177=ORIENTED_EDGE ( 'NONE', *, *, #5658, .T. ) ;
#9180=ADVANCED_FACE ( 'NONE', ( #6427 ), #10691, .T. ) ;
#9182=CARTESIAN_POINT ( 'NONE',  ( 10.69346802281034670, 77.87317997377837742, 2.619144277183853949E-15 ) ) ;
#9184=DIRECTION ( 'NONE',  ( -1.000000000000000000, 0.000000000000000000, 0.000000000000000000 ) ) ;
#9185=CARTESIAN_POINT ( 'NONE',  ( -5.680349950370690237, -113.5502101303394795, 1.948972962826602595 ) ) ;
#9186=CARTESIAN_POINT ( 'NONE',  ( 8.385254915620294014, 15.32944684068712782, -16.77050983124058092 ) ) ;
#9187=VERTEX_POINT ( 'NONE', #13033 ) ;
#9189=ORIENTED_EDGE ( 'NONE', *, *, #4368, .T. ) ;
#9190=DIRECTION ( 'NONE',  ( -2.797435172181481150E-17, 1.000000000000000000, -1.765856845898762549E-18 ) ) ;
#9192=VECTOR ( 'NONE', #13075, 1000.000000000000000 ) ;
#9193=DIRECTION ( 'NONE',  ( -2.797435172181481150E-17, 1.000000000000000000, -1.765856845898762549E-18 ) ) ;
#9194=ORIENTED_EDGE ( 'NONE', *, *, #11337, .T. ) ;
#9195=CARTESIAN_POINT ( 'NONE',  ( -8.385254915620295790, -24.99427717735608567, 16.77050983124058448 ) ) ;
#9196=CARTESIAN_POINT ( 'NONE',  ( 10.14576398710721783, -69.00000000000005684, -0.5510781487875693330 ) ) ;
#9197=ORIENTED_EDGE ( 'NONE', *, *, #2691, .F. ) ;
#9199=CARTESIAN_POINT ( 'NONE',  ( 9.567184148105981834, -70.42919439161140360, 3.281027098466867464 ) ) ;
#9202=AXIS2_PLACEMENT_3D ( 'NONE', #4221, #9633, #8575 ) ;
#9205=CARTESIAN_POINT ( 'NONE',  ( -0.7374174230184700196, -122.9090909090941182, -5.357146445002623381 ) ) ;
#9207=VECTOR ( 'NONE', #11629, 1000.000000000000114 ) ;
#9208=DIRECTION ( 'NONE',  ( 0.4545454545454531425, -0.8907235428302472391, 0.000000000000000000 ) ) ;
#9209=( NAMED_UNIT ( * ) SI_UNIT ( $, .STERADIAN. ) SOLID_ANGLE_UNIT ( ) );
#9211=ORIENTED_EDGE ( 'NONE', *, *, #12755, .T. ) ;
#9214=CARTESIAN_POINT ( 'NONE',  ( -2.766560656733045853, -127.7923590214256109, 3.298708284048937678 ) ) ;
#9217=FACE_OUTER_BOUND ( 'NONE', #12234, .T. ) ;
#9220=LINE ( 'NONE', #739, #3928 ) ;
#9222=CARTESIAN_POINT ( 'NONE',  ( -10.00000000000000711, 139.9999999999999716, 0.5000000000000000000 ) ) ;
#9223=CARTESIAN_POINT ( 'NONE',  ( 0.4876856653298393685, -123.8023944157542928, -4.768975623142601705 ) ) ;
#9224=EDGE_CURVE ( 'NONE', #5091, #10788, #2207, .T. ) ;
#9225=DIRECTION ( 'NONE',  ( 0.000000000000000000, 0.000000000000000000, 1.000000000000000000 ) ) ;
#9229=CARTESIAN_POINT ( 'NONE',  ( 50.00000000000000000, 120.0000000000000284, -0.5000000000000000000 ) ) ;
#9231=CARTESIAN_POINT ( 'NONE',  ( -8.385254915620295790, 50.40394642271930792, -8.900615385087330109E-17 ) ) ;
#9234=CARTESIAN_POINT ( 'NONE',  ( 12.99553232110413781, 39.34908859458022334, 0.000000000000000000 ) ) ;
#9236=CARTESIAN_POINT ( 'NONE',  ( -1.315456961488311816, -124.8181818181790845, 4.422452657364224216 ) ) ;
#9237=ORIENTED_EDGE ( 'NONE', *, *, #9173, .F. ) ;
#9238=ORIENTED_EDGE ( 'NONE', *, *, #6935, .T. ) ;
#9239=CARTESIAN_POINT ( 'NONE',  ( -4.769557440008701299, 90.26587002877201371, -1.504714191168455617 ) ) ;
#9242=CARTESIAN_POINT ( 'NONE',  ( 15.29705854078139105, 8.361467971976955127, 3.746698755667522411E-15 ) ) ;
#9244=CARTESIAN_POINT ( 'NONE',  ( -10.69346802281034847, 21.32451227372186864, 21.38693604562068629 ) ) ;
#9248=CARTESIAN_POINT ( 'NONE',  ( -6.048265501886390005, -84.12083291287146380, 7.424871006034148735 ) ) ;
#9251=CARTESIAN_POINT ( 'NONE',  ( -15.29705854078139993, -19.91286587805129926, -3.752661754979895291E-15 ) ) ;
#9253=CARTESIAN_POINT ( 'NONE',  ( -25.00000000000000355, 120.0000000000000284, 2.500000000000000000 ) ) ;
#9254=DIRECTION ( 'NONE',  ( 0.000000000000000000, -1.000000000000000000, 0.000000000000000000 ) ) ;
#9255=CARTESIAN_POINT ( 'NONE',  ( -3.941069743610159826, -121.1799723486271034, -3.201832936236748139 ) ) ;
#9261=CARTESIAN_POINT ( 'NONE',  ( -3.523137085080624953, 90.23509738553477177, -3.551515709300294255 ) ) ;
#9262=CIRCLE ( 'NONE', #7018, 8.385254915620294014 ) ;
#9267=COLOUR_RGB ( '', 0.72549020, 0.75294118, 0.79215686) ;
#9270=CARTESIAN_POINT ( 'NONE',  ( -2.517691654963332357E-15, 90.00000000000000000, -1.589271161308885878E-16 ) ) ;
#9272=B_SPLINE_CURVE_WITH_KNOTS ( 'NONE', 3,
 ( #10264, #541, #10338, #1567 ),
 .UNSPECIFIED., .F., .F.,
 ( 4, 4 ),
 ( 0.000000000000000000, 1.000000000000000000 ),
 .UNSPECIFIED. ) ;
#9275=EDGE_LOOP ( 'NONE', ( #9963, #9639, #12994, #2867 ) ) ;
#9277=CARTESIAN_POINT ( 'NONE',  ( -1.937321831943795631E-15, 69.25350232273815720, -1.222917711790730109E-16 ) ) ;
#9278=EDGE_LOOP ( 'NONE', ( #11872, #11104, #5494, #8971, #515, #2326, #783 ) ) ;
#9279=EDGE_CURVE ( 'NONE', #6913, #7969, #12749, .T. ) ;
#9282=CARTESIAN_POINT ( 'NONE',  ( -0.8176938719062516459, -100.6571748364077479, -7.534607991170741315 ) ) ;
#9284=B_SPLINE_CURVE_WITH_KNOTS ( 'NONE', 3,
 ( #10979, #5728, #993, #2101 ),
 .UNSPECIFIED., .F., .F.,
 ( 4, 4 ),
 ( 0.000000000000000000, 1.000000000000000000 ),
 .UNSPECIFIED. ) ;
#9287=CARTESIAN_POINT ( 'NONE',  ( 0.09563759420350162466, -159.7412891347186417, -1.519396412390668250 ) ) ;
#9289=CARTESIAN_POINT ( 'NONE',  ( 1.830305755871358242, -166.5454546033651866, 12.49768923215308192 ) ) ;
#9291=VECTOR ( 'NONE', #8790, 1000.000000000000000 ) ;
#9293=DIRECTION ( 'NONE',  ( -2.797435172181481150E-17, 1.000000000000000000, -1.765856845898762549E-18 ) ) ;
#9295=AXIS2_PLACEMENT_3D ( 'NONE', #4305, #4233, #10617 ) ;
#9296=CARTESIAN_POINT ( 'NONE',  ( -10.69346802281035202, 30.74929022373127196, 21.38693604562069339 ) ) ;
#9297=EDGE_CURVE ( 'NONE', #8022, #1419, #10283, .T. ) ;
#9301=CARTESIAN_POINT ( 'NONE',  ( 3.722721133221848611, -134.6363636363726073, -2.741844555831716601 ) ) ;
#9303=ORIENTED_EDGE ( 'NONE', *, *, #10941, .F. ) ;
#9306=DIRECTION ( 'NONE',  ( -1.000000000000000000, 0.000000000000000000, 0.000000000000000000 ) ) ;
#9309=DIRECTION ( 'NONE',  ( -1.000000000000000000, 0.000000000000000000, 0.000000000000000000 ) ) ;
#9310=DIRECTION ( 'NONE',  ( 0.000000000000000000, 0.000000000000000000, 1.000000000000000000 ) ) ;
#9314=CIRCLE ( 'NONE', #5267, 24.99999999999998934 ) ;
#9317=EDGE_CURVE ( 'NONE', #297, #10190, #11173, .T. ) ;
#9318=CIRCLE ( 'NONE', #3049, 15.29705854078139460 ) ;
#9319=EDGE_LOOP ( 'NONE', ( #5072, #9488, #5667 ) ) ;
#9320=ORIENTED_EDGE ( 'NONE', *, *, #1232, .T. ) ;
#9321=CARTESIAN_POINT ( 'NONE',  ( -10.69381717166375090, -21.56444287793185310, -21.38763434332751245 ) ) ;
#9322=CIRCLE ( 'NONE', #3265, 14.99999999999999112 ) ;
#9323=CARTESIAN_POINT ( 'NONE',  ( 8.385254915620299343, -34.41905512736551032, 1.085359338644428786E-15 ) ) ;
#9326=DIRECTION ( 'NONE',  ( 0.000000000000000000, 0.000000000000000000, 1.000000000000000000 ) ) ;
#9327=CARTESIAN_POINT ( 'NONE',  ( 2.933105132100035206, -136.4276418140068188, -1.575848925487235430 ) ) ;
#9328=DIRECTION ( 'NONE',  ( -1.000000000000000000, 0.000000000000000000, 0.000000000000000000 ) ) ;
#9329=VECTOR ( 'NONE', #12459, 1000.000000000000000 ) ;
#9331=EDGE_LOOP ( 'NONE', ( #6939, #8786, #6574, #9949 ) ) ;
#9333=DIRECTION ( 'NONE',  ( -1.000000000000000000, 0.000000000000000000, 0.000000000000000000 ) ) ;
#9336=ADVANCED_FACE ( 'NONE', ( #7537 ), #4775, .T. ) ;
#9340=CARTESIAN_POINT ( 'NONE',  ( -11.81226048336476886, -40.00941361824966691, -2.803437019582360665E-15 ) ) ;
#9343=CARTESIAN_POINT ( 'NONE',  ( -5.245880486160382716, -97.41991341987385056, -6.871249260548032645 ) ) ;
#9344=CARTESIAN_POINT ( 'NONE',  ( -1.937321831943795631E-15, 69.25350232273815720, -1.222917711790730109E-16 ) ) ;
#9347=CARTESIAN_POINT ( 'NONE',  ( 1.578201174752436931, -125.2149084904265237, 4.340944873416423988 ) ) ;
#9350=ORIENTED_EDGE ( 'NONE', *, *, #13131, .T. ) ;
#9354=CARTESIAN_POINT ( 'NONE',  ( -10.69346802281035025, 40.17406817374067174, 21.38693604562068629 ) ) ;
#9356=CARTESIAN_POINT ( 'NONE',  ( 25.00000000000000355, 120.0000000000000284, 2.500000000000000000 ) ) ;
#9358=CARTESIAN_POINT ( 'NONE',  ( -1.947123472254133514, -103.3177942292664682, 7.015773985931269330 ) ) ;
#9360=DIRECTION ( 'NONE',  ( -2.797435172181481150E-17, 1.000000000000000000, -1.765856845898762549E-18 ) ) ;
#9361=EDGE_CURVE ( 'NONE', #2743, #7000, #11893, .T. ) ;
#9362=CARTESIAN_POINT ( 'NONE',  ( 10.69346802281034314, 21.32451227372186864, 1.286451862695887858E-15 ) ) ;
#9364=CARTESIAN_POINT ( 'NONE',  ( -12.99553232110414491, 1.649976794542511893, -3.188994717863913482E-15 ) ) ;
#9366=CARTESIAN_POINT ( 'NONE',  ( 12.99553232110413425, 29.92431064457076673, 25.99106464220827917 ) ) ;
#9367=DIRECTION ( 'NONE',  ( -1.000000000000000000, 0.000000000000000000, 0.000000000000000000 ) ) ;
#9368=EDGE_LOOP ( 'NONE', ( #10990, #8408, #11268, #10999 ) ) ;
#9369=CARTESIAN_POINT ( 'NONE',  ( -10.00000000000000000, 97.99999999999994316, 0.5000000000000000000 ) ) ;
#9371=CARTESIAN_POINT ( 'NONE',  ( -2.518175769240240225, -124.8181818181793403, -12.81633841918550587 ) ) ;
#9373=CARTESIAN_POINT ( 'NONE',  ( -8.385254915620294014, -12.94488700934118341, -9.811799245552379678E-16 ) ) ;
#9378=CARTESIAN_POINT ( 'NONE',  ( 9.883290025451533012, -72.00000000000005684, 4.866269441041092492 ) ) ;
#9379=CARTESIAN_POINT ( 'NONE',  ( -6.295302226910096444, -164.3636363587446851, 1.035156591326615194 ) ) ;
#9380=CIRCLE ( 'NONE', #4666, 69.99999999999998579 ) ;
#9381=EDGE_CURVE ( 'NONE', #10921, #1460, #1768, .T. ) ;
#9382=DIRECTION ( 'NONE',  ( 1.000000000000000000, 0.000000000000000000, 0.000000000000000000 ) ) ;
#9383=DIRECTION ( 'NONE',  ( 1.000000000000000000, -0.000000000000000000, 0.000000000000000000 ) ) ;
#9384=CARTESIAN_POINT ( 'NONE',  ( -31.81818181818181657, 133.3608531424536920, 0.5000000000000000000 ) ) ;
#9385=CARTESIAN_POINT ( 'NONE',  ( -4.895553837162441191, 90.06565955263931755, 1.025098571782897539 ) ) ;
#9386=AXIS2_PLACEMENT_3D ( 'NONE', #13116, #10702, #1183 ) ;
#9387=ORIENTED_EDGE ( 'NONE', *, *, #7650, .T. ) ;
#9389=DIRECTION ( 'NONE',  ( -2.797435172181481150E-17, 1.000000000000000000, -1.765856845898762549E-18 ) ) ;
#9390=EDGE_LOOP ( 'NONE', ( #5533, #5530, #11686, #1431 ) ) ;
#9391=CARTESIAN_POINT ( 'NONE',  ( 15.29705854078139282, -10.48808792804187284, 1.919277763901059081E-15 ) ) ;
#9393=ADVANCED_FACE ( 'NONE', ( #5717 ), #9856, .T. ) ;
#9395=DIRECTION ( 'NONE',  ( -1.000000000000000000, 0.000000000000000000, -0.000000000000000000 ) ) ;
#9397=CARTESIAN_POINT ( 'NONE',  ( -38.80000000000001137, 101.5999999999999943, -0.5000000000000000000 ) ) ;
#9398=ORIENTED_EDGE ( 'NONE', *, *, #190, .T. ) ;
#9401=CARTESIAN_POINT ( 'NONE',  ( 12.99553232110413781, -7.774801155466914970, 25.99106464220828627 ) ) ;
#9406=CARTESIAN_POINT ( 'NONE',  ( 11.81226048336477419, -40.00941361824966691, -23.62452096672953061 ) ) ;
#9407=ORIENTED_EDGE ( 'NONE', *, *, #4267, .F. ) ;
#9408=DIRECTION ( 'NONE',  ( -1.000000000000000000, 0.000000000000000000, 0.000000000000000000 ) ) ;
#9409=CARTESIAN_POINT ( 'NONE',  ( -6.635975953222427393, -85.78354978363292105, 7.919939413296249064 ) ) ;
#9414=CARTESIAN_POINT ( 'NONE',  ( 0.005457668171268584105, -157.8901001905733779, -1.500051909670263139 ) ) ;
#9416=ORIENTED_EDGE ( 'NONE', *, *, #9857, .T. ) ;
#9419=AXIS2_PLACEMENT_3D ( 'NONE', #9807, #215, #4468 ) ;
#9421=ORIENTED_EDGE ( 'NONE', *, *, #12107, .T. ) ;
#9423=CARTESIAN_POINT ( 'NONE',  ( -15.29705854078139282, 90.00000000000000000, -1.589271161308885878E-16 ) ) ;
#9426=CARTESIAN_POINT ( 'NONE',  ( 6.961008101167614370, -85.11900100802145630, -6.453057539919575092 ) ) ;
#9427=AXIS2_PLACEMENT_3D ( 'NONE', #11135, #3694, #10290 ) ;
#9429=CARTESIAN_POINT ( 'NONE',  ( 15.29705854078139282, 64.91013567203349055, 1.757061666260241479E-15 ) ) ;
#9433=CARTESIAN_POINT ( 'NONE',  ( 15.29705854078138572, 66.79670324143890525, 1.757061666260240493E-15 ) ) ;
#9434=B_SPLINE_CURVE_WITH_KNOTS ( 'NONE', 3,
 ( #5950, #3972, #11336, #13554, #10356, #5092, #9239, #10285, #10222, #3904, #8183, #7193, #2987, #7259 ),
 .UNSPECIFIED., .F., .F.,
 ( 4, 2, 2, 2, 2, 2, 4 ),
 ( 0.000000000000000000, 0.0003997920717328744657, 0.0007995841434657492567, 0.001199376215198623939, 0.001599168286931498947, 0.002398752430397247878, 0.003198336573862997894 ),
 .UNSPECIFIED. ) ;
#9439=EDGE_LOOP ( 'NONE', ( #8052, #3563, #10284, #9320 ) ) ;
#9440=DIRECTION ( 'NONE',  ( -1.000000000000000000, 0.000000000000000000, 0.000000000000000000 ) ) ;
#9442=CARTESIAN_POINT ( 'NONE',  ( 2.078065350776520770, -164.3636363707227019, -0.8722068067433885741 ) ) ;
#9443=ADVANCED_FACE ( 'NONE', ( #3532 ), #494, .T. ) ;
#9445=DIRECTION ( 'NONE',  ( -1.000000000000000000, 0.000000000000000000, 0.000000000000000000 ) ) ;
#9447=CARTESIAN_POINT ( 'NONE',  ( -8.385254915620292238, -12.94488700934118341, 2.285881734483108495E-17 ) ) ;
#9448=CARTESIAN_POINT ( 'NONE',  ( -2.517691654963332357E-15, 90.00000000000000000, -1.589271161308885878E-16 ) ) ;
#9449=CARTESIAN_POINT ( 'NONE',  ( -0.05222919906010464047, -79.03030303040573301, 10.66847369583533833 ) ) ;
#9451=CARTESIAN_POINT ( 'NONE',  ( -2.318285725477304826, -147.1038961039276103, -4.595794441988434897 ) ) ;
#9455=DIRECTION ( 'NONE',  ( 0.8000000000000024869, 0.5999999999999966471, 0.000000000000000000 ) ) ;
#9456=EDGE_CURVE ( 'NONE', #10190, #3968, #1029, .T. ) ;
#9457=CARTESIAN_POINT ( 'NONE',  ( 8.385254915620294014, 78.67828027274755698, 8.868043070384791430E-16 ) ) ;
#9458=ADVANCED_FACE ( 'NONE', ( #7442 ), #10928, .T. ) ;
#9463=CARTESIAN_POINT ( 'NONE',  ( -10.69346802281035202, 68.44840202376897764, 21.38693604562068984 ) ) ;
#9465=CARTESIAN_POINT ( 'NONE',  ( 10.69381717166375800, -2.714886977913000266, -21.38763434332750890 ) ) ;
#9466=CARTESIAN_POINT ( 'NONE',  ( 0.1375295535854284268, -156.3065963616199952, 1.553835674430288361 ) ) ;
#9472=CIRCLE ( 'NONE', #13072, 8.385254915620294014 ) ;
#9474=CYLINDRICAL_SURFACE ( 'NONE', #8161, 15.29705854078139105 ) ;
#9475=CARTESIAN_POINT ( 'NONE',  ( 9.841115069317121211, -69.87878787878895537, 2.624300023644874802 ) ) ;
#9478=CARTESIAN_POINT ( 'NONE',  ( 1.693173457972444007, -102.5454545454498287, -7.725659299994166673 ) ) ;
#9482=DIRECTION ( 'NONE',  ( 1.000000000000000000, -0.000000000000000000, 0.000000000000000000 ) ) ;
#9483=AXIS2_PLACEMENT_3D ( 'NONE', #7484, #10640, #5312 ) ;
#9484=CARTESIAN_POINT ( 'NONE',  ( 1.588505082198262697, -106.0776627462951893, -6.756253827230843889 ) ) ;
#9487=ORIENTED_EDGE ( 'NONE', *, *, #2849, .T. ) ;
#9488=ORIENTED_EDGE ( 'NONE', *, *, #13453, .T. ) ;
#9491=ORIENTED_EDGE ( 'NONE', *, *, #13419, .F. ) ;
#9493=CARTESIAN_POINT ( 'NONE',  ( -2.656653910027198418, -104.0676472691006893, 6.674219718668044088 ) ) ;
#9496=FACE_OUTER_BOUND ( 'NONE', #83, .T. ) ;
#9498=FACE_OUTER_BOUND ( 'NONE', #1959, .T. ) ;
#9499=CARTESIAN_POINT ( 'NONE',  ( -8.385254915620299343, 31.55439052270045508, 16.77050983124058803 ) ) ;
#9501=CARTESIAN_POINT ( 'NONE',  ( -8.385254915620295790, 50.40394642271930792, -8.900615385087330109E-17 ) ) ;
#9503=CARTESIAN_POINT ( 'NONE',  ( 6.075667645224868352, -100.2727272727253762, 11.56208117637901367 ) ) ;
#9505=CARTESIAN_POINT ( 'NONE',  ( 36.36363636363638108, 142.2680885707561629, -0.5000000000000000000 ) ) ;
#9506=ORIENTED_EDGE ( 'NONE', *, *, #1706, .F. ) ;
#9511=CARTESIAN_POINT ( 'NONE',  ( -4.801896836367436805, -140.5584415584283136, -0.8531065430122782844 ) ) ;
#9512=FACE_OUTER_BOUND ( 'NONE', #12933, .T. ) ;
#9513=CARTESIAN_POINT ( 'NONE',  ( 8.385254915620288685, -22.36966495935058319, 16.77050983124058448 ) ) ;
#9514=CARTESIAN_POINT ( 'NONE',  ( -15.29705854078138749, 17.78624592198638155, -3.140796412417860432E-17 ) ) ;
#9517=( BOUNDED_SURFACE ( )  B_SPLINE_SURFACE ( 3, 3, ( 
 ( #4948, #5790, #8175, #9022 ),
 ( #2710, #553, #10276, #3895 ),
 ( #12393, #12319, #9093, #7892 ),
 ( #13409, #5873, #11327, #678 ) ),
 .UNSPECIFIED., .F., .F., .T. ) 
 B_SPLINE_SURFACE_WITH_KNOTS ( ( 4, 4 ),
 ( 4, 4 ),
 ( 0.000000000000000000, 1.000000000000000000 ),
 ( 0.000000000000000000, 1.000000000000000000 ),
 .UNSPECIFIED. ) 
 GEOMETRIC_REPRESENTATION_ITEM ( )  RATIONAL_B_SPLINE_SURFACE ( (
 ( 1.000000000000000000, 0.3333333333333334259, 0.3333333333333334259, 1.000000000000000000),
 ( 1.000000000000000000, 0.3333333333333334259, 0.3333333333333334259, 1.000000000000000000),
 ( 1.000000000000000000, 0.3333333333333334259, 0.3333333333333334259, 1.000000000000000000),
 ( 1.000000000000000000, 0.3333333333333334259, 0.3333333333333334259, 1.000000000000000000) ) ) 
 REPRESENTATION_ITEM ( '' )  SURFACE ( )  );
#9520=EDGE_LOOP ( 'NONE', ( #6117, #6294, #4645, #13057, #4697, #1828, #1456, #10398, #7099 ) ) ;
#9521=CARTESIAN_POINT ( 'NONE',  ( -10.69381717166375800, -12.13966492792242846, -2.608463437619201972E-15 ) ) ;
#9524=FACE_OUTER_BOUND ( 'NONE', #62, .T. ) ;
#9525=CARTESIAN_POINT ( 'NONE',  ( 15.29705854078139105, 55.48535772202409078, 3.746698755667522411E-15 ) ) ;
#9526=AXIS2_PLACEMENT_3D ( 'NONE', #4151, #2053, #13801 ) ;
#9528=CARTESIAN_POINT ( 'NONE',  ( -9.346811146468073872, -72.85217760321077662, -3.836677974710975825 ) ) ;
#9531=CARTESIAN_POINT ( 'NONE',  ( -0.09322702834623840251, -158.9444566874213649, 1.495102636027880738 ) ) ;
#9533=ORIENTED_EDGE ( 'NONE', *, *, #9456, .F. ) ;
#9536=AXIS2_PLACEMENT_3D ( 'NONE', #12150, #4715, #12294 ) ;
#9539=DIRECTION ( 'NONE',  ( -1.000000000000000000, 0.000000000000000000, 0.000000000000000000 ) ) ;
#9540=EDGE_LOOP ( 'NONE', ( #84, #13297, #12642, #7663 ) ) ;
#9541=CARTESIAN_POINT ( 'NONE',  ( -12.99553232110414136, 77.04820039461787928, -3.342169200734026966E-15 ) ) ;
#9543=CARTESIAN_POINT ( 'NONE',  ( 8.385254915620294014, 12.70483462268159869, 1.002145295323929345E-15 ) ) ;
#9548=FACE_OUTER_BOUND ( 'NONE', #9319, .T. ) ;
#9549=CARTESIAN_POINT ( 'NONE',  ( -10.69346802281034314, 68.44840202376897764, -21.38693604562069339 ) ) ;
#9550=CARTESIAN_POINT ( 'NONE',  ( 5.460914694296556959, -112.4006836749990157, -2.878044288879566537 ) ) ;
#9555=ORIENTED_EDGE ( 'NONE', *, *, #3976, .T. ) ;
#9556=CARTESIAN_POINT ( 'NONE',  ( 1.344026405355564169, -147.1527166344052944, -1.755549728608237103 ) ) ;
#9558=CARTESIAN_POINT ( 'NONE',  ( 10.69346802281033959, 40.17406817374067174, 21.38693604562069339 ) ) ;
#9559=CARTESIAN_POINT ( 'NONE',  ( 8.385254915620295790, 40.97916847270985841, -16.77050983124058803 ) ) ;
#9560=CARTESIAN_POINT ( 'NONE',  ( -4.482662878548983265, -106.3727478091148413, 5.212856551961477791 ) ) ;
#9563=CARTESIAN_POINT ( 'NONE',  ( -5.312266725920361310, -76.81818181818026403, -8.563072071058062562 ) ) ;
#9566=B_SPLINE_CURVE_WITH_KNOTS ( 'NONE', 3,
 ( #1739, #11482, #2994, #10565, #11410, #699, #5101, #2934, #12685, #2011, #967, #10495, #9385, #1876, #6023, #765 ),
 .UNSPECIFIED., .F., .F.,
 ( 4, 2, 2, 2, 2, 2, 2, 4 ),
 ( 0.000000000000000000, 0.0003997740159331186868, 0.0007995480318662373737, 0.001599096063732474747, 0.001998870079665579069, 0.002398644095598683607, 0.002798418111531788145, 0.003198192127464892683 ),
 .UNSPECIFIED. ) ;
#9569=CARTESIAN_POINT ( 'NONE',  ( 12.05891082652324187, -95.36363636363958562, 5.087868926931951918 ) ) ;
#9574=CYLINDRICAL_SURFACE ( 'NONE', #3452, 69.99999999999998579 ) ;
#9576=CARTESIAN_POINT ( 'NONE',  ( 12.85629483954539509, -68.90909090904808920, -2.086541329743980544 ) ) ;
#9577=( BOUNDED_SURFACE ( )  B_SPLINE_SURFACE ( 3, 3, ( 
 ( #4789, #1414, #10251, #3501 ),
 ( #3576, #6816, #13451, #1626 ),
 ( #8843, #10118, #8998, #5910 ),
 ( #7940, #387, #2465, #10044 ) ),
 .UNSPECIFIED., .F., .F., .T. ) 
 B_SPLINE_SURFACE_WITH_KNOTS ( ( 4, 4 ),
 ( 4, 4 ),
 ( 0.000000000000000000, 1.000000000000000000 ),
 ( 0.000000000000000000, 1.000000000000000000 ),
 .UNSPECIFIED. ) 
 GEOMETRIC_REPRESENTATION_ITEM ( )  RATIONAL_B_SPLINE_SURFACE ( (
 ( 1.000000000000000000, 0.3333333333333334259, 0.3333333333333334259, 1.000000000000000000),
 ( 1.000000000000000000, 0.3333333333333334259, 0.3333333333333334259, 1.000000000000000000),
 ( 1.000000000000000000, 0.3333333333333334259, 0.3333333333333334259, 1.000000000000000000),
 ( 1.000000000000000000, 0.3333333333333334259, 0.3333333333333334259, 1.000000000000000000) ) ) 
 REPRESENTATION_ITEM ( '' )  SURFACE ( )  );
#9578=B_SPLINE_CURVE_WITH_KNOTS ( 'NONE', 3,
 ( #13066, #7699, #6654, #7563, #9890, #4624, #1320, #8687, #80, #12925, #1262, #6524, #5527, #291, #4546, #13130 ),
 .UNSPECIFIED., .F., .F.,
 ( 4, 2, 2, 2, 2, 2, 2, 4 ),
 ( 0.000000000000000000, 0.0009977135201011866263, 0.001496570280151776578, 0.001995427040202366747, 0.002494283800252957133, 0.002993140560303546652, 0.003491997320354136604, 0.003990854080404726556 ),
 .UNSPECIFIED. ) ;
#9579=CARTESIAN_POINT ( 'NONE',  ( -2.517691654963332357E-15, 90.00000000000000000, -1.589271161308885878E-16 ) ) ;
#9580=DIRECTION ( 'NONE',  ( 2.797435172181480534E-17, -1.000000000000000000, 1.765856845898762164E-18 ) ) ;
#9581=CYLINDRICAL_SURFACE ( 'NONE', #8571, 40.00000000000001421 ) ;
#9583=EDGE_CURVE ( 'NONE', #3686, #4067, #5271, .T. ) ;
#9587=ORIENTED_EDGE ( 'NONE', *, *, #802, .F. ) ;
#9589=CARTESIAN_POINT ( 'NONE',  ( 8.385254915620286909, 69.25350232273815720, 16.77050983124058803 ) ) ;
#9591=CARTESIAN_POINT ( 'NONE',  ( -7.128864053853600780, -75.84752380246891335, -7.199434380052077920 ) ) ;
#9592=CARTESIAN_POINT ( 'NONE',  ( 1.390017065852572786, -130.6856209220848370, -3.735574746655039746 ) ) ;
#9594=CARTESIAN_POINT ( 'NONE',  ( -12.99553232110414314, 11.07475474455194053, 25.99106464220826851 ) ) ;
#9595=AXIS2_PLACEMENT_3D ( 'NONE', #2751, #2818, #13301 ) ;
#9596=EDGE_LOOP ( 'NONE', ( #7523, #10613, #4538, #3282 ) ) ;
#9598=ADVANCED_FACE ( 'NONE', ( #7309 ), #8608, .T. ) ;
#9602=CARTESIAN_POINT ( 'NONE',  ( -2.517691654963332357E-15, 90.00000000000000000, -1.589271161308885878E-16 ) ) ;
#9603=ORIENTED_EDGE ( 'NONE', *, *, #6097, .F. ) ;
#9605=CARTESIAN_POINT ( 'NONE',  ( -1.868594470333698657E-15, 66.79670324143890525, -1.179534157023628988E-16 ) ) ;
#9606=EDGE_LOOP ( 'NONE', ( #10898, #884, #7012, #5248 ) ) ;
#9607=CYLINDRICAL_SURFACE ( 'NONE', #2721, 5.000000000000000000 ) ;
#9608=CARTESIAN_POINT ( 'NONE',  ( 8.385254915620292238, 40.97916847270985130, 9.522168693316296019E-16 ) ) ;
#9611=CARTESIAN_POINT ( 'NONE',  ( 12.99553232110413958, 67.62342244460847951, -25.99106464220826851 ) ) ;
#9612=CARTESIAN_POINT ( 'NONE',  ( 2.008006476061143353, -80.00378950643523979, 9.910921260988354575 ) ) ;
#9617=ORIENTED_EDGE ( 'NONE', *, *, #6433, .T. ) ;
#9619=EDGE_CURVE ( 'NONE', #2743, #8621, #5129, .T. ) ;
#9621=DIRECTION ( 'NONE',  ( -1.000000000000000000, 0.000000000000000000, 0.000000000000000000 ) ) ;
#9622=ORIENTED_EDGE ( 'NONE', *, *, #6438, .F. ) ;
#9624=CARTESIAN_POINT ( 'NONE',  ( 8.406708282432173718, -87.41492670881856952, -3.778913651227076453 ) ) ;
#9626=AXIS2_PLACEMENT_3D ( 'NONE', #10141, #1779, #2708 ) ;
#9627=CARTESIAN_POINT ( 'NONE',  ( -1.995220113908458437, -142.5800865802677322, -1.459423439931805788 ) ) ;
#9628=CARTESIAN_POINT ( 'NONE',  ( -10.69381717166375623, 63.25855867215299355, -2.761346882366286462E-15 ) ) ;
#9631=CARTESIAN_POINT ( 'NONE',  ( -2.563982627555806637, -78.09090909090801347, -9.749794964675981390 ) ) ;
#9633=DIRECTION ( 'NONE',  ( -2.797435172181481150E-17, 1.000000000000000000, -1.765856845898762549E-18 ) ) ;
#9639=ORIENTED_EDGE ( 'NONE', *, *, #8736, .T. ) ;
#9641=CARTESIAN_POINT ( 'NONE',  ( -8.385254915620295790, 69.25350232273815720, -1.222917711790730109E-16 ) ) ;
#9645=CARTESIAN_POINT ( 'NONE',  ( 12.99553232110414491, 1.649976794542512559, 3.182987412051232562E-15 ) ) ;
#9646=CARTESIAN_POINT ( 'NONE',  ( -1.133743435584524839, -129.7272727272675752, 4.472427317383624867 ) ) ;
#9647=AXIS2_PLACEMENT_3D ( 'NONE', #3753, #7965, #12248 ) ;
#9649=FACE_OUTER_BOUND ( 'NONE', #722, .T. ) ;
#9652=DIRECTION ( 'NONE',  ( -2.797435172181481150E-17, 1.000000000000000000, -1.765856845898762549E-18 ) ) ;
#9653=TOROIDAL_SURFACE ( 'NONE', #3838, 22.99999999999999289, 2.000000000000000000 ) ;
#9655=AXIS2_PLACEMENT_3D ( 'NONE', #10139, #612, #11324 ) ;
#9660=CARTESIAN_POINT ( 'NONE',  ( 15.29705854078137861, 66.79670324143890525, 30.59411708156277498 ) ) ;
#9661=CARTESIAN_POINT ( 'NONE',  ( 12.99579180576516713, 54.65873172698324112, 3.183050967463142985E-15 ) ) ;
#9663=CARTESIAN_POINT ( 'NONE',  ( 15.29705854078139815, 0.8232575913728894523, 1.873561326908940224E-15 ) ) ;
#9665=ORIENTED_EDGE ( 'NONE', *, *, #1386, .T. ) ;
#9668=ORIENTED_EDGE ( 'NONE', *, *, #5433, .F. ) ;
#9671=EDGE_CURVE ( 'NONE', #9709, #11311, #12075, .T. ) ;
#9672=CARTESIAN_POINT ( 'NONE',  ( -8.385254915620294014, 90.00000000000000000, -1.589271161308885878E-16 ) ) ;
#9677=CARTESIAN_POINT ( 'NONE',  ( -7.874681298106575689, -95.09370015314794955, -2.462075568715513363 ) ) ;
#9679=CARTESIAN_POINT ( 'NONE',  ( 2.933974605883639275E-16, -10.48808792804187284, 1.852046186812095429E-17 ) ) ;
#9682=EDGE_LOOP ( 'NONE', ( #367, #7905, #9303, #5000 ) ) ;
#9683=CARTESIAN_POINT ( 'NONE',  ( -4.130090007162179333, 90.90347248489018739, 2.819710018450384048 ) ) ;
#9689=AXIS2_PLACEMENT_3D ( 'NONE', #6439, #4455, #2428 ) ;
#9694=CARTESIAN_POINT ( 'NONE',  ( 0.1768551147990858330, -79.21212121212114710, -10.18346664538823454 ) ) ;
#9695=CARTESIAN_POINT ( 'NONE',  ( -33.99999999999999289, 108.0000000000000142, -0.5000000000000000000 ) ) ;
#9698=AXIS2_PLACEMENT_3D ( 'NONE', #12968, #3336, #7613 ) ;
#9699=EDGE_CURVE ( 'NONE', #10906, #13516, #7644, .T. ) ;
#9700=ORIENTED_EDGE ( 'NONE', *, *, #2924, .T. ) ;
#9701=DIRECTION ( 'NONE',  ( -1.000000000000000000, -2.835060530349834805E-17, 0.000000000000000000 ) ) ;
#9706=DIRECTION ( 'NONE',  ( -1.000000000000000000, 0.000000000000000000, 0.000000000000000000 ) ) ;
#9708=FACE_OUTER_BOUND ( 'NONE', #3022, .T. ) ;
#9709=VERTEX_POINT ( 'NONE', #6534 ) ;
#9711=CARTESIAN_POINT ( 'NONE',  ( 15.29705854078138394, 27.21102387199583461, 30.59411708156277854 ) ) ;
#9715=DIRECTION ( 'NONE',  ( -1.000000000000000000, 0.000000000000000000, 0.000000000000000000 ) ) ;
#9720=DIRECTION ( 'NONE',  ( -1.000000000000000000, 0.000000000000000000, 0.000000000000000000 ) ) ;
#9722=EDGE_CURVE ( 'NONE', #11519, #13719, #2861, .T. ) ;
#9723=AXIS2_PLACEMENT_3D ( 'NONE', #1692, #10583, #8348 ) ;
#9726=DIRECTION ( 'NONE',  ( 0.000000000000000000, 0.000000000000000000, 1.000000000000000000 ) ) ;
#9727=AXIS2_PLACEMENT_3D ( 'NONE', #8965, #7906, #11896 ) ;
#9728=CARTESIAN_POINT ( 'NONE',  ( -15.29705854078138927, -38.76242177807012723, 6.844888786042043893E-17 ) ) ;
#9734=EDGE_LOOP ( 'NONE', ( #7166, #11398, #6485, #13107 ) ) ;
#9735=B_SPLINE_CURVE_WITH_KNOTS ( 'NONE', 3,
 ( #7535, #6561, #4311, #11039 ),
 .UNSPECIFIED., .F., .F.,
 ( 4, 4 ),
 ( 0.000000000000000000, 1.000000000000000000 ),
 .UNSPECIFIED. ) ;
#9738=ORIENTED_EDGE ( 'NONE', *, *, #2150, .T. ) ;
#9743=CARTESIAN_POINT ( 'NONE',  ( -9.175745902881725407E-17, 3.280056672672198914, -5.792110530374064999E-18 ) ) ;
#9746=CARTESIAN_POINT ( 'NONE',  ( -4.898028703968604347, -99.35382711894193619, -6.023273615114322688 ) ) ;
#9747=CYLINDRICAL_SURFACE ( 'NONE', #1027, 2.000000000000000000 ) ;
#9751=EDGE_LOOP ( 'NONE', ( #11467, #11080, #8277, #11833 ) ) ;
#9756=ORIENTED_EDGE ( 'NONE', *, *, #8331, .F. ) ;
#9764=CARTESIAN_POINT ( 'NONE',  ( -7.668969345093498369, -75.54545454545399252, -6.730503492161166612 ) ) ;
#9765=CARTESIAN_POINT ( 'NONE',  ( 8.385254915620295790, -15.56949922734665570, 2.053795118489800793E-15 ) ) ;
#9768=ADVANCED_FACE ( 'NONE', ( #228 ), #1143, .T. ) ;
#9769=CARTESIAN_POINT ( 'NONE',  ( 25.00000000000000355, 120.0000000000000284, -2.500000000000000000 ) ) ;
#9771=ORIENTED_EDGE ( 'NONE', *, *, #12755, .F. ) ;
#9773=B_SPLINE_CURVE_WITH_KNOTS ( 'NONE', 3,
 ( #308, #5410, #6469, #2258 ),
 .UNSPECIFIED., .F., .F.,
 ( 4, 4 ),
 ( 0.000000000000000000, 0.002999984647841453037 ),
 .UNSPECIFIED. ) ;
#9777=VERTEX_POINT ( 'NONE', #13143 ) ;
#9782=FACE_OUTER_BOUND ( 'NONE', #4326, .T. ) ;
#9783=TOROIDAL_SURFACE ( 'NONE', #6421, 16.99999999999998934, 2.000000000000000000 ) ;
#9784=CARTESIAN_POINT ( 'NONE',  ( 1.031578115675553693E-15, -36.87585420866476227, 6.511747960273540061E-17 ) ) ;
#9785=B_SPLINE_SURFACE_WITH_KNOTS ( 'NONE', 3, 3, ( 
 ( #1620, #3792, #8009, #11298, #8079, #12424, #12362, #10179, #5905, #651, #11364, #7019, #13296, #9196 ),
 ( #522, #721, #588, #2746, #2815, #2532, #1693, #4854, #7857, #7088, #10112, #1757, #4986, #13222 ),
 ( #3569, #12143, #6809, #4783, #444, #11085, #11161, #13375, #1477, #5758, #10036, #7936, #12219, #2608 ),
 ( #6882, #3725, #12285, #9128, #7293, #13848, #6380, #8281, #784, #6313, #5057, #9475, #13650, #10649 ) ),
 .UNSPECIFIED., .F., .F., .F.,
 ( 4, 4 ),
 ( 4, 1, 1, 1, 1, 1, 1, 1, 1, 1, 1, 4 ),
 ( -0.0003000000000000000279, 0.003299999999999999982 ),
 ( 0.07900000000000007017, 0.08000000000000005718, 0.08063636363636368654, 0.08172727272727277337, 0.08336363636363640361, 0.08445454545454547657, 0.08554545454545456340, 0.08663636363636365023, 0.08827272727272726660, 0.08936363636363635343, 0.08999999999999998279, 0.09099999999999996980 ),
 .UNSPECIFIED. ) ;
#9786=CARTESIAN_POINT ( 'NONE',  ( 12.99579180576516535, 35.80917582696438473, 0.000000000000000000 ) ) ;
#9787=CARTESIAN_POINT ( 'NONE',  ( 15.29705854078139282, 27.21102387199583461, -30.59411708156277498 ) ) ;
#9789=DIRECTION ( 'NONE',  ( -2.797435172181481150E-17, 1.000000000000000000, -1.765856845898762549E-18 ) ) ;
#9791=DIRECTION ( 'NONE',  ( -1.000000000000000000, 0.000000000000000000, 0.000000000000000000 ) ) ;
#9792=AXIS2_PLACEMENT_3D ( 'NONE', #8036, #5642, #6767 ) ;
#9797=VERTEX_POINT ( 'NONE', #1546 ) ;
#9799=DIRECTION ( 'NONE',  ( -0.000000000000000000, -0.000000000000000000, -1.000000000000000000 ) ) ;
#9804=EDGE_CURVE ( 'NONE', #4522, #8317, #8276, .T. ) ;
#9807=CARTESIAN_POINT ( 'NONE',  ( 8.894289287455980914E-16, -31.79444290936001138, 5.614443467303076398E-17 ) ) ;
#9809=CARTESIAN_POINT ( 'NONE',  ( 15.29705854078139282, 74.33491362204294717, 3.746698755667523989E-15 ) ) ;
#9812=CARTESIAN_POINT ( 'NONE',  ( -5.215656969546267341, -75.40994152784138294, -8.686150200711136193 ) ) ;
#9813=CIRCLE ( 'NONE', #11819, 15.29705854078138927 ) ;
#9815=CARTESIAN_POINT ( 'NONE',  ( -10.00000000000000711, 97.99999999999994316, 2.500000000000000000 ) ) ;
#9816=CARTESIAN_POINT ( 'NONE',  ( 15.29705854078140526, -29.33764382806072746, -30.59411708156279630 ) ) ;
#9818=EDGE_LOOP ( 'NONE', ( #5978, #1089, #4362, #4280 ) ) ;
#9819=ORIENTED_EDGE ( 'NONE', *, *, #10268, .F. ) ;
#9821=CIRCLE ( 'NONE', #13217, 15.29705854078139105 ) ;
#9825=CARTESIAN_POINT ( 'NONE',  ( 12.99579180576516002, 35.80917582696438473, 25.99158361153033070 ) ) ;
#9827=DIRECTION ( 'NONE',  ( 0.000000000000000000, 0.000000000000000000, 1.000000000000000000 ) ) ;
#9828=LINE ( 'NONE', #4564, #1583 ) ;
#9829=CARTESIAN_POINT ( 'NONE',  ( -4.858750903447957903, -78.09090909090917876, -8.996753037508826267 ) ) ;
#9831=VECTOR ( 'NONE', #6461, 1000.000000000000000 ) ;
#9832=CARTESIAN_POINT ( 'NONE',  ( 12.99553232110414669, -17.19957910547634228, 3.182987412051232956E-15 ) ) ;
#9833=FILL_AREA_STYLE_COLOUR ( '', #9267 ) ;
#9837=CARTESIAN_POINT ( 'NONE',  ( 8.385254915620288685, 71.87811454074363837, 9.540301975042856912E-16 ) ) ;
#9840=DIRECTION ( 'NONE',  ( 0.000000000000000000, 0.000000000000000000, 1.000000000000000000 ) ) ;
#9841=CIRCLE ( 'NONE', #12767, 69.99999999999998579 ) ;
#9843=ORIENTED_EDGE ( 'NONE', *, *, #271, .F. ) ;
#9845=CARTESIAN_POINT ( 'NONE',  ( -8.385254915620292238, -31.79444290936001138, 5.614443467303076398E-17 ) ) ;
#9846=CIRCLE ( 'NONE', #3803, 5.000000000000000000 ) ;
#9847=CARTESIAN_POINT ( 'NONE',  ( -10.69346802281034847, 2.474956373702985157, -1.318312975903535027E-15 ) ) ;
#9851=CARTESIAN_POINT ( 'NONE',  ( -10.69346802281034492, 11.89973432371241380, -2.649684675786613482E-15 ) ) ;
#9853=CARTESIAN_POINT ( 'NONE',  ( -10.69381717166376333, -30.98922082794128485, 21.38763434332751601 ) ) ;
#9856=CYLINDRICAL_SURFACE ( 'NONE', #6042, 8.385254915620292238 ) ;
#9857=EDGE_CURVE ( 'NONE', #2825, #11519, #8008, .T. ) ;
#9859=EDGE_LOOP ( 'NONE', ( #2638, #8817, #5702, #3553, #4384, #3344, #2292 ) ) ;
#9860=CARTESIAN_POINT ( 'NONE',  ( 10.00000000000000711, 139.9999999999999716, 2.500000000000000000 ) ) ;
#9864=FACE_OUTER_BOUND ( 'NONE', #8751, .T. ) ;
#9866=PRODUCT_CONTEXT ( 'NONE', #10065, 'mechanical' ) ;
#9867=ORIENTED_EDGE ( 'NONE', *, *, #7211, .F. ) ;
#9868=DIRECTION ( 'NONE',  ( 1.000000000000000000, 0.000000000000000000, 0.000000000000000000 ) ) ;
#9870=CIRCLE ( 'NONE', #8740, 8.385254915620294014 ) ;
#9872=ADVANCED_FACE ( 'NONE', ( #6808 ), #845, .T. ) ;
#9874=CARTESIAN_POINT ( 'NONE',  ( 8.385254915620294014, 12.70483462268159869, 2.053795118489800793E-15 ) ) ;
#9876=ORIENTED_EDGE ( 'NONE', *, *, #11489, .T. ) ;
#9878=AXIS2_PLACEMENT_3D ( 'NONE', #3047, #8442, #947 ) ;
#9881=AXIS2_PLACEMENT_3D ( 'NONE', #902, #4055, #8336 ) ;
#9883=VERTEX_POINT ( 'NONE', #10178 ) ;
#9884=DIRECTION ( 'NONE',  ( 2.797435172181480534E-17, -1.000000000000000000, 1.765856845898762164E-18 ) ) ;
#9886=EDGE_CURVE ( 'NONE', #11768, #10108, #4853, .T. ) ;
#9888=VECTOR ( 'NONE', #2775, 1000.000000000000000 ) ;
#9889=CARTESIAN_POINT ( 'NONE',  ( -8.385254915620294014, -15.56949922734665570, 2.749350679782564022E-17 ) ) ;
#9890=CARTESIAN_POINT ( 'NONE',  ( 3.286535165834786554, 90.13351245737435136, -3.771524672989932547 ) ) ;
#9893=VERTEX_POINT ( 'NONE', #4914 ) ;
#9894=EDGE_CURVE ( 'NONE', #6329, #10788, #2099, .T. ) ;
#9901=CARTESIAN_POINT ( 'NONE',  ( -8.385254915620292238, -3.520109059331755663, -1.014465541883437468E-15 ) ) ;
#9905=LINE ( 'NONE', #7653, #9176 ) ;
#9908=DIRECTION ( 'NONE',  ( -1.000000000000000000, 0.000000000000000000, 0.000000000000000000 ) ) ;
#9909=EDGE_LOOP ( 'NONE', ( #12138, #8556, #6013, #7884 ) ) ;
#9910=ORIENTED_EDGE ( 'NONE', *, *, #6470, .F. ) ;
#9913=CIRCLE ( 'NONE', #8356, 8.385254915620295790 ) ;
#9914=DIRECTION ( 'NONE',  ( -0.000000000000000000, -0.000000000000000000, -1.000000000000000000 ) ) ;
#9919=ORIENTED_EDGE ( 'NONE', *, *, #27, .T. ) ;
#9921=CYLINDRICAL_SURFACE ( 'NONE', #675, 15.29705854078139105 ) ;
#9925=CARTESIAN_POINT ( 'NONE',  ( 8.385254915620292238, -31.79444290936001494, 16.77050983124058803 ) ) ;
#9926=CARTESIAN_POINT ( 'NONE',  ( -1.747091603990086329E-15, 62.45333659073423860, -1.102836519679677113E-16 ) ) ;
#9930=DIRECTION ( 'NONE',  ( -2.797435172181481150E-17, 1.000000000000000000, -1.765856845898762549E-18 ) ) ;
#9933=CIRCLE ( 'NONE', #2990, 5.000000000000000000 ) ;
#9936=FACE_OUTER_BOUND ( 'NONE', #9081, .T. ) ;
#9937=ORIENTED_EDGE ( 'NONE', *, *, #2420, .F. ) ;
#9942=CARTESIAN_POINT ( 'NONE',  ( 5.049283658538309183, -77.73593556436266283, 8.777051982195970936 ) ) ;
#9945=ORIENTED_EDGE ( 'NONE', *, *, #7461, .T. ) ;
#9947=B_SPLINE_CURVE_WITH_KNOTS ( 'NONE', 3,
 ( #3654, #2614, #3798, #8085 ),
 .UNSPECIFIED., .F., .F.,
 ( 4, 4 ),
 ( 0.000000000000000000, 1.000000000000000000 ),
 .UNSPECIFIED. ) ;
#9949=ORIENTED_EDGE ( 'NONE', *, *, #207, .F. ) ;
#9950=CARTESIAN_POINT ( 'NONE',  ( 32.72727272727274084, 135.1423002281142089, -2.500000000000000000 ) ) ;
#9951=EDGE_CURVE ( 'NONE', #13265, #1727, #3413, .T. ) ;
#9952=CARTESIAN_POINT ( 'NONE',  ( -10.69346802281034670, -35.22415542633469698, -2.569297226391742986E-15 ) ) ;
#9954=EDGE_CURVE ( 'NONE', #2529, #13355, #264, .T. ) ;
#9958=CARTESIAN_POINT ( 'NONE',  ( -2.517691654963332357E-15, 90.00000000000000000, -1.589271161308885878E-16 ) ) ;
#9959=CARTESIAN_POINT ( 'NONE',  ( 10.69346802281034314, 59.02362407375952102, 2.619144277183853160E-15 ) ) ;
#9960=ORIENTED_EDGE ( 'NONE', *, *, #8397, .F. ) ;
#9963=ORIENTED_EDGE ( 'NONE', *, *, #1457, .F. ) ;
#9964=AXIS2_PLACEMENT_3D ( 'NONE', #7795, #1426, #401 ) ;
#9965=TOROIDAL_SURFACE ( 'NONE', #13595, 48.00000000000001421, 2.000000000000000000 ) ;
#9966=CARTESIAN_POINT ( 'NONE',  ( -10.00000000000000000, 92.00000000000000000, -0.5000000000000000000 ) ) ;
#9968=( BOUNDED_SURFACE ( )  B_SPLINE_SURFACE ( 3, 3, ( 
 ( #11058, #7910, #13277, #7063 ),
 ( #3698, #9244, #12262, #11343 ),
 ( #6860, #4891, #1738, #13424 ),
 ( #13559, #5807, #10013, #501 ) ),
 .UNSPECIFIED., .F., .F., .F. ) 
 B_SPLINE_SURFACE_WITH_KNOTS ( ( 4, 4 ),
 ( 4, 4 ),
 ( 0.000000000000000000, 1.000000000000000000 ),
 ( 0.000000000000000000, 1.000000000000000000 ),
 .UNSPECIFIED. ) 
 GEOMETRIC_REPRESENTATION_ITEM ( )  RATIONAL_B_SPLINE_SURFACE ( (
 ( 1.000000000000000000, 0.3333333333333334259, 0.3333333333333334259, 1.000000000000000000),
 ( 1.000000000000000000, 0.3333333333333334259, 0.3333333333333334259, 1.000000000000000000),
 ( 1.000000000000000000, 0.3333333333333334259, 0.3333333333333334259, 1.000000000000000000),
 ( 1.000000000000000000, 0.3333333333333334259, 0.3333333333333334259, 1.000000000000000000) ) ) 
 REPRESENTATION_ITEM ( '' )  SURFACE ( )  );
#9974=CARTESIAN_POINT ( 'NONE',  ( 5.494716852924988792, -106.9090909090932087, -4.862358660864441795 ) ) ;
#9976=CARTESIAN_POINT ( 'NONE',  ( 2.179449471770333435, 90.00000000000000000, 4.500000000000000888 ) ) ;
#9978=CARTESIAN_POINT ( 'NONE',  ( 6.213657885906443745, -97.41991341991004560, 5.968417174470181941 ) ) ;
#9980=CARTESIAN_POINT ( 'NONE',  ( 15.29705854078139637, -18.02629830864593785, 3.746698755667523989E-15 ) ) ;
#9982=PRESENTATION_STYLE_ASSIGNMENT (( #10256 ) ) ;
#9991=DIRECTION ( 'NONE',  ( -1.000000000000000000, 0.000000000000000000, 0.000000000000000000 ) ) ;
#9995=DIRECTION ( 'NONE',  ( -2.797435172181481150E-17, 1.000000000000000000, -1.765856845898762549E-18 ) ) ;
#9997=DIRECTION ( 'NONE',  ( -2.797435172181481150E-17, 1.000000000000000000, -1.765856845898762549E-18 ) ) ;
#10005=CARTESIAN_POINT ( 'NONE',  ( 10.69346802281034847, -6.949821576306441706, 1.321354522272860754E-15 ) ) ;
#10006=ORIENTED_EDGE ( 'NONE', *, *, #950, .F. ) ;
#10007=VECTOR ( 'NONE', #9383, 1000.000000000000000 ) ;
#10008=ORIENTED_EDGE ( 'NONE', *, *, #636, .F. ) ;
#10013=CARTESIAN_POINT ( 'NONE',  ( 15.29705854078138394, 19.67281349139177138, 30.59411708156277854 ) ) ;
#10015=DIRECTION ( 'NONE',  ( -2.797435172181481150E-17, 1.000000000000000000, -1.765856845898762549E-18 ) ) ;
#10016=PRODUCT ( 'Threaded Steel Worm Screw Spindle', 'Threaded Steel Worm Screw Spindle', '', ( #9866 ) ) ;
#10018=CARTESIAN_POINT ( 'NONE',  ( 10.69346802281034847, -25.79937747632526879, 1.362902637283517672E-15 ) ) ;
#10019=VECTOR ( 'NONE', #9482, 1000.000000000000000 ) ;
#10026=CARTESIAN_POINT ( 'NONE',  ( 3.930324603630738878, -100.3934781419522011, 6.514713691489384395 ) ) ;
#10028=CARTESIAN_POINT ( 'NONE',  ( 15.29705854078138749, 17.78624592198638155, 1.840275709580739737E-15 ) ) ;
#10029=ADVANCED_FACE ( 'NONE', ( #5113 ), #13720, .F. ) ;
#10030=ORIENTED_EDGE ( 'NONE', *, *, #3431, .F. ) ;
#10031=EDGE_LOOP ( 'NONE', ( #10907, #11027, #4979, #12990 ) ) ;
#10032=ADVANCED_FACE ( 'NONE', ( #6244 ), #9474, .T. ) ;
#10033=ADVANCED_FACE ( 'NONE', ( #9864 ), #7749, .T. ) ;
#10036=CARTESIAN_POINT ( 'NONE',  ( 9.601587402597818510, -70.78787878788214982, 2.975959431766512342 ) ) ;
#10038=CARTESIAN_POINT ( 'NONE',  ( 4.363680981163678751, 91.46147893603955481, 2.443653808501017544 ) ) ;
#10042=CARTESIAN_POINT ( 'NONE',  ( 15.29705854078139637, 90.00000000000000000, 1.714422261702873555E-15 ) ) ;
#10044=CARTESIAN_POINT ( 'NONE',  ( -15.29705854078139460, -18.02629830864593785, -3.728963417185749694E-15 ) ) ;
#10045=CARTESIAN_POINT ( 'NONE',  ( 3.692320488640516096, -128.7272727272744248, -2.755591346289505417 ) ) ;
#10047=EDGE_CURVE ( 'NONE', #11768, #11046, #990, .T. ) ;
#10054=EDGE_CURVE ( 'NONE', #9032, #1176, #4407, .T. ) ;
#10057=CARTESIAN_POINT ( 'NONE',  ( 1.528183159915511125, -102.9021681410130356, -7.139114381135374998 ) ) ;
#10059=DIRECTION ( 'NONE',  ( 0.4545454545454531425, 0.8907235428302472391, 0.000000000000000000 ) ) ;
#10060=CARTESIAN_POINT ( 'NONE',  ( -0.1215172727492840610, -143.6254824914774701, 2.565777989091288180 ) ) ;
#10062=DIRECTION ( 'NONE',  ( -2.797435172181481150E-17, 1.000000000000000000, -1.765856845898762549E-18 ) ) ;
#10065=APPLICATION_CONTEXT ( 'automotive_design' ) ;
#10067=DIRECTION ( 'NONE',  ( 2.797435172181480534E-17, -1.000000000000000000, 1.765856845898762164E-18 ) ) ;
#10069=DIRECTION ( 'NONE',  ( -2.797435172181481150E-17, 1.000000000000000000, -1.765856845898762549E-18 ) ) ;
#10075=ORIENTED_EDGE ( 'NONE', *, *, #13592, .F. ) ;
#10076=CARTESIAN_POINT ( 'NONE',  ( -3.056920711451915018, -140.5584415584246187, -3.800163123440760238 ) ) ;
#10077=CIRCLE ( 'NONE', #1559, 2.000000000000000000 ) ;
#10082=CARTESIAN_POINT ( 'NONE',  ( -56.97938482099326762, -167.3636363668308888, -8.923382220094675077 ) ) ;
#10088=CIRCLE ( 'NONE', #8505, 15.29705854078138927 ) ;
#10089=CARTESIAN_POINT ( 'NONE',  ( -15.29705854078138927, -38.76242177807012723, 6.844888786042043893E-17 ) ) ;
#10091=B_SPLINE_CURVE_WITH_KNOTS ( 'NONE', 3,
 ( #3048, #5283, #4023, #8310 ),
 .UNSPECIFIED., .F., .F.,
 ( 4, 4 ),
 ( 0.000000000000000000, 1.000000000000000000 ),
 .UNSPECIFIED. ) ;
#10097=CARTESIAN_POINT ( 'NONE',  ( 10.69346802281035202, -35.22415542633469698, -21.38693604562068984 ) ) ;
#10098=DIRECTION ( 'NONE',  ( -1.000000000000000000, 0.000000000000000000, 0.000000000000000000 ) ) ;
#10099=CARTESIAN_POINT ( 'NONE',  ( -12.99579180576516713, 35.80917582696438473, -1.717993240291646161E-15 ) ) ;
#10101=CARTESIAN_POINT ( 'NONE',  ( 5.563246471219282618, -98.57715322402732738, 5.512450067888273075 ) ) ;
#10103=CARTESIAN_POINT ( 'NONE',  ( 8.385254915620286909, 59.82872437272870769, 16.77050983124058448 ) ) ;
#10105=AXIS2_PLACEMENT_3D ( 'NONE', #217, #11976, #12 ) ;
#10106=CIRCLE ( 'NONE', #4053, 8.385254915620290461 ) ;
#10107=ORIENTED_EDGE ( 'NONE', *, *, #2935, .F. ) ;
#10108=VERTEX_POINT ( 'NONE', #5801 ) ;
#10110=EDGE_CURVE ( 'NONE', #4633, #11396, #267, .T. ) ;
#10112=CARTESIAN_POINT ( 'NONE',  ( 9.888538082662813977, -70.78787878787576915, 1.806551902650904484 ) ) ;
#10114=CARTESIAN_POINT ( 'NONE',  ( 5.938565219940902473, -74.76276777339397484, 8.199189651718064908 ) ) ;
#10118=CARTESIAN_POINT ( 'NONE',  ( 12.99553232110415024, -17.19957910547634228, -25.99106464220828627 ) ) ;
#10119=CARTESIAN_POINT ( 'NONE',  ( -3.341303593452078058, -106.9090909090913755, 6.231874970755803211 ) ) ;
#10120=CYLINDRICAL_SURFACE ( 'NONE', #13600, 15.29705854078139105 ) ;
#10123=ORIENTED_EDGE ( 'NONE', *, *, #816, .T. ) ;
#10128=CARTESIAN_POINT ( 'NONE',  ( 6.160012261085373808, -112.2768544234564416, -0.06296530155695967412 ) ) ;
#10132=ORIENTED_EDGE ( 'NONE', *, *, #3242, .F. ) ;
#10133=ORIENTED_EDGE ( 'NONE', *, *, #43, .T. ) ;
#10136=EDGE_CURVE ( 'NONE', #1146, #8762, #1675, .T. ) ;
#10137=CARTESIAN_POINT ( 'NONE',  ( 2.898805451609365758, -136.7680419189706811, 1.590792564838447998 ) ) ;
#10138=CARTESIAN_POINT ( 'NONE',  ( 4.769534092270758308, 90.26591089801031842, -1.504791211541889329 ) ) ;
#10139=CARTESIAN_POINT ( 'NONE',  ( -2.517691654963332357E-15, 90.00000000000000000, -1.589271161308885878E-16 ) ) ;
#10141=CARTESIAN_POINT ( 'NONE',  ( 9.847276892489302169E-17, -3.520109059331727686, 6.216008680731233110E-18 ) ) ;
#10146=LINE ( 'NONE', #12174, #9329 ) ;
#10147=CARTESIAN_POINT ( 'NONE',  ( 15.29705854078139282, -8.601520358636511432, 1.890204135573039875E-15 ) ) ;
#10148=DIRECTION ( 'NONE',  ( 5.551115123125776539E-17, -1.000000000000000000, -3.944304526105059027E-31 ) ) ;
#10150=CARTESIAN_POINT ( 'NONE',  ( -12.93801431150469128, -134.6363636363606986, 1.977757875721223968 ) ) ;
#10151=AXIS2_PLACEMENT_3D ( 'NONE', #6562, #9652, #3194 ) ;
#10152=ADVANCED_FACE ( 'NONE', ( #4675 ), #6378, .T. ) ;
#10153=EDGE_LOOP ( 'NONE', ( #5700, #12395, #5547, #5780 ) ) ;
#10155=LINE ( 'NONE', #11400, #10189 ) ;
#10156=CARTESIAN_POINT ( 'NONE',  ( 10.69381717166375445, 34.98422482212468054, 1.263224666758019907E-15 ) ) ;
#10157=ADVANCED_FACE ( 'NONE', ( #9936 ), #11731, .T. ) ;
#10161=CARTESIAN_POINT ( 'NONE',  ( -12.97449437267217576, -39.59556244224027211, -1.449077110393148750E-15 ) ) ;
#10164=ORIENTED_EDGE ( 'NONE', *, *, #6097, .T. ) ;
#10165=CARTESIAN_POINT ( 'NONE',  ( 8.385254915620294014, 31.55439052270045508, 9.688596779957294507E-16 ) ) ;
#10172=CARTESIAN_POINT ( 'NONE',  ( 1.383078971141448177, -102.9954216821132746, 7.191944656388454149 ) ) ;
#10173=CARTESIAN_POINT ( 'NONE',  ( -8.385254915620297567, 50.40394642271930792, -2.186308893455868305E-15 ) ) ;
#10177=VERTEX_POINT ( 'NONE', #2422 ) ;
#10178=CARTESIAN_POINT ( 'NONE',  ( -9.736331930512843513, -69.99978782402621391, -2.722951059031194276 ) ) ;
#10179=CARTESIAN_POINT ( 'NONE',  ( 8.599520226296911929, -74.45454545454452955, 5.474475378420848415 ) ) ;
#10180=ORIENTED_EDGE ( 'NONE', *, *, #2211, .T. ) ;
#10181=CARTESIAN_POINT ( 'NONE',  ( 4.942677383991346041, 90.01345119373434045, 0.7661926690451046351 ) ) ;
#10184=CARTESIAN_POINT ( 'NONE',  ( -5.390560935658909258, -117.0909090909071750, -3.329211565280856266 ) ) ;
#10186=CIRCLE ( 'NONE', #9698, 71.99999999999998579 ) ;
#10187=FACE_OUTER_BOUND ( 'NONE', #4406, .T. ) ;
#10188=CARTESIAN_POINT ( 'NONE',  ( -8.385254915620292238, 43.60378069071538221, -7.699803463976802609E-17 ) ) ;
#10189=VECTOR ( 'NONE', #13417, 1000.000000000000000 ) ;
#10190=VERTEX_POINT ( 'NONE', #5650 ) ;
#10192=VERTEX_POINT ( 'NONE', #4599 ) ;
#10193=CARTESIAN_POINT ( 'NONE',  ( 0.2490282479001026672, -158.6998983971402026, 1.476456505561915877 ) ) ;
#10194=AXIS2_PLACEMENT_3D ( 'NONE', #10202, #7108, #11382 ) ;
#10196=CARTESIAN_POINT ( 'NONE',  ( -3.658761532827469409, -133.3911832492017595, 0.09517750528092941420 ) ) ;
#10202=CARTESIAN_POINT ( 'NONE',  ( -1.288514859053046853E-15, 46.06057977201469100, -8.133639011647813827E-17 ) ) ;
#10203=CARTESIAN_POINT ( 'NONE',  ( 0.3257135472934549747, -142.6406298964565451, 2.652232148860325101 ) ) ;
#10204=CARTESIAN_POINT ( 'NONE',  ( 14.13596196814457606, -39.17949320881311337, 0.000000000000000000 ) ) ;
#10209=FACE_OUTER_BOUND ( 'NONE', #4612, .T. ) ;
#10213=EDGE_CURVE ( 'NONE', #2480, #4529, #936, .T. ) ;
#10214=VERTEX_POINT ( 'NONE', #3690 ) ;
#10215=CARTESIAN_POINT ( 'NONE',  ( -8.385254915620288685, 53.02855864072483882, -16.77050983124058092 ) ) ;
#10217=CARTESIAN_POINT ( 'NONE',  ( 14.14432607165388056, -111.7272727272740838, -3.395498375151920101 ) ) ;
#10221=ORIENTED_EDGE ( 'NONE', *, *, #8327, .F. ) ;
#10222=CARTESIAN_POINT ( 'NONE',  ( -4.658052367537133698, 90.49197326372723182, -1.819943918220761514 ) ) ;
#10224=CARTESIAN_POINT ( 'NONE',  ( 2.139171521560111700, -164.3636363655099615, 0.7092570206224070306 ) ) ;
#10228=CARTESIAN_POINT ( 'NONE',  ( 10.09953664735706447, -70.24026703789812132, 0.01926284265930006817 ) ) ;
#10234=CARTESIAN_POINT ( 'NONE',  ( -8.385254915620294014, -34.41905512736551032, -16.77050983124059869 ) ) ;
#10235=AXIS2_PLACEMENT_3D ( 'NONE', #346, #3766, #12406 ) ;
#10239=CARTESIAN_POINT ( 'NONE',  ( -2.835131095452588124, -107.5510716257525843, 6.137765108552229343 ) ) ;
#10246=CARTESIAN_POINT ( 'NONE',  ( -8.385254915620294014, 90.00000000000000000, -1.589271161308885878E-16 ) ) ;
#10247=ORIENTED_EDGE ( 'NONE', *, *, #12955, .T. ) ;
#10248=CARTESIAN_POINT ( 'NONE',  ( 9.515638018240474949, -70.53215315925814366, 3.421011899655237887 ) ) ;
#10251=CARTESIAN_POINT ( 'NONE',  ( -8.385254915620290461, -15.56949922734665748, -16.77050983124058803 ) ) ;
#10252=CARTESIAN_POINT ( 'NONE',  ( 0.8583871962662020794, -102.5454545454553568, 7.611802117357260755 ) ) ;
#10254=B_SPLINE_CURVE_WITH_KNOTS ( 'NONE', 3,
 ( #5934, #10204, #8368, #7374 ),
 .UNSPECIFIED., .F., .F.,
 ( 4, 4 ),
 ( 0.000000000000000000, 1.000000000000000000 ),
 .UNSPECIFIED. ) ;
#10256=SURFACE_STYLE_USAGE ( .BOTH. , #5768 ) ;
#10257=ORIENTED_EDGE ( 'NONE', *, *, #9699, .F. ) ;
#10259=ORIENTED_EDGE ( 'NONE', *, *, #7336, .T. ) ;
#10261=CARTESIAN_POINT ( 'NONE',  ( 0.3820449743694532829, -101.7806079922463169, -7.430334148094327240 ) ) ;
#10264=CARTESIAN_POINT ( 'NONE',  ( -8.385254915620297567, 31.55439052270045508, -5.572053652267360357E-17 ) ) ;
#10265=CARTESIAN_POINT ( 'NONE',  ( -2.517691654963332357E-15, 90.00000000000000000, -1.589271161308885878E-16 ) ) ;
#10266=CARTESIAN_POINT ( 'NONE',  ( 25.00000000000000355, 120.0000000000000284, -0.5000000000000000000 ) ) ;
#10267=CARTESIAN_POINT ( 'NONE',  ( 1.640938733393168425, -125.5689954488632907, -4.287054131913241584 ) ) ;
#10268=EDGE_CURVE ( 'NONE', #5587, #11738, #10155, .T. ) ;
#10269=CARTESIAN_POINT ( 'NONE',  ( 4.338055960494658692, 91.73205429892865936, -2.486400748338238653 ) ) ;
#10274=FACE_OUTER_BOUND ( 'NONE', #7934, .T. ) ;
#10276=CARTESIAN_POINT ( 'NONE',  ( 12.99579180576516180, 64.08350967699263379, 25.99158361153034136 ) ) ;
#10278=VERTEX_POINT ( 'NONE', #1734 ) ;
#10279=CARTESIAN_POINT ( 'NONE',  ( 8.385254915620290461, 53.02855864072483882, -16.77050983124057737 ) ) ;
#10281=CARTESIAN_POINT ( 'NONE',  ( 3.682460330391462033, -161.0909090907768189, 2.758257593130142737 ) ) ;
#10283=CIRCLE ( 'NONE', #12061, 77.99999999999997158 ) ;
#10284=ORIENTED_EDGE ( 'NONE', *, *, #10213, .T. ) ;
#10285=CARTESIAN_POINT ( 'NONE',  ( -4.696484759529494291, 90.40938722714874132, -1.719265504264336109 ) ) ;
#10287=EDGE_CURVE ( 'NONE', #2229, #13867, #4128, .T. ) ;
#10290=DIRECTION ( 'NONE',  ( -1.000000000000000000, 0.000000000000000000, 0.000000000000000000 ) ) ;
#10295=DIRECTION ( 'NONE',  ( 0.000000000000000000, 0.000000000000000000, -1.000000000000000000 ) ) ;
#10296=EDGE_LOOP ( 'NONE', ( #9491, #10259, #10767, #6649 ) ) ;
#10298=ORIENTED_EDGE ( 'NONE', *, *, #6602, .T. ) ;
#10299=CARTESIAN_POINT ( 'NONE',  ( -5.384951958016893414, -83.47453208601771735, 7.985098097371742476 ) ) ;
#10301=AXIS2_PLACEMENT_3D ( 'NONE', #475, #6901, #5870 ) ;
#10302=ORIENTED_EDGE ( 'NONE', *, *, #375, .T. ) ;
#10304=ORIENTED_EDGE ( 'NONE', *, *, #11404, .T. ) ;
#10307=ADVANCED_FACE ( 'NONE', ( #8184 ), #12468, .T. ) ;
#10308=CARTESIAN_POINT ( 'NONE',  ( -10.00000000000000000, 99.99999999999994316, -0.5000000000000000000 ) ) ;
#10311=CARTESIAN_POINT ( 'NONE',  ( -5.225617147457730205, -118.1447657390923922, -1.522498834799536294 ) ) ;
#10317=VERTEX_POINT ( 'NONE', #12610 ) ;
#10318=CARTESIAN_POINT ( 'NONE',  ( -4.231485814931500222, 91.18833760977217651, -2.665113332093635101 ) ) ;
#10319=CARTESIAN_POINT ( 'NONE',  ( -35.20000000000000995, 106.4000000000000199, 2.500000000000000000 ) ) ;
#10320=EDGE_LOOP ( 'NONE', ( #10678, #1911, #13279, #6936 ) ) ;
#10321=CARTESIAN_POINT ( 'NONE',  ( 4.867363524069543423, 90.10434700764739091, 1.150748602993065139 ) ) ;
#10322=( NAMED_UNIT ( * ) SI_UNIT ( $, .STERADIAN. ) SOLID_ANGLE_UNIT ( ) );
#10323=VECTOR ( 'NONE', #6985, 1000.000000000000114 ) ;
#10324=CARTESIAN_POINT ( 'NONE',  ( 12.99579180576516535, 45.23395377697384134, 3.183050967463142591E-15 ) ) ;
#10326=ADVANCED_FACE ( 'NONE', ( #11744 ), #889, .T. ) ;
#10329=DIRECTION ( 'NONE',  ( -0.000000000000000000, -0.000000000000000000, -1.000000000000000000 ) ) ;
#10335=CARTESIAN_POINT ( 'NONE',  ( 3.943110440846829157, -117.6640828201278026, 3.845144683265616870 ) ) ;
#10336=AXIS2_PLACEMENT_3D ( 'NONE', #673, #746, #11189 ) ;
#10338=CARTESIAN_POINT ( 'NONE',  ( -12.99553232110414314, 29.92431064457076673, -1.697177803646649065E-15 ) ) ;
#10342=CARTESIAN_POINT ( 'NONE',  ( -0.6786374973538379374, -157.4026716423472294, -1.357839624991837413 ) ) ;
#10343=CARTESIAN_POINT ( 'NONE',  ( 0.1852016367018599341, -70.00000000000000000, -1.488522876466113365 ) ) ;
#10345=DIRECTION ( 'NONE',  ( -2.797435172181481150E-17, 1.000000000000000000, -1.765856845898762549E-18 ) ) ;
#10347=CARTESIAN_POINT ( 'NONE',  ( -2.517691654963332357E-15, 90.00000000000000000, -1.589271161308885878E-16 ) ) ;
#10351=CARTESIAN_POINT ( 'NONE',  ( -10.00000000000000711, 139.9999999999999716, 0.5000000000000000000 ) ) ;
#10353=CARTESIAN_POINT ( 'NONE',  ( 54.35437857507979231, -62.63636364489408237, 19.28415345520743429 ) ) ;
#10355=ORIENTED_EDGE ( 'NONE', *, *, #7990, .F. ) ;
#10356=CARTESIAN_POINT ( 'NONE',  ( -4.867363524069549641, 90.10434700764739091, -1.150748602993065139 ) ) ;
#10358=CARTESIAN_POINT ( 'NONE',  ( 9.412634226148496097, -71.99999999999992895, 5.970118669234167008 ) ) ;
#10359=CARTESIAN_POINT ( 'NONE',  ( -11.72298137502696669, -168.9999999999999147, -2.970135970081303256 ) ) ;
#10360=CARTESIAN_POINT ( 'NONE',  ( 15.29705854078138394, 38.52236939141059935, 1.806990092252540040E-15 ) ) ;
#10362=FACE_OUTER_BOUND ( 'NONE', #12298, .T. ) ;
#10363=UNCERTAINTY_MEASURE_WITH_UNIT (LENGTH_MEASURE( 1.000000000000000082E-05 ), #3864, 'distance_accuracy_value', 'NONE');
#10364=DIRECTION ( 'NONE',  ( 2.797435172181480534E-17, -1.000000000000000000, 1.765856845898762164E-18 ) ) ;
#10366=EDGE_LOOP ( 'NONE', ( #11588, #5726 ) ) ;
#10368=ORIENTED_EDGE ( 'NONE', *, *, #9886, .F. ) ;
#10369=CARTESIAN_POINT ( 'NONE',  ( -15.29705854078139282, -19.91286587805129926, -30.59411708156279630 ) ) ;
#10373=DIRECTION ( 'NONE',  ( -2.797435172181481150E-17, 1.000000000000000000, -1.765856845898762549E-18 ) ) ;
#10374=CARTESIAN_POINT ( 'NONE',  ( -2.715682715547387271, -123.3573972935287202, -4.033725032893866747 ) ) ;
#10376=DIRECTION ( 'NONE',  ( -2.797435172181481150E-17, 1.000000000000000000, -1.765856845898762549E-18 ) ) ;
#10377=VERTEX_POINT ( 'NONE', #7260 ) ;
#10383=CARTESIAN_POINT ( 'NONE',  ( -15.29705854078139815, -8.601520358636511432, 30.59411708156277854 ) ) ;
#10384=ADVANCED_FACE ( 'NONE', ( #13755 ), #9574, .F. ) ;
#10387=CARTESIAN_POINT ( 'NONE',  ( -3.288118420601238601, 90.13403546913524167, -3.770150660886110838 ) ) ;
#10389=CARTESIAN_POINT ( 'NONE',  ( -11.81226048336476353, -40.00941361824966691, -23.62452096672953772 ) ) ;
#10394=DIRECTION ( 'NONE',  ( 0.000000000000000000, 0.000000000000000000, 1.000000000000000000 ) ) ;
#10396=CARTESIAN_POINT ( 'NONE',  ( -1.487915231218352785, -147.9615408504190270, -1.535193590670937969 ) ) ;
#10398=ORIENTED_EDGE ( 'NONE', *, *, #368, .T. ) ;
#10400=ORIENTED_EDGE ( 'NONE', *, *, #2150, .F. ) ;
#10401=B_SPLINE_CURVE_WITH_KNOTS ( 'NONE', 3,
 ( #9514, #3123, #2932, #3978 ),
 .UNSPECIFIED., .F., .F.,
 ( 4, 4 ),
 ( 0.000000000000000000, 1.000000000000000000 ),
 .UNSPECIFIED. ) ;
#10402=DIRECTION ( 'NONE',  ( -2.797435172181481150E-17, 1.000000000000000000, -1.765856845898762549E-18 ) ) ;
#10403=ADVANCED_FACE ( 'NONE', ( #12890 ), #1028, .T. ) ;
#10404=DIRECTION ( 'NONE',  ( -2.797435172181481150E-17, 1.000000000000000000, -1.765856845898762549E-18 ) ) ;
#10406=CARTESIAN_POINT ( 'NONE',  ( -5.389985679975356270, -107.9165190526823039, 3.974935440706736323 ) ) ;
#10408=CARTESIAN_POINT ( 'NONE',  ( 0.3668613529500256987, -160.9696969691409549, -1.703459722499988338 ) ) ;
#10409=DIRECTION ( 'NONE',  ( -2.797435172181481150E-17, 1.000000000000000000, -1.765856845898762549E-18 ) ) ;
#10410=CARTESIAN_POINT ( 'NONE',  ( 10.69346802281034670, 21.32451227372186864, -21.38693604562068273 ) ) ;
#10411=CARTESIAN_POINT ( 'NONE',  ( 3.621248221984613947E-16, -12.94488700934118341, 2.285881734483108495E-17 ) ) ;
#10417=CARTESIAN_POINT ( 'NONE',  ( 3.036220672062631021, -100.2727272727342580, 3.474096187148000503 ) ) ;
#10421=DIRECTION ( 'NONE',  ( -1.000000000000000000, 0.000000000000000000, 0.000000000000000000 ) ) ;
#10422=ORIENTED_EDGE ( 'NONE', *, *, #3858, .F. ) ;
#10423=DIRECTION ( 'NONE',  ( 9.860761315262647568E-32, 3.204747427460360459E-31, -1.000000000000000000 ) ) ;
#10426=( BOUNDED_SURFACE ( )  B_SPLINE_SURFACE ( 3, 3, ( 
 ( #2137, #9787, #7533, #5427 ),
 ( #2341, #1172, #10755, #10687 ),
 ( #8656, #7671, #7400, #11682 ),
 ( #1099, #5358, #57, #4310 ) ),
 .UNSPECIFIED., .F., .F., .F. ) 
 B_SPLINE_SURFACE_WITH_KNOTS ( ( 4, 4 ),
 ( 4, 4 ),
 ( 0.000000000000000000, 1.000000000000000000 ),
 ( 0.000000000000000000, 1.000000000000000000 ),
 .UNSPECIFIED. ) 
 GEOMETRIC_REPRESENTATION_ITEM ( )  RATIONAL_B_SPLINE_SURFACE ( (
 ( 1.000000000000000000, 0.3333333333333334259, 0.3333333333333334259, 1.000000000000000000),
 ( 1.000000000000000000, 0.3333333333333334259, 0.3333333333333334259, 1.000000000000000000),
 ( 1.000000000000000000, 0.3333333333333334259, 0.3333333333333334259, 1.000000000000000000),
 ( 1.000000000000000000, 0.3333333333333334259, 0.3333333333333334259, 1.000000000000000000) ) ) 
 REPRESENTATION_ITEM ( '' )  SURFACE ( )  );
#10427=CARTESIAN_POINT ( 'NONE',  ( 4.154595973944849696, -168.9999999999999432, -0.9946518452610428884 ) ) ;
#10428=DIRECTION ( 'NONE',  ( 0.000000000000000000, 0.000000000000000000, 1.000000000000000000 ) ) ;
#10429=CIRCLE ( 'NONE', #13826, 15.29705854078138749 ) ;
#10430=DIRECTION ( 'NONE',  ( 2.797435172181479917E-17, -1.000000000000000000, 1.765856845898779112E-18 ) ) ;
#10431=CARTESIAN_POINT ( 'NONE',  ( 12.97449437267217753, -39.59556244224027211, 3.177834600809665306E-15 ) ) ;
#10432=MECHANICAL_DESIGN_GEOMETRIC_PRESENTATION_REPRESENTATION('',(#3700),#4147);
#10435=CARTESIAN_POINT ( 'NONE',  ( -7.925252723941369482, -86.41510259838975117, 5.018155542691334681 ) ) ;
#10437=ORIENTED_EDGE ( 'NONE', *, *, #2791, .F. ) ;
#10438=FACE_OUTER_BOUND ( 'NONE', #4177, .T. ) ;
#10440=ADVANCED_FACE ( 'NONE', ( #960 ), #5355, .T. ) ;
#10441=CARTESIAN_POINT ( 'NONE',  ( 12.99553232110414136, 29.92431064457076673, 1.549257345293556973E-15 ) ) ;
#10443=CARTESIAN_POINT ( 'NONE',  ( 0.3898256620743995593, -154.2032979590117918, 1.618808203873735030 ) ) ;
#10444=CARTESIAN_POINT ( 'NONE',  ( 12.99553232110414314, 48.77386654458962312, -25.99106464220827561 ) ) ;
#10447=EDGE_LOOP ( 'NONE', ( #6616, #3426, #570, #8471, #13426, #6750, #10302 ) ) ;
#10448=ORIENTED_EDGE ( 'NONE', *, *, #6337, .F. ) ;
#10451=ORIENTED_EDGE ( 'NONE', *, *, #4923, .F. ) ;
#10452=CARTESIAN_POINT ( 'NONE',  ( -8.385254915620295790, 78.67828027274755698, -16.77050983124059513 ) ) ;
#10454=CARTESIAN_POINT ( 'NONE',  ( 25.00000000000000355, 120.0000000000000284, 2.500000000000000000 ) ) ;
#10456=CARTESIAN_POINT ( 'NONE',  ( -9.841394828007315354, -91.60173160170883477, -2.396245945941702704 ) ) ;
#10458=EDGE_CURVE ( 'NONE', #4633, #2958, #7269, .T. ) ;
#10460=DIRECTION ( 'NONE',  ( 2.797435172181480534E-17, -1.000000000000000000, 1.765856845898762164E-18 ) ) ;
#10461=CARTESIAN_POINT ( 'NONE',  ( -2.440375224551862843, -143.3570535663918122, -0.8181369023438933574 ) ) ;
#10462=CARTESIAN_POINT ( 'NONE',  ( 15.29705854078138749, 17.78624592198638155, 1.840275709580739737E-15 ) ) ;
#10463=ORIENTED_EDGE ( 'NONE', *, *, #9804, .T. ) ;
#10466=DIRECTION ( 'NONE',  ( 1.000000000000000000, 1.665334536937735599E-15, 0.000000000000000000 ) ) ;
#10467=CARTESIAN_POINT ( 'NONE',  ( 0.7814938847207267836, -100.6906014649701433, 7.534213779343278183 ) ) ;
#10468=CARTESIAN_POINT ( 'NONE',  ( -0.5078243831721187540, -154.2164502162252404, -1.847253022830592561 ) ) ;
#10469=FACE_OUTER_BOUND ( 'NONE', #4316, .T. ) ;
#10470=EDGE_CURVE ( 'NONE', #2108, #9893, #11529, .T. ) ;
#10471=DIRECTION ( 'NONE',  ( 1.000000000000000000, 3.568574007723717789E-15, 0.000000000000000000 ) ) ;
#10475=FACE_OUTER_BOUND ( 'NONE', #7815, .T. ) ;
#10476=EDGE_CURVE ( 'NONE', #887, #9797, #13576, .T. ) ;
#10478=VERTEX_POINT ( 'NONE', #9845 ) ;
#10481=CARTESIAN_POINT ( 'NONE',  ( 3.894934744998975518, -89.44155844158821367, -2.935215040338265968 ) ) ;
#10482=ORIENTED_EDGE ( 'NONE', *, *, #9224, .F. ) ;
#10489=CARTESIAN_POINT ( 'NONE',  ( -12.05891082652281199, -95.36363636363795138, -5.087868926931797375 ) ) ;
#10490=AXIS2_PLACEMENT_3D ( 'NONE', #11149, #1466, #10098 ) ;
#10492=CARTESIAN_POINT ( 'NONE',  ( -12.99553232110414491, 48.77386654458962312, 25.99106464220826851 ) ) ;
#10494=CARTESIAN_POINT ( 'NONE',  ( 15.29705854078138394, -36.87585420866476937, 30.59411708156277854 ) ) ;
#10495=CARTESIAN_POINT ( 'NONE',  ( -4.866961404864796670, 90.10495303670558087, 1.152376359967959063 ) ) ;
#10497=EDGE_LOOP ( 'NONE', ( #10774, #12220, #2940, #1949 ) ) ;
#10498=CARTESIAN_POINT ( 'NONE',  ( -1.433044453979095634, -80.32154590898655044, 10.00519026140878864 ) ) ;
#10500=CARTESIAN_POINT ( 'NONE',  ( 12.99579180576517423, -20.73949187309215247, 1.656338139122241719E-15 ) ) ;
#10504=CARTESIAN_POINT ( 'NONE',  ( 1.781428662358381487, -131.6218529372965804, -3.442014977257640940 ) ) ;
#10508=CARTESIAN_POINT ( 'NONE',  ( 15.29705854078139460, -8.601520358636511432, 3.746698755667523200E-15 ) ) ;
#10514=CARTESIAN_POINT ( 'NONE',  ( 12.99553232110413781, 77.04820039461787928, 1.478563310446379610E-15 ) ) ;
#10521=CARTESIAN_POINT ( 'NONE',  ( 8.385254915620294014, 69.25350232273815720, -16.77050983124058448 ) ) ;
#10523=CARTESIAN_POINT ( 'NONE',  ( 3.721216335461446700, -108.7938388513467061, -5.424520069322383620 ) ) ;
#10524=DIRECTION ( 'NONE',  ( -1.000000000000000000, 0.000000000000000000, 0.000000000000000000 ) ) ;
#10525=ORIENTED_EDGE ( 'NONE', *, *, #11002, .T. ) ;
#10526=CIRCLE ( 'NONE', #12334, 16.99999999999998934 ) ;
#10531=EDGE_CURVE ( 'NONE', #12589, #4671, #1681, .T. ) ;
#10535=CARTESIAN_POINT ( 'NONE',  ( 2.780317640840915594, -98.85838219806488780, 7.289431051163909991 ) ) ;
#10539=CARTESIAN_POINT ( 'NONE',  ( 15.29705854078139460, 64.91013567203349055, -30.59411708156277854 ) ) ;
#10540=DIRECTION ( 'NONE',  ( -1.000000000000000000, 0.000000000000000000, 0.000000000000000000 ) ) ;
#10543=CARTESIAN_POINT ( 'NONE',  ( 8.385254915620292238, 69.25350232273815720, 9.022884433393300556E-16 ) ) ;
#10547=EDGE_CURVE ( 'NONE', #3686, #13516, #4099, .T. ) ;
#10550=CARTESIAN_POINT ( 'NONE',  ( 6.062451257354256384, -129.7272727272775512, -11.56901651898783001 ) ) ;
#10553=CARTESIAN_POINT ( 'NONE',  ( 15.29705854078138749, -10.48808792804187284, 30.59411708156277854 ) ) ;
#10555=ORIENTED_EDGE ( 'NONE', *, *, #4190, .F. ) ;
#10557=EDGE_CURVE ( 'NONE', #1069, #9187, #4568, .T. ) ;
#10559=CARTESIAN_POINT ( 'NONE',  ( 7.328281203649089193, -76.12121211817229494, 4.753922619608384359 ) ) ;
#10560=CARTESIAN_POINT ( 'NONE',  ( -2.247751904815863622, -65.63636362841093330, 0.1634371276632270997 ) ) ;
#10563=CARTESIAN_POINT ( 'NONE',  ( 10.69381717166375800, -21.56444287793185666, 2.619229793989004345E-15 ) ) ;
#10564=CARTESIAN_POINT ( 'NONE',  ( -15.29705854078139282, -36.87585420866476937, 30.59411708156277498 ) ) ;
#10565=CARTESIAN_POINT ( 'NONE',  ( -4.367873154833913141, 91.47215508561177444, 2.433639722925613924 ) ) ;
#10566=ORIENTED_EDGE ( 'NONE', *, *, #8259, .T. ) ;
#10568=CIRCLE ( 'NONE', #511, 8.385254915620290461 ) ;
#10570=ORIENTED_EDGE ( 'NONE', *, *, #701, .F. ) ;
#10571=CARTESIAN_POINT ( 'NONE',  ( 8.385254915620295790, -12.94488700934118341, -16.77050983124058448 ) ) ;
#10572=CARTESIAN_POINT ( 'NONE',  ( -8.385254915620295790, 69.25350232273815720, -1.271481101603046320E-15 ) ) ;
#10573=CARTESIAN_POINT ( 'NONE',  ( -15.29705854078139815, 55.48535772202409788, 30.59411708156277854 ) ) ;
#10574=LINE ( 'NONE', #10308, #1798 ) ;
#10575=CARTESIAN_POINT ( 'NONE',  ( 0.4884533741263017981, -128.8023475767107016, -4.172574844680278616 ) ) ;
#10576=LINE ( 'NONE', #713, #7789 ) ;
#10578=ORIENTED_EDGE ( 'NONE', *, *, #7132, .F. ) ;
#10580=( BOUNDED_SURFACE ( )  B_SPLINE_SURFACE ( 3, 3, ( 
 ( #498, #4760, #4963, #9242 ),
 ( #13348, #3908, #7982, #12260 ),
 ( #11341, #2647, #564, #4830 ),
 ( #13421, #12332, #1799, #8187 ) ),
 .UNSPECIFIED., .F., .F., .F. ) 
 B_SPLINE_SURFACE_WITH_KNOTS ( ( 4, 4 ),
 ( 4, 4 ),
 ( 0.000000000000000000, 1.000000000000000000 ),
 ( 0.000000000000000000, 1.000000000000000000 ),
 .UNSPECIFIED. ) 
 GEOMETRIC_REPRESENTATION_ITEM ( )  RATIONAL_B_SPLINE_SURFACE ( (
 ( 1.000000000000000000, 0.3333333333333334259, 0.3333333333333334259, 1.000000000000000000),
 ( 1.000000000000000000, 0.3333333333333334259, 0.3333333333333334259, 1.000000000000000000),
 ( 1.000000000000000000, 0.3333333333333334259, 0.3333333333333334259, 1.000000000000000000),
 ( 1.000000000000000000, 0.3333333333333334259, 0.3333333333333334259, 1.000000000000000000) ) ) 
 REPRESENTATION_ITEM ( '' )  SURFACE ( )  );
#10583=DIRECTION ( 'NONE',  ( -0.000000000000000000, -0.000000000000000000, -1.000000000000000000 ) ) ;
#10585=CARTESIAN_POINT ( 'NONE',  ( -15.29705854078138394, -38.76242177807012723, -30.59411708156277854 ) ) ;
#10586=ORIENTED_EDGE ( 'NONE', *, *, #12304, .F. ) ;
#10593=CARTESIAN_POINT ( 'NONE',  ( -1.952880862260572670, -132.1386478743458781, 3.257033108385012365 ) ) ;
#10594=DIRECTION ( 'NONE',  ( 0.000000000000000000, 1.000000000000000000, -0.000000000000000000 ) ) ;
#10596=ORIENTED_EDGE ( 'NONE', *, *, #255, .F. ) ;
#10598=CARTESIAN_POINT ( 'NONE',  ( -1.246623049074521372, -140.6414058277869970, -2.594349448477115683 ) ) ;
#10599=VECTOR ( 'NONE', #923, 1000.000000000000000 ) ;
#10603=CARTESIAN_POINT ( 'NONE',  ( -5.190364408751921843, -107.5279543462731056, 4.303367517544086418 ) ) ;
#10606=CARTESIAN_POINT ( 'NONE',  ( -8.385254915620294014, 22.12961257269105531, -2.113820870476202140E-15 ) ) ;
#10609=FACE_OUTER_BOUND ( 'NONE', #13793, .T. ) ;
#10611=LINE ( 'NONE', #1996, #237 ) ;
#10612=CARTESIAN_POINT ( 'NONE',  ( -4.980291965142432886, -118.2727272727225483, -1.265069668247100543 ) ) ;
#10613=ORIENTED_EDGE ( 'NONE', *, *, #11278, .T. ) ;
#10614=DIRECTION ( 'NONE',  ( 1.000000000000000000, 1.850371707708595154E-15, 0.000000000000000000 ) ) ;
#10617=DIRECTION ( 'NONE',  ( 1.000000000000000000, 0.000000000000000000, 0.000000000000000000 ) ) ;
#10620=CARTESIAN_POINT ( 'NONE',  ( 8.931512003261595112, -153.6493506494127814, -10.28374512068234559 ) ) ;
#10621=EDGE_CURVE ( 'NONE', #10825, #6779, #3016, .T. ) ;
#10622=CARTESIAN_POINT ( 'NONE',  ( -15.29705854078139105, -10.48808792804187284, 1.852046186812095429E-17 ) ) ;
#10623=CARTESIAN_POINT ( 'NONE',  ( 12.99553232110414314, 11.07475474455194053, -25.99106464220826851 ) ) ;
#10626=CYLINDRICAL_SURFACE ( 'NONE', #13768, 5.000000000000000000 ) ;
#10627=DIRECTION ( 'NONE',  ( 0.000000000000000000, 0.000000000000000000, 1.000000000000000000 ) ) ;
#10637=CARTESIAN_POINT ( 'NONE',  ( -15.29705854078138394, 29.09759144140119957, -30.59411708156277854 ) ) ;
#10640=DIRECTION ( 'NONE',  ( -2.797435172181481150E-17, 1.000000000000000000, -1.765856845898762549E-18 ) ) ;
#10643=EDGE_CURVE ( 'NONE', #10377, #7475, #1356, .T. ) ;
#10647=VECTOR ( 'NONE', #4548, 1000.000000000000000 ) ;
#10648=DIRECTION ( 'NONE',  ( -2.797435172181481150E-17, 1.000000000000000000, -1.765856845898762549E-18 ) ) ;
#10649=CARTESIAN_POINT ( 'NONE',  ( 9.701113296676155073, -69.00000000000008527, 3.021359762293434503 ) ) ;
#10651=CARTESIAN_POINT ( 'NONE',  ( -10.69381717166375623, 72.68333662216238622, -1.566311632108520979E-15 ) ) ;
#10652=DIRECTION ( 'NONE',  ( -0.4545454545454531425, -0.8907235428302472391, 0.000000000000000000 ) ) ;
#10656=CARTESIAN_POINT ( 'NONE',  ( 12.99553232110413781, 67.62342244460847951, 1.492702117415814531E-15 ) ) ;
#10657=CARTESIAN_POINT ( 'NONE',  ( 0.07095332755016135751, -158.6814110685799051, -1.494078031317318755 ) ) ;
#10661=VERTEX_POINT ( 'NONE', #6837 ) ;
#10667=CARTESIAN_POINT ( 'NONE',  ( -12.99553232110413781, 39.34908859458022334, -3.265581959298969830E-15 ) ) ;
#10668=CARTESIAN_POINT ( 'NONE',  ( -2.094721958917744153, -120.2871812560114506, -4.762225812260485469 ) ) ;
#10669=CARTESIAN_POINT ( 'NONE',  ( 15.29705854078139815, -8.601520358636511432, -30.59411708156277854 ) ) ;
#10670=CARTESIAN_POINT ( 'NONE',  ( 1.109824446840197210, -148.3982683987656799, -1.619194360870498173 ) ) ;
#10671=CARTESIAN_POINT ( 'NONE',  ( -12.99579180576516535, 64.08350967699263379, -25.99158361153034136 ) ) ;
#10673=CARTESIAN_POINT ( 'NONE',  ( -7.783279735887626671, -74.45454545454313688, -6.359494517302866967 ) ) ;
#10678=ORIENTED_EDGE ( 'NONE', *, *, #2327, .T. ) ;
#10679=VERTEX_POINT ( 'NONE', #11032 ) ;
#10680=CARTESIAN_POINT ( 'NONE',  ( 8.385254915620294014, 24.75422479069652582, 9.855024866598292994E-16 ) ) ;
#10681=VERTEX_POINT ( 'NONE', #11116 ) ;
#10684=CARTESIAN_POINT ( 'NONE',  ( 12.99579180576516180, 26.38439787695498495, 25.99158361153033425 ) ) ;
#10687=CARTESIAN_POINT ( 'NONE',  ( -12.99579180576517068, 26.38439787695498495, -3.233995902620226781E-15 ) ) ;
#10691=PLANE ( 'NONE',  #11836 ) ;
#10696=FACE_OUTER_BOUND ( 'NONE', #4248, .T. ) ;
#10699=CARTESIAN_POINT ( 'NONE',  ( -10.07809618140513663, -70.83793457579116648, -0.9291402644571875591 ) ) ;
#10701=AXIS2_PLACEMENT_3D ( 'NONE', #8207, #5048, #1821 ) ;
#10702=DIRECTION ( 'NONE',  ( -2.797435172181481150E-17, 1.000000000000000000, -1.765856845898762549E-18 ) ) ;
#10706=ADVANCED_FACE ( 'NONE', ( #610 ), #12448, .T. ) ;
#10707=EDGE_CURVE ( 'NONE', #12700, #6483, #13686, .T. ) ;
#10708=ORIENTED_EDGE ( 'NONE', *, *, #5903, .F. ) ;
#10714=CARTESIAN_POINT ( 'NONE',  ( -3.656918945275430932, -76.68408302446904656, -9.436988915889060081 ) ) ;
#10715=DIRECTION ( 'NONE',  ( -2.797435172181481150E-17, 1.000000000000000000, -1.765856845898762549E-18 ) ) ;
#10717=CARTESIAN_POINT ( 'NONE',  ( -6.423503816350314644, -86.98444705607441563, 6.714555888684349050 ) ) ;
#10718=DIRECTION ( 'NONE',  ( 0.000000000000000000, 0.000000000000000000, 1.000000000000000000 ) ) ;
#10723=AXIS2_PLACEMENT_3D ( 'NONE', #2783, #10148, #9094 ) ;
#10724=ADVANCED_FACE ( 'NONE', ( #11791 ), #11402, .T. ) ;
#10725=CARTESIAN_POINT ( 'NONE',  ( -3.286535165834789662, 90.13351245737436557, 3.771524672989932547 ) ) ;
#10728=CARTESIAN_POINT ( 'NONE',  ( 15.29705854078139282, -1.063309978032445091, 3.746698755667523200E-15 ) ) ;
#10729=CARTESIAN_POINT ( 'NONE',  ( 15.29705854078138572, 38.52236939141059935, 1.806990092252540040E-15 ) ) ;
#10738=CARTESIAN_POINT ( 'NONE',  ( 2.224254061606619093, -80.66666666666661456, -9.925145656127773108 ) ) ;
#10739=CIRCLE ( 'NONE', #4465, 8.385254915620292238 ) ;
#10740=CARTESIAN_POINT ( 'NONE',  ( -10.69346802281034670, -16.37459952631584059, -1.251741741247135829E-15 ) ) ;
#10742=ORIENTED_EDGE ( 'NONE', *, *, #1818, .F. ) ;
#10745=CIRCLE ( 'NONE', #692, 8.385254915620294014 ) ;
#10747=AXIS2_PLACEMENT_3D ( 'NONE', #12516, #13397, #13317 ) ;
#10749=EDGE_LOOP ( 'NONE', ( #10482, #3660, #6447, #2896, #441, #7732 ) ) ;
#10751=DIRECTION ( 'NONE',  ( -1.000000000000000000, 0.000000000000000000, 0.000000000000000000 ) ) ;
#10754=CIRCLE ( 'NONE', #2719, 11.81226048336476886 ) ;
#10755=CARTESIAN_POINT ( 'NONE',  ( -12.99579180576516535, 26.38439787695498495, -25.99158361153034136 ) ) ;
#10758=DIRECTION ( 'NONE',  ( -1.000000000000000000, 0.000000000000000000, 0.000000000000000000 ) ) ;
#10759=B_SPLINE_CURVE_WITH_KNOTS ( 'NONE', 3,
 ( #11120, #7891, #2087, #12839, #1437, #8951, #5311, #5243, #3205, #9591, #5714, #13257, #10770, #6197, #9528, #7483, #2152, #6437, #8872, #13182, #10699, #12172, #13840, #12098 ),
 .UNSPECIFIED., .F., .F.,
 ( 4, 2, 2, 2, 2, 2, 2, 2, 2, 2, 2, 4 ),
 ( 0.000000000000000000, 0.002159622253435538111, 0.003239433380153306733, 0.004319244506871076222, 0.006478866760306590915, 0.008638489013742107342, 0.01079811126717762637, 0.01295773352061314540, 0.01403754464733089277, 0.01511735577404864188, 0.01619716690076638752, 0.01727697802748413489 ),
 .UNSPECIFIED. ) ;
#10761=CARTESIAN_POINT ( 'NONE',  ( -1.747091603990086329E-15, 62.45333659073423860, -1.102836519679677113E-16 ) ) ;
#10762=B_SPLINE_CURVE_WITH_KNOTS ( 'NONE', 3,
 ( #4902, #11354, #7923, #12349 ),
 .UNSPECIFIED., .F., .F.,
 ( 4, 4 ),
 ( 0.000000000000000000, 1.000000000000000000 ),
 .UNSPECIFIED. ) ;
#10763=VERTEX_POINT ( 'NONE', #169 ) ;
#10765=ORIENTED_EDGE ( 'NONE', *, *, #9361, .F. ) ;
#10767=ORIENTED_EDGE ( 'NONE', *, *, #12699, .T. ) ;
#10769=DIRECTION ( 'NONE',  ( 0.000000000000000000, 0.000000000000000000, 1.000000000000000000 ) ) ;
#10770=CARTESIAN_POINT ( 'NONE',  ( -8.557187102284723679, -74.11437728923387169, -5.386762695872780782 ) ) ;
#10774=ORIENTED_EDGE ( 'NONE', *, *, #1141, .T. ) ;
#10776=ORIENTED_EDGE ( 'NONE', *, *, #13514, .T. ) ;
#10777=DIRECTION ( 'NONE',  ( 0.000000000000000000, 0.000000000000000000, 1.000000000000000000 ) ) ;
#10779=CARTESIAN_POINT ( 'NONE',  ( -6.850226882306651000, -73.90543885042040984, -7.468286930689518321 ) ) ;
#10781=CARTESIAN_POINT ( 'NONE',  ( -15.29705854078138394, 66.79670324143890525, -30.59411708156277498 ) ) ;
#10782=ADVANCED_FACE ( 'NONE', ( #10795 ), #3032, .T. ) ;
#10783=CARTESIAN_POINT ( 'NONE',  ( 1.574536146393409775, -80.31525646925749129, 9.985167164889261926 ) ) ;
#10785=DIRECTION ( 'NONE',  ( 0.000000000000000000, 0.000000000000000000, 1.000000000000000000 ) ) ;
#10788=VERTEX_POINT ( 'NONE', #12935 ) ;
#10789=ORIENTED_EDGE ( 'NONE', *, *, #11862, .F. ) ;
#10790=ADVANCED_FACE ( 'NONE', ( #5406 ), #8530, .T. ) ;
#10793=ORIENTED_EDGE ( 'NONE', *, *, #9722, .T. ) ;
#10794=CARTESIAN_POINT ( 'NONE',  ( 15.29705854078139815, 90.00000000000000000, 1.714422261702873752E-15 ) ) ;
#10795=FACE_OUTER_BOUND ( 'NONE', #8737, .T. ) ;
#10799=CARTESIAN_POINT ( 'NONE',  ( -1.956031471770462549, -154.2164502162973747, -1.283490743970612025 ) ) ;
#10800=CARTESIAN_POINT ( 'NONE',  ( -8.627629343136057116, -71.90909090909200074, -5.462837922541642577 ) ) ;
#10804=EDGE_LOOP ( 'NONE', ( #9622, #5993, #10950, #6593 ) ) ;
#10805=EDGE_CURVE ( 'NONE', #7777, #7988, #1909, .T. ) ;
#10806=CARTESIAN_POINT ( 'NONE',  ( 4.330127018922190985, 92.00000000000000000, 2.500000000000000000 ) ) ;
#10812=CARTESIAN_POINT ( 'NONE',  ( 15.29705854078139460, -18.02629830864596627, 1.906846944237139921E-15 ) ) ;
#10815=CARTESIAN_POINT ( 'NONE',  ( -12.99579180576517068, 54.65873172698324112, -3.291435486758484277E-15 ) ) ;
#10823=CARTESIAN_POINT ( 'NONE',  ( -9.175745902881725407E-17, 3.280056672672198914, -5.792110530374064999E-18 ) ) ;
#10825=VERTEX_POINT ( 'NONE', #9505 ) ;
#10830=CARTESIAN_POINT ( 'NONE',  ( -1.077638310512993291E-15, 38.52236939141059935, -6.802498971006334016E-17 ) ) ;
#10831=CARTESIAN_POINT ( 'NONE',  ( 8.385254915620292238, -3.520109059331727241, 1.035430912652128846E-15 ) ) ;
#10832=AXIS2_PLACEMENT_3D ( 'NONE', #3601, #4580, #7885 ) ;
#10834=CARTESIAN_POINT ( 'NONE',  ( -8.385254915620295790, 12.70483462268160046, 16.77050983124058448 ) ) ;
#10839=DIRECTION ( 'NONE',  ( -1.000000000000000000, 0.000000000000000000, 0.000000000000000000 ) ) ;
#10845=DIRECTION ( 'NONE',  ( -1.000000000000000000, -0.000000000000000000, -0.000000000000000000 ) ) ;
#10847=CARTESIAN_POINT ( 'NONE',  ( -1.087924057176452797, -78.56626508165413725, -10.04922990886309719 ) ) ;
#10850=FACE_OUTER_BOUND ( 'NONE', #3759, .T. ) ;
#10851=AXIS2_PLACEMENT_3D ( 'NONE', #1416, #7868, #8846 ) ;
#10853=ORIENTED_EDGE ( 'NONE', *, *, #4899, .F. ) ;
#10855=AXIS2_PLACEMENT_3D ( 'NONE', #6321, #6127, #860 ) ;
#10856=ADVANCED_FACE ( 'NONE', ( #2000 ), #8990, .T. ) ;
#10857=CARTESIAN_POINT ( 'NONE',  ( -4.267662252619976115, 91.33687515530510836, 2.605658972705547693 ) ) ;
#10858=EDGE_CURVE ( 'NONE', #3017, #5860, #957, .T. ) ;
#10859=CARTESIAN_POINT ( 'NONE',  ( -0.6169032162240980499, -80.00108109729535499, 10.04415339342917513 ) ) ;
#10862=CIRCLE ( 'NONE', #11769, 15.29705854078138927 ) ;
#10863=CARTESIAN_POINT ( 'NONE',  ( 15.29705854078138927, 57.37192529142944863, -30.59411708156276788 ) ) ;
#10865=DIRECTION ( 'NONE',  ( 1.000000000000000000, -0.000000000000000000, 0.000000000000000000 ) ) ;
#10866=EDGE_CURVE ( 'NONE', #9032, #11418, #12883, .T. ) ;
#10868=CARTESIAN_POINT ( 'NONE',  ( -10.14576398710722493, -69.00000000000014211, 0.5510781487875697771 ) ) ;
#10869=CARTESIAN_POINT ( 'NONE',  ( -12.99553232110414491, -17.19957910547634228, -1.530749717005650972E-15 ) ) ;
#10870=LINE ( 'NONE', #7720, #8374 ) ;
#10871=ORIENTED_EDGE ( 'NONE', *, *, #1232, .F. ) ;
#10872=CARTESIAN_POINT ( 'NONE',  ( 10.69346802281034847, 2.474956373702985601, 0.000000000000000000 ) ) ;
#10873=CARTESIAN_POINT ( 'NONE',  ( 10.69381717166375623, 72.68333662216240043, -21.38763434332750535 ) ) ;
#10875=CARTESIAN_POINT ( 'NONE',  ( 15.29705854078138927, 90.00000000000000000, 1.714422261702872766E-15 ) ) ;
#10876=CARTESIAN_POINT ( 'NONE',  ( -8.385254915620295790, -34.41905512736551032, 6.077912412602530076E-17 ) ) ;
#10877=ADVANCED_FACE ( 'NONE', ( #12737 ), #7191, .T. ) ;
#10882=CARTESIAN_POINT ( 'NONE',  ( 32.72727272727274084, 135.1423002281142089, -0.5000000000000000000 ) ) ;
#10883=CARTESIAN_POINT ( 'NONE',  ( -12.99579180576517068, 26.38439787695498495, -1.684707622963446858E-15 ) ) ;
#10886=CARTESIAN_POINT ( 'NONE',  ( 8.385254915620288685, 71.87811454074363837, 9.022884433393296612E-16 ) ) ;
#10887=EDGE_CURVE ( 'NONE', #8407, #2160, #2811, .T. ) ;
#10888=CARTESIAN_POINT ( 'NONE',  ( -15.29705854078139282, -1.063309978032473291, 1.877653204021102445E-18 ) ) ;
#10889=CARTESIAN_POINT ( 'NONE',  ( 10.00000000000000711, 139.9999999999999716, -0.5000000000000000000 ) ) ;
#10890=CARTESIAN_POINT ( 'NONE',  ( 12.99579180576517068, -30.16426982310158422, 25.99158361153035202 ) ) ;
#10892=CARTESIAN_POINT ( 'NONE',  ( 0.000000000000000000, 71.01020514433645303, 2.500000000000000000 ) ) ;
#10896=DIRECTION ( 'NONE',  ( -1.000000000000000000, 0.000000000000000000, 0.000000000000000000 ) ) ;
#10898=ORIENTED_EDGE ( 'NONE', *, *, #10557, .T. ) ;
#10899=DIRECTION ( 'NONE',  ( -2.797435172181481150E-17, 1.000000000000000000, -1.765856845898762549E-18 ) ) ;
#10900=ADVANCED_FACE ( 'NONE', ( #3183 ), #13687, .T. ) ;
#10904=CARTESIAN_POINT ( 'NONE',  ( -10.69346802281034492, 11.89973432371241380, -1.351598593231734330E-15 ) ) ;
#10905=ORIENTED_EDGE ( 'NONE', *, *, #6941, .F. ) ;
#10906=VERTEX_POINT ( 'NONE', #9641 ) ;
#10907=ORIENTED_EDGE ( 'NONE', *, *, #7724, .F. ) ;
#10908=FACE_OUTER_BOUND ( 'NONE', #2763, .T. ) ;
#10909=EDGE_LOOP ( 'NONE', ( #8053, #9177, #10247, #3689 ) ) ;
#10910=CARTESIAN_POINT ( 'NONE',  ( 12.99579180576516713, 73.50828762700209040, 3.183050967463143379E-15 ) ) ;
#10912=DIRECTION ( 'NONE',  ( -2.797435172181481150E-17, 1.000000000000000000, -1.765856845898762549E-18 ) ) ;
#10914=B_SPLINE_CURVE_WITH_KNOTS ( 'NONE', 3,
 ( #12739, #3116, #13320, #6554 ),
 .UNSPECIFIED., .F., .F.,
 ( 4, 4 ),
 ( 0.000000000000000000, 1.000000000000000000 ),
 .UNSPECIFIED. ) ;
#10918=CARTESIAN_POINT ( 'NONE',  ( -8.620861567158451422, -92.33329736102577101, 0.6435148816328051247 ) ) ;
#10921=VERTEX_POINT ( 'NONE', #10680 ) ;
#10922=EDGE_LOOP ( 'NONE', ( #10708, #12709, #7618, #8962 ) ) ;
#10923=B_SPLINE_CURVE_WITH_KNOTS ( 'NONE', 3,
 ( #11964, #2355, #274, #7908 ),
 .UNSPECIFIED., .F., .F.,
 ( 4, 4 ),
 ( 0.000000000000000000, 1.000000000000000000 ),
 .UNSPECIFIED. ) ;
#10928=( BOUNDED_SURFACE ( )  B_SPLINE_SURFACE ( 3, 3, ( 
 ( #4349, #6664, #3299, #7714 ),
 ( #4494, #1334, #3233, #7578 ),
 ( #6539, #7651, #12797, #11792 ),
 ( #5475, #11858, #13081, #11724 ) ),
 .UNSPECIFIED., .F., .F., .T. ) 
 B_SPLINE_SURFACE_WITH_KNOTS ( ( 4, 4 ),
 ( 4, 4 ),
 ( 0.000000000000000000, 1.000000000000000000 ),
 ( 0.000000000000000000, 1.000000000000000000 ),
 .UNSPECIFIED. ) 
 GEOMETRIC_REPRESENTATION_ITEM ( )  RATIONAL_B_SPLINE_SURFACE ( (
 ( 1.000000000000000000, 0.3333333333333334259, 0.3333333333333334259, 1.000000000000000000),
 ( 1.000000000000000000, 0.3333333333333334259, 0.3333333333333334259, 1.000000000000000000),
 ( 1.000000000000000000, 0.3333333333333334259, 0.3333333333333334259, 1.000000000000000000),
 ( 1.000000000000000000, 0.3333333333333334259, 0.3333333333333334259, 1.000000000000000000) ) ) 
 REPRESENTATION_ITEM ( '' )  SURFACE ( )  );
#10931=DIRECTION ( 'NONE',  ( 0.000000000000000000, 0.000000000000000000, 1.000000000000000000 ) ) ;
#10932=CARTESIAN_POINT ( 'NONE',  ( -10.69381717166375623, 34.98422482212468054, -1.433169162795722386E-15 ) ) ;
#10934=CARTESIAN_POINT ( 'NONE',  ( -0.2714810715539830999, -148.3982683978709929, -1.717521498780891109 ) ) ;
#10935=CARTESIAN_POINT ( 'NONE',  ( -15.29705854078139637, 0.8232575913728885642, -1.453755053663958216E-18 ) ) ;
#10936=DIRECTION ( 'NONE',  ( 1.000000000000000000, 0.000000000000000000, 0.000000000000000000 ) ) ;
#10937=CARTESIAN_POINT ( 'NONE',  ( -6.374260517225369682, -76.81818181818198354, -7.989319691426040926 ) ) ;
#10941=EDGE_CURVE ( 'NONE', #5403, #7000, #6377, .T. ) ;
#10942=VERTEX_POINT ( 'NONE', #11472 ) ;
#10946=CARTESIAN_POINT ( 'NONE',  ( 10.00000000000000000, 99.99999999999994316, -0.5000000000000000000 ) ) ;
#10950=ORIENTED_EDGE ( 'NONE', *, *, #13430, .T. ) ;
#10951=CARTESIAN_POINT ( 'NONE',  ( -1.673669778670227307E-15, 59.82872437272870769, -1.056489625149731375E-16 ) ) ;
#10952=ORIENTED_EDGE ( 'NONE', *, *, #5568, .T. ) ;
#10954=CIRCLE ( 'NONE', #684, 16.99999999999998934 ) ;
#10955=CIRCLE ( 'NONE', #11635, 40.00000000000001421 ) ;
#10956=DIRECTION ( 'NONE',  ( 0.000000000000000000, -1.000000000000000000, 0.000000000000000000 ) ) ;
#10957=DIRECTION ( 'NONE',  ( -1.000000000000000000, 0.000000000000000000, 0.000000000000000000 ) ) ;
#10960=CARTESIAN_POINT ( 'NONE',  ( -8.385254915620292238, -31.79444290936001138, 5.614443467303076398E-17 ) ) ;
#10961=FACE_OUTER_BOUND ( 'NONE', #7072, .T. ) ;
#10964=DIRECTION ( 'NONE',  ( -1.000000000000000000, 0.000000000000000000, 0.000000000000000000 ) ) ;
#10967=FACE_OUTER_BOUND ( 'NONE', #3547, .T. ) ;
#10968=CIRCLE ( 'NONE', #4942, 15.29705854078138749 ) ;
#10979=CARTESIAN_POINT ( 'NONE',  ( 15.29705854078139282, 64.91013567203349055, 1.757061666260241085E-15 ) ) ;
#10981=CARTESIAN_POINT ( 'NONE',  ( -15.29705854078139282, 90.00000000000000000, -1.589271161308885878E-16 ) ) ;
#10983=ORIENTED_EDGE ( 'NONE', *, *, #3161, .T. ) ;
#10984=CIRCLE ( 'NONE', #3146, 8.385254915620290461 ) ;
#10985=ORIENTED_EDGE ( 'NONE', *, *, #13589, .F. ) ;
#10990=ORIENTED_EDGE ( 'NONE', *, *, #1386, .F. ) ;
#10991=CARTESIAN_POINT ( 'NONE',  ( -12.99553232110414491, -26.62435705548577047, -1.497464099677451275E-15 ) ) ;
#10993=CARTESIAN_POINT ( 'NONE',  ( -8.385254915620292238, 34.17900274070598243, -6.035522597566817733E-17 ) ) ;
#10997=CARTESIAN_POINT ( 'NONE',  ( -5.855857762045447501, -86.34391607673575209, 7.325803626397927815 ) ) ;
#10999=ORIENTED_EDGE ( 'NONE', *, *, #4289, .F. ) ;
#11002=EDGE_CURVE ( 'NONE', #8545, #6810, #3920, .T. ) ;
#11006=EDGE_CURVE ( 'NONE', #11917, #8407, #7275, .T. ) ;
#11010=CARTESIAN_POINT ( 'NONE',  ( -8.385254915620294014, 59.82872437272870769, -2.210471567782421984E-15 ) ) ;
#11012=CARTESIAN_POINT ( 'NONE',  ( 2.054569550993968541, -122.9090909090962924, 4.917417506341301703 ) ) ;
#11013=CARTESIAN_POINT ( 'NONE',  ( -10.69381717166375623, 44.40900277213413716, -1.466454780123922280E-15 ) ) ;
#11015=CARTESIAN_POINT ( 'NONE',  ( 2.134167523386926835, -102.5454545454519746, 7.554873526039220799 ) ) ;
#11021=ORIENTED_EDGE ( 'NONE', *, *, #1041, .F. ) ;
#11023=CARTESIAN_POINT ( 'NONE',  ( 40.00000000000000711, 100.0000000000000000, 2.500000000000000000 ) ) ;
#11025=CIRCLE ( 'NONE', #4314, 8.385254915620295790 ) ;
#11026=DIRECTION ( 'NONE',  ( -2.797435172181481150E-17, 1.000000000000000000, -1.765856845898762549E-18 ) ) ;
#11027=ORIENTED_EDGE ( 'NONE', *, *, #11246, .T. ) ;
#11029=ORIENTED_EDGE ( 'NONE', *, *, #11692, .F. ) ;
#11031=EDGE_LOOP ( 'NONE', ( #1255, #13312, #12439, #5246 ) ) ;
#11032=CARTESIAN_POINT ( 'NONE',  ( 15.29705854078139282, 64.91013567203349055, 1.757061666260241085E-15 ) ) ;
#11034=CARTESIAN_POINT ( 'NONE',  ( -12.99579180576517068, 54.65873172698324112, -1.784564474948045950E-15 ) ) ;
#11037=CARTESIAN_POINT ( 'NONE',  ( -12.99579180576517423, -30.16426982310158067, -1.484993918994249462E-15 ) ) ;
#11038=DIRECTION ( 'NONE',  ( 1.000000000000000000, -1.665334536937735599E-15, 0.000000000000000000 ) ) ;
#11039=CARTESIAN_POINT ( 'NONE',  ( 8.385254915620292238, -22.36966495935058319, 1.068716529980328346E-15 ) ) ;
#11040=FACE_OUTER_BOUND ( 'NONE', #8555, .T. ) ;
#11042=CARTESIAN_POINT ( 'NONE',  ( -6.924833908958124424E-16, 24.75422479069652582, -4.371241731156832241E-17 ) ) ;
#11045=CARTESIAN_POINT ( 'NONE',  ( 4.131580040049976255, 90.90692022676346085, 2.817507346490923048 ) ) ;
#11046=VERTEX_POINT ( 'NONE', #10876 ) ;
#11048=AXIS2_PLACEMENT_3D ( 'NONE', #8507, #12526, #5213 ) ;
#11050=ADVANCED_FACE ( 'NONE', ( #6679 ), #4365, .T. ) ;
#11057=EDGE_CURVE ( 'NONE', #13719, #2222, #7661, .T. ) ;
#11058=CARTESIAN_POINT ( 'NONE',  ( -8.385254915620294014, 22.12961257269105531, -1.105053014962047635E-15 ) ) ;
#11059=CARTESIAN_POINT ( 'NONE',  ( 10.10544246783441835, -70.44230941463432316, 0.3214603529571786189 ) ) ;
#11063=AXIS2_PLACEMENT_3D ( 'NONE', #12692, #7276, #7480 ) ;
#11065=ORIENTED_EDGE ( 'NONE', *, *, #9008, .F. ) ;
#11069=CARTESIAN_POINT ( 'NONE',  ( -15.29705854078139460, -27.45107625865536605, 4.847467093863555185E-17 ) ) ;
#11070=AXIS2_PLACEMENT_3D ( 'NONE', #5293, #1094, #2198 ) ;
#11071=LINE ( 'NONE', #13361, #12043 ) ;
#11073=EDGE_CURVE ( 'NONE', #5183, #10278, #3235, .T. ) ;
#11076=CARTESIAN_POINT ( 'NONE',  ( 25.00000000000000355, 120.0000000000000284, 0.5000000000000000000 ) ) ;
#11078=CARTESIAN_POINT ( 'NONE',  ( -15.29705854078139105, 57.37192529142945574, -2.075970591910287010E-15 ) ) ;
#11080=ORIENTED_EDGE ( 'NONE', *, *, #3976, .F. ) ;
#11082=AXIS2_PLACEMENT_3D ( 'NONE', #2195, #9840, #6550 ) ;
#11084=CARTESIAN_POINT ( 'NONE',  ( 10.69346802281034314, -25.79937747632526879, 21.38693604562069694 ) ) ;
#11085=CARTESIAN_POINT ( 'NONE',  ( 4.250272934615505704, -76.81818181818026403, 9.136824450690475885 ) ) ;
#11086=ORIENTED_EDGE ( 'NONE', *, *, #10476, .T. ) ;
#11087=CARTESIAN_POINT ( 'NONE',  ( -2.517691654963332357E-15, 90.00000000000000000, -1.589271161308885878E-16 ) ) ;
#11090=CARTESIAN_POINT ( 'NONE',  ( 0.1852016367018599896, -70.00000000000000000, -1.488522876466113809 ) ) ;
#11092=CARTESIAN_POINT ( 'NONE',  ( 5.655105406253481348, -85.78354978357639027, -8.815184813446974132 ) ) ;
#11095=CARTESIAN_POINT ( 'NONE',  ( -2.517691654963332357E-15, 90.00000000000000000, -1.589271161308885878E-16 ) ) ;
#11098=DIRECTION ( 'NONE',  ( 0.000000000000000000, 0.000000000000000000, 1.000000000000000000 ) ) ;
#11100=ORIENTED_EDGE ( 'NONE', *, *, #13462, .F. ) ;
#11102=ORIENTED_EDGE ( 'NONE', *, *, #11246, .F. ) ;
#11104=ORIENTED_EDGE ( 'NONE', *, *, #9011, .F. ) ;
#11105=CARTESIAN_POINT ( 'NONE',  ( -3.377085873584029674, -129.6408637431290458, 2.289279048948418716 ) ) ;
#11108=VECTOR ( 'NONE', #582, 1000.000000000000000 ) ;
#11109=LINE ( 'NONE', #13315, #805 ) ;
#11110=CARTESIAN_POINT ( 'NONE',  ( 2.179449471770333435, 90.00000000000000000, -4.500000000000000888 ) ) ;
#11111=ORIENTED_EDGE ( 'NONE', *, *, #9297, .F. ) ;
#11112=ORIENTED_EDGE ( 'NONE', *, *, #10054, .T. ) ;
#11113=DIRECTION ( 'NONE',  ( -2.797435172181481150E-17, 1.000000000000000000, -1.765856845898762549E-18 ) ) ;
#11114=ORIENTED_EDGE ( 'NONE', *, *, #13865, .T. ) ;
#11116=CARTESIAN_POINT ( 'NONE',  ( -31.81818181818181657, 133.3608531424536920, -0.5000000000000000000 ) ) ;
#11119=DIRECTION ( 'NONE',  ( 2.797435172181480534E-17, -1.000000000000000000, 1.765856845898762164E-18 ) ) ;
#11120=CARTESIAN_POINT ( 'NONE',  ( -2.008006351130390499, -80.00378950643924725, -9.910921267331605833 ) ) ;
#11123=DIRECTION ( 'NONE',  ( -2.797435172181481150E-17, 1.000000000000000000, -1.765856845898762549E-18 ) ) ;
#11124=B_SPLINE_CURVE_WITH_KNOTS ( 'NONE', 3,
 ( #7178, #5080, #12451, #11662, #1080, #3371, #5540, #13085, #12802, #3169 ),
 .UNSPECIFIED., .F., .F.,
 ( 4, 3, 3, 4 ),
 ( 0.000000000000000000, 0.0006882994548164135529, 0.001843858713197575735, 0.002999417971958379548 ),
 .UNSPECIFIED. ) ;
#11125=CARTESIAN_POINT ( 'NONE',  ( -10.69346802281034314, -6.949821576306441706, -21.38693604562069694 ) ) ;
#11126=CARTESIAN_POINT ( 'NONE',  ( -10.69381717166375267, 53.83378072214353693, -21.38763434332751245 ) ) ;
#11127=ORIENTED_EDGE ( 'NONE', *, *, #5654, .F. ) ;
#11128=CARTESIAN_POINT ( 'NONE',  ( 56.97938482224745371, -167.3636363686644870, 8.923382219704807383 ) ) ;
#11134=CARTESIAN_POINT ( 'NONE',  ( -10.69381717166375090, 34.98422482212468054, -21.38763434332750890 ) ) ;
#11135=CARTESIAN_POINT ( 'NONE',  ( 8.207015671355002297E-16, -29.33764382806072746, 5.180607919632063331E-17 ) ) ;
#11136=FACE_OUTER_BOUND ( 'NONE', #8916, .T. ) ;
#11138=CARTESIAN_POINT ( 'NONE',  ( 15.29705854078138749, -38.76242177807012723, 30.59411708156277854 ) ) ;
#11140=B_SPLINE_SURFACE_WITH_KNOTS ( 'NONE', 3, 3, ( 
 ( #6911, #11128, #5880, #8114, #7052, #5797, #11198, #8178, #10150, #3758, #4954, #12463, #10217, #13412, #2715, #9096, #555, #12179, #6991, #11331, #6012, #13484, #10353, #13338 ),
 ( #6849, #8042, #3830, #10281, #1515, #3687, #4820, #10076, #488, #13549, #9236, #2642, #2846, #12323, #5944, #683, #9027, #621, #7973, #12254, #4881, #12397, #11395, #753 ),
 ( #5019, #3969, #9442, #12605, #7254, #13880, #6345, #7387, #9301, #7320, #13750, #10612, #1933, #8378, #10417, #2916, #10481, #1998, #2125, #6150, #6220, #11469, #1020, #4227 ),
 ( #3112, #7456, #13620, #954, #6278, #4096, #13683, #2982, #8242, #10550, #9371, #883, #5151, #5216, #9503, #9569, #13813, #4163, #8447, #12734, #5288, #12815, #11737, #12534 ) ),
 .UNSPECIFIED., .F., .F., .F.,
 ( 4, 4 ),
 ( 4, 1, 1, 1, 1, 1, 1, 1, 1, 1, 1, 1, 1, 1, 1, 1, 1, 1, 1, 1, 1, 4 ),
 ( -0.02200000000000000566, 0.002000000000000001776 ),
 ( -0.009000000000000030545, -0.004090909090909119854, -2.775557561562891043E-17, 0.0008181818181817908375, 0.005727272727272700661, 0.01250649350649347610, 0.02045454545454543360, 0.02536363636363634516, 0.03027272727272725672, 0.03518181818181816828, 0.04009090909090907984, 0.04990909090909089602, 0.05481818181818180757, 0.05972727272727271913, 0.06463636363636363069, 0.06954545454545453531, 0.07749350649350648934, 0.08427272727272726305, 0.08918181818181818155, 0.08999999999999998279, 0.09409090909090908617, 0.09900000000000000466 ),
 .UNSPECIFIED. ) ;
#11143=EDGE_CURVE ( 'NONE', #6441, #11311, #9272, .T. ) ;
#11144=CARTESIAN_POINT ( 'NONE',  ( 2.008006476061143353, -80.00378950643523979, 9.910921260988354575 ) ) ;
#11146=VERTEX_POINT ( 'NONE', #10946 ) ;
#11149=CARTESIAN_POINT ( 'NONE',  ( -25.00000000000000355, 120.0000000000000284, 2.500000000000000000 ) ) ;
#11151=CARTESIAN_POINT ( 'NONE',  ( 8.385254915620299343, -34.41905512736551032, 1.085359338644428786E-15 ) ) ;
#11152=CARTESIAN_POINT ( 'NONE',  ( 8.592794974440716160, -91.93698159008127391, -1.116928117929663955 ) ) ;
#11153=CARTESIAN_POINT ( 'NONE',  ( -15.29705854078139282, 57.37192529142944863, 30.59411708156276788 ) ) ;
#11157=ADVANCED_FACE ( 'NONE', ( #5004 ), #7069, .T. ) ;
#11161=CARTESIAN_POINT ( 'NONE',  ( 5.783440176334763372, -75.54545454545555572, 8.231660884606897710 ) ) ;
#11163=CARTESIAN_POINT ( 'NONE',  ( 39.99999999999999289, 120.0000000000000284, -0.5000000000000000000 ) ) ;
#11165=CARTESIAN_POINT ( 'NONE',  ( 15.29705854078139105, -10.48808792804187284, 1.890204135573039875E-15 ) ) ;
#11166=DIRECTION ( 'NONE',  ( 0.9923485843107423543, 2.797833471351478217E-17, 0.1234677578012386562 ) ) ;
#11167=CARTESIAN_POINT ( 'NONE',  ( -3.371721678969553881, -122.9090909090926260, -4.477688567679849463 ) ) ;
#11171=ORIENTED_EDGE ( 'NONE', *, *, #11598, .F. ) ;
#11172=ORIENTED_EDGE ( 'NONE', *, *, #3264, .T. ) ;
#11173=CIRCLE ( 'NONE', #2660, 8.385254915620294014 ) ;
#11176=CARTESIAN_POINT ( 'NONE',  ( 1.738256873884670206, -152.7600787142097261, 0.2641564897029298753 ) ) ;
#11179=CARTESIAN_POINT ( 'NONE',  ( 5.458723002619491282, -108.0793881314434088, -3.832583767769556005 ) ) ;
#11181=DIRECTION ( 'NONE',  ( -2.797435172181481150E-17, 1.000000000000000000, -1.765856845898762549E-18 ) ) ;
#11183=ORIENTED_EDGE ( 'NONE', *, *, #11057, .F. ) ;
#11186=ORIENTED_EDGE ( 'NONE', *, *, #9175, .F. ) ;
#11187=CARTESIAN_POINT ( 'NONE',  ( -1.786297911977085207, -149.6807761101056826, 0.8805805580279005840 ) ) ;
#11188=VECTOR ( 'NONE', #10404, 1000.000000000000000 ) ;
#11189=DIRECTION ( 'NONE',  ( -1.000000000000000000, 0.000000000000000000, 0.000000000000000000 ) ) ;
#11194=CARTESIAN_POINT ( 'NONE',  ( 10.69381717166375445, 16.13466892210585613, 2.619229793989003951E-15 ) ) ;
#11196=CARTESIAN_POINT ( 'NONE',  ( 4.318061424038318385, 91.66495677434029687, 2.521242278247964208 ) ) ;
#11197=VERTEX_POINT ( 'NONE', #4729 ) ;
#11198=CARTESIAN_POINT ( 'NONE',  ( 0.2321914886046761162, -147.1038961038780997, -14.56966866480831335 ) ) ;
#11203=CARTESIAN_POINT ( 'NONE',  ( -54.35437857574594744, -62.63636364547547686, -19.28415345477669973 ) ) ;
#11205=TOROIDAL_SURFACE ( 'NONE', #7837, 16.99999999999998934, 2.000000000000000000 ) ;
#11207=CARTESIAN_POINT ( 'NONE',  ( 15.29705854078140170, -19.91286587805129926, 3.746698755667524778E-15 ) ) ;
#11208=CIRCLE ( 'NONE', #4464, 2.000000000000000000 ) ;
#11209=CARTESIAN_POINT ( 'NONE',  ( -12.99553232110414136, -36.04913500549519512, -1.464178482349251183E-15 ) ) ;
#11215=CIRCLE ( 'NONE', #12344, 24.99999999999998934 ) ;
#11216=VECTOR ( 'NONE', #9914, 1000.000000000000000 ) ;
#11217=FACE_OUTER_BOUND ( 'NONE', #6499, .T. ) ;
#11219=CARTESIAN_POINT ( 'NONE',  ( -12.99553232110413425, -36.04913500549519512, -25.99106464220827917 ) ) ;
#11220=CARTESIAN_POINT ( 'NONE',  ( -8.385254915620299343, 78.67828027274755698, -1.304766718931246017E-15 ) ) ;
#11222=CYLINDRICAL_SURFACE ( 'NONE', #9102, 15.29705854078139105 ) ;
#11223=CARTESIAN_POINT ( 'NONE',  ( 8.591959856086345937, -92.28134618798193856, -0.7058139155579893353 ) ) ;
#11225=CARTESIAN_POINT ( 'NONE',  ( 8.385254915620294014, 50.40394642271930792, 9.813990265092209853E-16 ) ) ;
#11228=AXIS2_PLACEMENT_3D ( 'NONE', #11375, #9004, #13391 ) ;
#11232=CARTESIAN_POINT ( 'NONE',  ( -2.504065471750553911E-13, 90.00000000000000000, 4.500000000000000888 ) ) ;
#11233=DIRECTION ( 'NONE',  ( -2.797435172181481150E-17, 1.000000000000000000, -1.765856845898762549E-18 ) ) ;
#11240=DIRECTION ( 'NONE',  ( -1.000000000000000000, 0.000000000000000000, 0.000000000000000000 ) ) ;
#11241=CARTESIAN_POINT ( 'NONE',  ( 5.245880486154336886, -97.41991341991632680, 6.871249260556994365 ) ) ;
#11242=CARTESIAN_POINT ( 'NONE',  ( -15.29705854078138749, -36.87585420866476227, 6.511747960273540061E-17 ) ) ;
#11243=CARTESIAN_POINT ( 'NONE',  ( 25.00000000000000355, 120.0000000000000284, 2.500000000000000000 ) ) ;
#11245=DIRECTION ( 'NONE',  ( -2.797435172181481150E-17, 1.000000000000000000, -1.765856845898762549E-18 ) ) ;
#11246=EDGE_CURVE ( 'NONE', #3535, #1501, #2589, .T. ) ;
#11249=ORIENTED_EDGE ( 'NONE', *, *, #2082, .T. ) ;
#11250=CARTESIAN_POINT ( 'NONE',  ( 0.6788169696763596273, -157.4020095821269649, 1.357710655470797834 ) ) ;
#11252=CARTESIAN_POINT ( 'NONE',  ( 5.164320697881710664, -107.4929201522786002, -4.328224869514438744 ) ) ;
#11253=CARTESIAN_POINT ( 'NONE',  ( -25.00000000000000355, 120.0000000000000284, 2.500000000000000000 ) ) ;
#11256=FACE_OUTER_BOUND ( 'NONE', #4387, .T. ) ;
#11259=CARTESIAN_POINT ( 'NONE',  ( 3.655937883597065952, -133.4173050103803746, -0.08043032631485191875 ) ) ;
#11264=CARTESIAN_POINT ( 'NONE',  ( -10.00000000000000711, 97.99999999999994316, -0.5000000000000000000 ) ) ;
#11267=EDGE_LOOP ( 'NONE', ( #10570, #1847, #9919, #4382 ) ) ;
#11268=ORIENTED_EDGE ( 'NONE', *, *, #5573, .T. ) ;
#11269=ORIENTED_EDGE ( 'NONE', *, *, #10136, .T. ) ;
#11270=VERTEX_POINT ( 'NONE', #11317 ) ;
#11273=EDGE_CURVE ( 'NONE', #717, #8407, #9220, .T. ) ;
#11274=CARTESIAN_POINT ( 'NONE',  ( 12.99579180576517068, 35.80917582696438473, -25.99158361153033070 ) ) ;
#11275=B_SPLINE_CURVE_WITH_KNOTS ( 'NONE', 3,
 ( #11355, #1817, #12632, #3006 ),
 .UNSPECIFIED., .F., .F.,
 ( 4, 4 ),
 ( 0.000000000000000000, 1.000000000000000000 ),
 .UNSPECIFIED. ) ;
#11278=EDGE_CURVE ( 'NONE', #6854, #4529, #12238, .T. ) ;
#11279=CARTESIAN_POINT ( 'NONE',  ( 12.99553232110414314, -36.04913500549519512, 3.182987412051232168E-15 ) ) ;
#11280=CARTESIAN_POINT ( 'NONE',  ( 8.557187120185842488, -74.11437726413154792, 5.386762667206737021 ) ) ;
#11285=FACE_OUTER_BOUND ( 'NONE', #417, .T. ) ;
#11286=ORIENTED_EDGE ( 'NONE', *, *, #3264, .F. ) ;
#11287=CARTESIAN_POINT ( 'NONE',  ( 10.69346802281034137, 77.87317997377837742, 21.38693604562069694 ) ) ;
#11288=CARTESIAN_POINT ( 'NONE',  ( -9.567184146940780565, -70.42919439405125104, -3.281027101740300989 ) ) ;
#11290=CARTESIAN_POINT ( 'NONE',  ( 8.530666014548659248, -92.96565381893854862, 0.1002375751519047481 ) ) ;
#11291=CARTESIAN_POINT ( 'NONE',  ( 8.385254915620292238, 15.32944684068712782, 1.008767855514154504E-15 ) ) ;
#11293=ORIENTED_EDGE ( 'NONE', *, *, #1654, .F. ) ;
#11294=ORIENTED_EDGE ( 'NONE', *, *, #3718, .T. ) ;
#11295=EDGE_CURVE ( 'NONE', #8596, #13265, #11109, .T. ) ;
#11296=ORIENTED_EDGE ( 'NONE', *, *, #2009, .F. ) ;
#11298=CARTESIAN_POINT ( 'NONE',  ( 3.385241169372599668, -79.21212121212093393, 9.605957155564981420 ) ) ;
#11299=ORIENTED_EDGE ( 'NONE', *, *, #12213, .T. ) ;
#11300=DIRECTION ( 'NONE',  ( -2.797435172181481150E-17, 1.000000000000000000, -1.765856845898762549E-18 ) ) ;
#11301=CARTESIAN_POINT ( 'NONE',  ( 0.5797347049570226174, -122.9090909090902528, -5.796875383663783410 ) ) ;
#11304=( NAMED_UNIT ( * ) PLANE_ANGLE_UNIT ( ) SI_UNIT ( $, .RADIAN. ) );
#11305=AXIS2_PLACEMENT_3D ( 'NONE', #7057, #561, #13555 ) ;
#11311=VERTEX_POINT ( 'NONE', #2626 ) ;
#11312=EDGE_CURVE ( 'NONE', #12645, #4658, #10429, .T. ) ;
#11313=CARTESIAN_POINT ( 'NONE',  ( -3.735183152658258177, -131.9664157448443973, 0.9167613680711519386 ) ) ;
#11317=CARTESIAN_POINT ( 'NONE',  ( -4.547999443521272056, -70.00000000000000000, -2.077426547854386296 ) ) ;
#11321=DIRECTION ( 'NONE',  ( 0.000000000000000000, 0.000000000000000000, 1.000000000000000000 ) ) ;
#11323=CARTESIAN_POINT ( 'NONE',  ( 4.866961404864791341, 90.10495303670558087, -1.152376359967959507 ) ) ;
#11324=DIRECTION ( 'NONE',  ( -1.000000000000000000, 0.000000000000000000, 0.000000000000000000 ) ) ;
#11326=DIRECTION ( 'NONE',  ( -1.000000000000000000, 0.000000000000000000, 0.000000000000000000 ) ) ;
#11327=CARTESIAN_POINT ( 'NONE',  ( 8.385254915620285132, 62.45333659073424570, 16.77050983124058092 ) ) ;
#11329=ORIENTED_EDGE ( 'NONE', *, *, #10941, .T. ) ;
#11331=CARTESIAN_POINT ( 'NONE',  ( 10.12341346682585552, -72.18181818173118813, 6.554034102529832317 ) ) ;
#11336=CARTESIAN_POINT ( 'NONE',  ( -4.942677383991351370, 90.01345119373434045, -0.7661926690451024147 ) ) ;
#11337=EDGE_CURVE ( 'NONE', #3017, #9032, #8189, .T. ) ;
#11339=AXIS2_PLACEMENT_3D ( 'NONE', #1261, #5526, #8483 ) ;
#11340=CARTESIAN_POINT ( 'NONE',  ( 3.794964386185876837, -129.7272727272737995, -2.624161884219710750 ) ) ;
#11341=CARTESIAN_POINT ( 'NONE',  ( -10.69381717166375623, 6.709890972096426154, -1.333312310811123490E-15 ) ) ;
#11342=CARTESIAN_POINT ( 'NONE',  ( -15.29705854078139637, 90.00000000000000000, -1.589271161308885878E-16 ) ) ;
#11343=CARTESIAN_POINT ( 'NONE',  ( 10.69346802281034314, 21.32451227372186864, 2.619144277183852766E-15 ) ) ;
#11344=CARTESIAN_POINT ( 'NONE',  ( 10.00000000000000000, 92.00000000000000000, -0.5000000000000000000 ) ) ;
#11345=CIRCLE ( 'NONE', #3065, 22.99999999999999645 ) ;
#11347=ADVANCED_FACE ( 'NONE', ( #8018 ), #10120, .T. ) ;
#11349=EDGE_CURVE ( 'NONE', #11270, #9083, #7968, .T. ) ;
#11350=ORIENTED_EDGE ( 'NONE', *, *, #2599, .F. ) ;
#11352=CARTESIAN_POINT ( 'NONE',  ( -15.29705854078138749, -10.48808792804187284, -30.59411708156277854 ) ) ;
#11354=CARTESIAN_POINT ( 'NONE',  ( -10.69346802281034847, -6.949821576306442594, -1.285027358575335329E-15 ) ) ;
#11355=CARTESIAN_POINT ( 'NONE',  ( -8.385254915620294014, 59.82872437272870769, -1.056489625149731375E-16 ) ) ;
#11356=CARTESIAN_POINT ( 'NONE',  ( -10.00000000000000000, 99.99999999999994316, -0.5000000000000000000 ) ) ;
#11357=CARTESIAN_POINT ( 'NONE',  ( -5.081042958706433410, -118.5729905622867193, -1.793999374523247203 ) ) ;
#11358=CARTESIAN_POINT ( 'NONE',  ( -8.385254915620294014, 59.82872437272870769, -1.238195484274846031E-15 ) ) ;
#11359=VERTEX_POINT ( 'NONE', #7942 ) ;
#11363=CARTESIAN_POINT ( 'NONE',  ( -8.385254915620292238, -12.94488700934118341, 2.285881734483108495E-17 ) ) ;
#11364=CARTESIAN_POINT ( 'NONE',  ( 10.17548876272776859, -70.78787878787939292, 0.6371443735352817495 ) ) ;
#11367=CARTESIAN_POINT ( 'NONE',  ( 10.69381717166374912, 44.40900277213413716, 21.38763434332751245 ) ) ;
#11368=DIRECTION ( 'NONE',  ( -2.797435172181481150E-17, 1.000000000000000000, -1.765856845898762549E-18 ) ) ;
#11369=DIRECTION ( 'NONE',  ( -2.797435172181481150E-17, 1.000000000000000000, -1.765856845898762549E-18 ) ) ;
#11371=CARTESIAN_POINT ( 'NONE',  ( 0.1741500050819346779, -159.7355659919405184, -1.510064380825568708 ) ) ;
#11375=CARTESIAN_POINT ( 'NONE',  ( -35.20000000000000995, 106.4000000000000199, 0.5000000000000000000 ) ) ;
#11377=( BOUNDED_SURFACE ( )  B_SPLINE_SURFACE ( 3, 3, ( 
 ( #11220, #8060, #8131, #13433 ),
 ( #6874, #3782, #11287, #9182 ),
 ( #13208, #13506, #13283, #1533 ),
 ( #4771, #7076, #7844, #12132 ) ),
 .UNSPECIFIED., .F., .F., .T. ) 
 B_SPLINE_SURFACE_WITH_KNOTS ( ( 4, 4 ),
 ( 4, 4 ),
 ( 0.000000000000000000, 1.000000000000000000 ),
 ( 0.000000000000000000, 1.000000000000000000 ),
 .UNSPECIFIED. ) 
 GEOMETRIC_REPRESENTATION_ITEM ( )  RATIONAL_B_SPLINE_SURFACE ( (
 ( 1.000000000000000000, 0.3333333333333334259, 0.3333333333333334259, 1.000000000000000000),
 ( 1.000000000000000000, 0.3333333333333334259, 0.3333333333333334259, 1.000000000000000000),
 ( 1.000000000000000000, 0.3333333333333334259, 0.3333333333333334259, 1.000000000000000000),
 ( 1.000000000000000000, 0.3333333333333334259, 0.3333333333333334259, 1.000000000000000000) ) ) 
 REPRESENTATION_ITEM ( '' )  SURFACE ( )  );
#11378=CARTESIAN_POINT ( 'NONE',  ( 2.952295391231332111, -104.4213889740930199, -6.466433248859399185 ) ) ;
#11382=DIRECTION ( 'NONE',  ( -1.000000000000000000, 0.000000000000000000, 0.000000000000000000 ) ) ;
#11386=CARTESIAN_POINT ( 'NONE',  ( 8.385254915620295790, 3.280056672672171381, -16.77050983124058448 ) ) ;
#11393=VERTEX_POINT ( 'NONE', #6955 ) ;
#11394=CARTESIAN_POINT ( 'NONE',  ( 8.385254915620294014, 3.280056672672199358, 1.018788103988028997E-15 ) ) ;
#11395=CARTESIAN_POINT ( 'NONE',  ( 17.09331748281897490, -62.63636361073249503, 11.08568378623573558 ) ) ;
#11396=VERTEX_POINT ( 'NONE', #11242 ) ;
#11397=CIRCLE ( 'NONE', #3544, 2.000000000000003109 ) ;
#11398=ORIENTED_EDGE ( 'NONE', *, *, #12123, .T. ) ;
#11400=CARTESIAN_POINT ( 'NONE',  ( 8.385254915620294014, 90.00000000000000000, 8.679704431140118580E-16 ) ) ;
#11401=B_SPLINE_CURVE_WITH_KNOTS ( 'NONE', 3,
 ( #5889, #3768, #3545, #4893, #3624, #1383, #9942, #12339, #8051, #12192, #5662, #2726, #11280, #1674, #4610, #12040, #7833, #12119, #502, #2511, #6786, #11059, #10228, #1452 ),
 .UNSPECIFIED., .F., .F.,
 ( 4, 2, 2, 2, 2, 2, 2, 2, 2, 2, 2, 4 ),
 ( 0.000000000000000000, 0.002159622240606462202, 0.003239433360909706097, 0.004319244481212950425, 0.006478866721819439949, 0.008638488962425930340, 0.01079811120303241813, 0.01295773344363890592, 0.01403754456394215068, 0.01511735568424539371, 0.01619716680454863847, 0.01727697792485188150 ),
 .UNSPECIFIED. ) ;
#11402=( BOUNDED_SURFACE ( )  B_SPLINE_SURFACE ( 3, 3, ( 
 ( #7649, #383, #6596, #11010 ),
 ( #3496, #4636, #6538, #6739 ),
 ( #1410, #2252, #8919, #1209 ),
 ( #8770, #10863, #5688, #3572 ) ),
 .UNSPECIFIED., .F., .F., .T. ) 
 B_SPLINE_SURFACE_WITH_KNOTS ( ( 4, 4 ),
 ( 4, 4 ),
 ( 0.000000000000000000, 1.000000000000000000 ),
 ( 0.000000000000000000, 1.000000000000000000 ),
 .UNSPECIFIED. ) 
 GEOMETRIC_REPRESENTATION_ITEM ( )  RATIONAL_B_SPLINE_SURFACE ( (
 ( 1.000000000000000000, 0.3333333333333334259, 0.3333333333333334259, 1.000000000000000000),
 ( 1.000000000000000000, 0.3333333333333334259, 0.3333333333333334259, 1.000000000000000000),
 ( 1.000000000000000000, 0.3333333333333334259, 0.3333333333333334259, 1.000000000000000000),
 ( 1.000000000000000000, 0.3333333333333334259, 0.3333333333333334259, 1.000000000000000000) ) ) 
 REPRESENTATION_ITEM ( '' )  SURFACE ( )  );
#11403=CARTESIAN_POINT ( 'NONE',  ( -12.97432671026129292, -68.90909090921795155, -1.142286363974290175 ) ) ;
#11404=EDGE_CURVE ( 'NONE', #1745, #8317, #5694, .T. ) ;
#11405=DIRECTION ( 'NONE',  ( 0.000000000000000000, 0.000000000000000000, 1.000000000000000000 ) ) ;
#11406=DIRECTION ( 'NONE',  ( -2.797435172181481150E-17, 1.000000000000000000, -1.765856845898762549E-18 ) ) ;
#11408=CARTESIAN_POINT ( 'NONE',  ( 12.99579180576517601, -30.16426982310158067, 0.000000000000000000 ) ) ;
#11409=AXIS2_PLACEMENT_3D ( 'NONE', #12931, #4486, #9621 ) ;
#11410=CARTESIAN_POINT ( 'NONE',  ( -4.390129302555909163, 91.34360472797649777, 2.393760519723236779 ) ) ;
#11415=VERTEX_POINT ( 'NONE', #13385 ) ;
#11418=VERTEX_POINT ( 'NONE', #4565 ) ;
#11419=CARTESIAN_POINT ( 'NONE',  ( 10.69381717166375978, -12.13966492792242846, -21.38763434332751245 ) ) ;
#11424=CARTESIAN_POINT ( 'NONE',  ( -2.517691654963332357E-15, 90.00000000000000000, -1.589271161308885878E-16 ) ) ;
#11425=CARTESIAN_POINT ( 'NONE',  ( 5.863164109270496915, -98.21466495864295609, 5.258484191817180076 ) ) ;
#11426=CARTESIAN_POINT ( 'NONE',  ( -12.99553232110414314, 48.77386654458962312, -3.284728769657734804E-15 ) ) ;
#11428=ADVANCED_FACE ( 'NONE', ( #3579 ), #3734, .T. ) ;
#11433=CIRCLE ( 'NONE', #4482, 15.29705854078139105 ) ;
#11434=AXIS2_PLACEMENT_3D ( 'NONE', #3669, #5928, #542 ) ;
#11436=CARTESIAN_POINT ( 'NONE',  ( -4.131580040049980695, 90.90692022676346085, -2.817507346490921716 ) ) ;
#11439=VERTEX_POINT ( 'NONE', #13154 ) ;
#11440=DIRECTION ( 'NONE',  ( -0.000000000000000000, -0.000000000000000000, -1.000000000000000000 ) ) ;
#11441=B_SPLINE_CURVE_WITH_KNOTS ( 'NONE', 3,
 ( #8760, #4479, #20, #4405 ),
 .UNSPECIFIED., .F., .F.,
 ( 4, 4 ),
 ( 0.000000000000000000, 1.000000000000000000 ),
 .UNSPECIFIED. ) ;
#11442=CIRCLE ( 'NONE', #12792, 2.000000000000000000 ) ;
#11443=CARTESIAN_POINT ( 'NONE',  ( 8.385254915620290461, 43.60378069071538221, 2.053795118489799215E-15 ) ) ;
#11447=CARTESIAN_POINT ( 'NONE',  ( -2.625033373859935182, -142.3538918234897608, -0.5598298894019758665 ) ) ;
#11457=CARTESIAN_POINT ( 'NONE',  ( -4.330127018922195425, 92.00000000000000000, 2.500000000000000000 ) ) ;
#11458=CARTESIAN_POINT ( 'NONE',  ( -1.344244725514634808, -147.1541672456599485, 1.755023797081159298 ) ) ;
#11459=CARTESIAN_POINT ( 'NONE',  ( -1.713057075430773901, -163.8787878553926589, -2.641018403485157595 ) ) ;
#11460=CARTESIAN_POINT ( 'NONE',  ( -8.385254915620295790, 40.97916847270985130, -7.236334518677345233E-17 ) ) ;
#11462=DIRECTION ( 'NONE',  ( -1.000000000000000000, 0.000000000000000000, 0.000000000000000000 ) ) ;
#11463=CARTESIAN_POINT ( 'NONE',  ( -10.00000000000000000, 90.00000000000000000, -0.5000000000000000000 ) ) ;
#11464=CARTESIAN_POINT ( 'NONE',  ( 12.99553232110414136, 29.92431064457076673, 3.182987412051232168E-15 ) ) ;
#11466=DIRECTION ( 'NONE',  ( -2.797435172181481150E-17, 1.000000000000000000, -1.765856845898762549E-18 ) ) ;
#11467=ORIENTED_EDGE ( 'NONE', *, *, #10547, .F. ) ;
#11469=CARTESIAN_POINT ( 'NONE',  ( 2.247751904495991049, -65.63636362675833880, -0.1634371280250800362 ) ) ;
#11472=CARTESIAN_POINT ( 'NONE',  ( 8.385254915620292238, 22.12961257269105531, 9.855024866598291022E-16 ) ) ;
#11478=CARTESIAN_POINT ( 'NONE',  ( -2.940534136605371440, -72.18181818208977063, -3.082537950463050791 ) ) ;
#11480=CARTESIAN_POINT ( 'NONE',  ( 15.29705854078138927, 47.94714734142005597, 3.746698755667522411E-15 ) ) ;
#11481=DIRECTION ( 'NONE',  ( -2.797435172181481150E-17, 1.000000000000000000, -1.765856845898762549E-18 ) ) ;
#11482=CARTESIAN_POINT ( 'NONE',  ( -4.330127018922195425, 91.86461561432780343, 2.500000000000000000 ) ) ;
#11485=CARTESIAN_POINT ( 'NONE',  ( 25.00000000000000355, 120.0000000000000284, 0.5000000000000000000 ) ) ;
#11486=ADVANCED_FACE ( 'NONE', ( #13656 ), #2821, .T. ) ;
#11487=( BOUNDED_SURFACE ( )  B_SPLINE_SURFACE ( 3, 3, ( 
 ( #7887, #549, #3171, #10606 ),
 ( #9362, #10410, #6210, #11727 ),
 ( #8439, #6335, #8234, #13807 ),
 ( #13608, #7376, #11530, #5279 ) ),
 .UNSPECIFIED., .F., .F., .F. ) 
 B_SPLINE_SURFACE_WITH_KNOTS ( ( 4, 4 ),
 ( 4, 4 ),
 ( 0.000000000000000000, 1.000000000000000000 ),
 ( 0.000000000000000000, 1.000000000000000000 ),
 .UNSPECIFIED. ) 
 GEOMETRIC_REPRESENTATION_ITEM ( )  RATIONAL_B_SPLINE_SURFACE ( (
 ( 1.000000000000000000, 0.3333333333333334259, 0.3333333333333334259, 1.000000000000000000),
 ( 1.000000000000000000, 0.3333333333333334259, 0.3333333333333334259, 1.000000000000000000),
 ( 1.000000000000000000, 0.3333333333333334259, 0.3333333333333334259, 1.000000000000000000),
 ( 1.000000000000000000, 0.3333333333333334259, 0.3333333333333334259, 1.000000000000000000) ) ) 
 REPRESENTATION_ITEM ( '' )  SURFACE ( )  );
#11488=AXIS2_PLACEMENT_3D ( 'NONE', #13045, #1382, #5661 ) ;
#11489=EDGE_CURVE ( 'NONE', #10942, #1315, #8409, .T. ) ;
#11495=CIRCLE ( 'NONE', #11063, 40.00000000000001421 ) ;
#11496=CARTESIAN_POINT ( 'NONE',  ( 2.034007080467508111, -145.4043805342818985, 1.227505828596866744 ) ) ;
#11497=VECTOR ( 'NONE', #7295, 1000.000000000000000 ) ;
#11499=VERTEX_POINT ( 'NONE', #7231 ) ;
#11501=ORIENTED_EDGE ( 'NONE', *, *, #9886, .T. ) ;
#11516=CARTESIAN_POINT ( 'NONE',  ( 5.783304142548281845, -114.8445492426030938, -0.9050494705503316917 ) ) ;
#11519=VERTEX_POINT ( 'NONE', #5065 ) ;
#11520=ORIENTED_EDGE ( 'NONE', *, *, #6079, .F. ) ;
#11522=CARTESIAN_POINT ( 'NONE',  ( -2.531075078303758552, -137.7090071379864753, -1.916367648672105295 ) ) ;
#11524=CARTESIAN_POINT ( 'NONE',  ( -8.385254915620295790, 40.97916847270985130, -2.162146219129312653E-15 ) ) ;
#11525=CARTESIAN_POINT ( 'NONE',  ( 4.319514923984686838, -82.51052574872602463, -8.744483155999079216 ) ) ;
#11527=CARTESIAN_POINT ( 'NONE',  ( 0.1425268984561593455, -158.0606060592834297, -0.6718241418694251843 ) ) ;
#11528=CARTESIAN_POINT ( 'NONE',  ( 9.987599105592503079, -70.00000000000073896, 0.7388069301397282018 ) ) ;
#11529=CIRCLE ( 'NONE', #13806, 22.99999999999999289 ) ;
#11530=CARTESIAN_POINT ( 'NONE',  ( -15.29705854078138394, 19.67281349139177138, -30.59411708156277854 ) ) ;
#11531=FACE_OUTER_BOUND ( 'NONE', #9331, .T. ) ;
#11533=TOROIDAL_SURFACE ( 'NONE', #6173, 77.99999999999997158, 2.000000000000000000 ) ;
#11534=DIRECTION ( 'NONE',  ( -1.000000000000000000, 0.000000000000000000, 0.000000000000000000 ) ) ;
#11535=LINE ( 'NONE', #2978, #8120 ) ;
#11539=AXIS2_PLACEMENT_3D ( 'NONE', #49, #4303, #9445 ) ;
#11541=CARTESIAN_POINT ( 'NONE',  ( 8.385254915620292238, 90.00000000000000000, 8.679704431140114636E-16 ) ) ;
#11546=CARTESIAN_POINT ( 'NONE',  ( -3.036220672062509340, -100.2727272727325953, -3.474096187147796222 ) ) ;
#11548=CARTESIAN_POINT ( 'NONE',  ( -8.385254915620297567, 50.40394642271930792, -1.204909866946646925E-15 ) ) ;
#11550=CARTESIAN_POINT ( 'NONE',  ( 1.958204620527036102E-15, -69.99999999999998579, 1.236099792129133461E-16 ) ) ;
#11552=( GEOMETRIC_REPRESENTATION_CONTEXT ( 3 ) GLOBAL_UNCERTAINTY_ASSIGNED_CONTEXT ( ( #4892 ) ) GLOBAL_UNIT_ASSIGNED_CONTEXT ( ( #2535, #6738, #4558 ) ) REPRESENTATION_CONTEXT ( 'NONE', 'WORKASPACE' ) );
#11555=CARTESIAN_POINT ( 'NONE',  ( -8.873256490562051013, -89.39237735558731401, 1.261745358756553470 ) ) ;
#11559=CARTESIAN_POINT ( 'NONE',  ( -8.385254915620294014, -12.94488700934118341, -2.033253645871467057E-15 ) ) ;
#11564=CARTESIAN_POINT ( 'NONE',  ( 1.377327726974544753, -148.4679005553610125, 1.573913393350005796 ) ) ;
#11565=B_SPLINE_CURVE_WITH_KNOTS ( 'NONE', 3,
 ( #7741, #12027, #1101, #5429 ),
 .UNSPECIFIED., .F., .F.,
 ( 4, 4 ),
 ( 0.000000000000000000, 1.000000000000000000 ),
 .UNSPECIFIED. ) ;
#11567=ORIENTED_EDGE ( 'NONE', *, *, #11598, .T. ) ;
#11570=DIRECTION ( 'NONE',  ( 2.797435172181644469E-17, -1.000000000000000000, 0.000000000000000000 ) ) ;
#11573=CARTESIAN_POINT ( 'NONE',  ( -12.97449437267217576, -39.59556244224027211, -3.094637852359278775E-15 ) ) ;
#11577=CARTESIAN_POINT ( 'NONE',  ( -10.00000000000000711, 139.9999999999999716, 2.500000000000000000 ) ) ;
#11578=FACE_OUTER_BOUND ( 'NONE', #7872, .T. ) ;
#11579=DIRECTION ( 'NONE',  ( -1.000000000000000000, 0.000000000000000000, 0.000000000000000000 ) ) ;
#11582=CARTESIAN_POINT ( 'NONE',  ( 5.770584880507684922, -114.4337404266380531, -1.236082595024905695 ) ) ;
#11584=DIRECTION ( 'NONE',  ( 0.5999999999999989786, -0.8000000000000008216, 0.000000000000000000 ) ) ;
#11586=ORIENTED_EDGE ( 'NONE', *, *, #632, .T. ) ;
#11588=ORIENTED_EDGE ( 'NONE', *, *, #3189, .T. ) ;
#11589=EDGE_CURVE ( 'NONE', #2825, #5181, #8630, .T. ) ;
#11591=CARTESIAN_POINT ( 'NONE',  ( 0.7069570379179631603, -145.1287559931344902, -2.290092706300334235 ) ) ;
#11592=CARTESIAN_POINT ( 'NONE',  ( 12.99553232110412893, 39.34908859458022334, 25.99106464220826851 ) ) ;
#11593=CARTESIAN_POINT ( 'NONE',  ( 10.69346802281034492, 40.17406817374066463, 1.263183422977906849E-15 ) ) ;
#11594=CARTESIAN_POINT ( 'NONE',  ( 1.870037860061202206, -80.63037769710965108, -9.873254449573801494 ) ) ;
#11595=CARTESIAN_POINT ( 'NONE',  ( 2.974540731479519701E-17, -1.063309978032472847, 1.877653204021102445E-18 ) ) ;
#11597=CARTESIAN_POINT ( 'NONE',  ( -8.385254915620290461, 3.280056672672170492, -16.77050983124058803 ) ) ;
#11598=EDGE_CURVE ( 'NONE', #6854, #6129, #12460, .T. ) ;
#11599=CARTESIAN_POINT ( 'NONE',  ( -10.00000000000000000, 97.99999999999994316, -0.5000000000000000000 ) ) ;
#11600=DIRECTION ( 'NONE',  ( -2.797435172181481150E-17, 1.000000000000000000, -1.765856845898762549E-18 ) ) ;
#11602=EDGE_CURVE ( 'NONE', #11415, #2835, #8874, .T. ) ;
#11605=CARTESIAN_POINT ( 'NONE',  ( -15.29705854078139282, -10.48808792804187284, -1.836308454097519790E-15 ) ) ;
#11609=DIRECTION ( 'NONE',  ( -1.000000000000000000, 0.000000000000000000, 0.000000000000000000 ) ) ;
#11610=AXIS2_PLACEMENT_3D ( 'NONE', #11243, #10329, #5914 ) ;
#11611=CARTESIAN_POINT ( 'NONE',  ( -12.65441377644764209, -89.44155844155457658, 5.520840484228807021 ) ) ;
#11614=B_SPLINE_CURVE_WITH_KNOTS ( 'NONE', 3,
 ( #4137, #7356, #5123, #2890 ),
 .UNSPECIFIED., .F., .F.,
 ( 4, 4 ),
 ( 0.000000000000000000, 1.000000000000000000 ),
 .UNSPECIFIED. ) ;
#11615=CYLINDRICAL_SURFACE ( 'NONE', #7570, 2.000000000000000000 ) ;
#11617=VECTOR ( 'NONE', #12911, 1000.000000000000000 ) ;
#11624=CARTESIAN_POINT ( 'NONE',  ( -10.69381717166375623, -2.714886977913000710, -2.620524279449481830E-15 ) ) ;
#11629=DIRECTION ( 'NONE',  ( -0.9923485843107423543, -2.797833471351478217E-17, -0.1234677578012386562 ) ) ;
#11631=CARTESIAN_POINT ( 'NONE',  ( -15.29705854078139460, -8.601520358636511432, -1.842971270612889916E-15 ) ) ;
#11632=ORIENTED_EDGE ( 'NONE', *, *, #6375, .T. ) ;
#11633=EDGE_CURVE ( 'NONE', #4067, #8513, #10862, .T. ) ;
#11634=CARTESIAN_POINT ( 'NONE',  ( -3.917571877187561391, 90.55481622686230025, -3.109379165354180241 ) ) ;
#11635=AXIS2_PLACEMENT_3D ( 'NONE', #10351, #8446, #12733 ) ;
#11637=CARTESIAN_POINT ( 'NONE',  ( -8.385254915620294014, -24.99427717735608212, 4.413631546192547049E-17 ) ) ;
#11639=LINE ( 'NONE', #2884, #10599 ) ;
#11640=DIRECTION ( 'NONE',  ( 1.000000000000000000, 0.000000000000000000, -0.000000000000000000 ) ) ;
#11641=CARTESIAN_POINT ( 'NONE',  ( -8.012933686896012375, -76.12121212232311507, -3.597289645623622967 ) ) ;
#11645=CARTESIAN_POINT ( 'NONE',  ( 0.1431275062634679851, -159.4724345549973918, -1.503676168307738870 ) ) ;
#11646=PLANE ( 'NONE',  #8850 ) ;
#11652=CARTESIAN_POINT ( 'NONE',  ( 0.3181136358666373787, -144.1302678916006812, -2.473221358873241016 ) ) ;
#11653=DIRECTION ( 'NONE',  ( -1.000000000000000000, 0.000000000000000000, 0.000000000000000000 ) ) ;
#11654=ADVANCED_FACE ( 'NONE', ( #12924 ), #219, .T. ) ;
#11656=ADVANCED_FACE ( 'NONE', ( #9548 ), #11779, .F. ) ;
#11659=CARTESIAN_POINT ( 'NONE',  ( -4.912780601956176163, -116.0400786845119114, -2.910660294657916314 ) ) ;
#11661=CARTESIAN_POINT ( 'NONE',  ( -15.29705854078138927, 64.91013567203349055, -30.59411708156278564 ) ) ;
#11662=CARTESIAN_POINT ( 'NONE',  ( 0.3001389404147826179, -80.00109702611953821, -10.02811144968829282 ) ) ;
#11668=CARTESIAN_POINT ( 'NONE',  ( 15.29705854078138927, 46.06057977201469100, 1.790347283588440388E-15 ) ) ;
#11671=CIRCLE ( 'NONE', #1599, 8.385254915620292238 ) ;
#11672=CARTESIAN_POINT ( 'NONE',  ( 8.385254915620290461, -12.94488700934118341, 16.77050983124058803 ) ) ;
#11676=CARTESIAN_POINT ( 'NONE',  ( -3.913402758220056121, -81.93939393932039650, 9.205743832036068497 ) ) ;
#11678=CARTESIAN_POINT ( 'NONE',  ( 12.85867081388377109, -161.0909090910740815, 2.071848600315243871 ) ) ;
#11681=CARTESIAN_POINT ( 'NONE',  ( 10.00000000000000000, 97.99999999999994316, -2.500000000000000000 ) ) ;
#11682=CARTESIAN_POINT ( 'NONE',  ( -10.69381717166375800, 25.55944687211528077, -2.674742811949561692E-15 ) ) ;
#11684=LINE ( 'NONE', #4514, #2527 ) ;
#11685=DIRECTION ( 'NONE',  ( -2.797435172181481150E-17, 1.000000000000000000, -1.765856845898762549E-18 ) ) ;
#11686=ORIENTED_EDGE ( 'NONE', *, *, #1122, .T. ) ;
#11687=ADVANCED_FACE ( 'NONE', ( #2444 ), #11222, .T. ) ;
#11689=EDGE_LOOP ( 'NONE', ( #3359, #4506, #1910, #6794 ) ) ;
#11690=CARTESIAN_POINT ( 'NONE',  ( 8.385254915620290461, 43.60378069071538221, -16.77050983124057737 ) ) ;
#11691=CARTESIAN_POINT ( 'NONE',  ( 15.29705854078138572, 66.79670324143890525, 3.746698755667520834E-15 ) ) ;
#11692=EDGE_CURVE ( 'NONE', #2348, #4358, #1040, .T. ) ;
#11693=CARTESIAN_POINT ( 'NONE',  ( 10.69346802281034670, 30.74929022373126841, 1.274817642836897748E-15 ) ) ;
#11695=CARTESIAN_POINT ( 'NONE',  ( 0.6082774961674913827, -152.6296145370220358, 1.642986734028079709 ) ) ;
#11700=CARTESIAN_POINT ( 'NONE',  ( -8.385254915620294014, 24.75422479069652582, -4.371241731156832241E-17 ) ) ;
#11707=CARTESIAN_POINT ( 'NONE',  ( 12.99579180576516535, 7.534841976936129448, 0.000000000000000000 ) ) ;
#11708=DIRECTION ( 'NONE',  ( -2.797435172181481150E-17, 1.000000000000000000, -1.765856845898762549E-18 ) ) ;
#11713=CARTESIAN_POINT ( 'NONE',  ( -0.01927387650405660430, -127.9334134464769335, 4.304559060634273848 ) ) ;
#11714=DIRECTION ( 'NONE',  ( -1.000000000000000000, 0.000000000000000000, 0.000000000000000000 ) ) ;
#11715=ORIENTED_EDGE ( 'NONE', *, *, #636, .T. ) ;
#11716=ORIENTED_EDGE ( 'NONE', *, *, #3680, .F. ) ;
#11722=CARTESIAN_POINT ( 'NONE',  ( -25.00000000000000355, 120.0000000000000284, 2.500000000000000000 ) ) ;
#11723=CARTESIAN_POINT ( 'NONE',  ( -5.570638609096381089, -114.5775772725542083, -1.854390173297266742 ) ) ;
#11724=CARTESIAN_POINT ( 'NONE',  ( -8.385254915620292238, 5.904668890677671200, -2.066539263199666360E-15 ) ) ;
#11725=CARTESIAN_POINT ( 'NONE',  ( -3.189539364161578128, -137.4545454545680627, 1.430838129453288143 ) ) ;
#11726=CARTESIAN_POINT ( 'NONE',  ( 9.860966656300464095, -69.99999999999933209, 1.730751479080362865 ) ) ;
#11727=CARTESIAN_POINT ( 'NONE',  ( -10.69346802281034492, 21.32451227372186864, -2.671336073255822280E-15 ) ) ;
#11728=CARTESIAN_POINT ( 'NONE',  ( -10.13852281052241189, -69.87878787878712217, 0.9720347947262422128 ) ) ;
#11729=CARTESIAN_POINT ( 'NONE',  ( 1.119237408740483668E-15, -40.00941361824963849, 7.065089693818137167E-17 ) ) ;
#11731=TOROIDAL_SURFACE ( 'NONE', #7258, 42.00000000000001421, 2.000000000000000000 ) ;
#11733=EDGE_CURVE ( 'NONE', #4358, #2229, #5973, .T. ) ;
#11734=ORIENTED_EDGE ( 'NONE', *, *, #8071, .T. ) ;
#11735=CARTESIAN_POINT ( 'NONE',  ( 10.69381717166375267, 72.68333662216238622, 1.216686267861946676E-15 ) ) ;
#11737=CARTESIAN_POINT ( 'NONE',  ( -57.42880470198044662, -62.63636363089489123, -5.311255545846308657 ) ) ;
#11738=VERTEX_POINT ( 'NONE', #8823 ) ;
#11740=DIRECTION ( 'NONE',  ( -2.797435172181481150E-17, 1.000000000000000000, -1.765856845898762549E-18 ) ) ;
#11741=ORIENTED_EDGE ( 'NONE', *, *, #7546, .T. ) ;
#11744=FACE_OUTER_BOUND ( 'NONE', #9368, .T. ) ;
#11745=CARTESIAN_POINT ( 'NONE',  ( 10.69346802281034314, 2.474956373702985601, 21.38693604562069694 ) ) ;
#11747=CARTESIAN_POINT ( 'NONE',  ( 4.246087656260705501, -68.90909090936584391, -1.771789674505831247 ) ) ;
#11750=CARTESIAN_POINT ( 'NONE',  ( 10.00000000000000000, 90.00000000000000000, -0.5000000000000000000 ) ) ;
#11752=DIRECTION ( 'NONE',  ( 0.000000000000000000, 0.000000000000000000, 1.000000000000000000 ) ) ;
#11753=AXIS2_PLACEMENT_3D ( 'NONE', #3248, #3449, #6756 ) ;
#11756=EDGE_CURVE ( 'NONE', #30, #8596, #3712, .T. ) ;
#11759=ORIENTED_EDGE ( 'NONE', *, *, #10287, .F. ) ;
#11762=CARTESIAN_POINT ( 'NONE',  ( -10.69381717166375978, 53.83378072214353693, 21.38763434332750890 ) ) ;
#11765=CARTESIAN_POINT ( 'NONE',  ( -10.69346802281034847, 11.89973432371241202, 21.38693604562068629 ) ) ;
#11766=ORIENTED_EDGE ( 'NONE', *, *, #11489, .F. ) ;
#11767=VERTEX_POINT ( 'NONE', #9889 ) ;
#11768=VERTEX_POINT ( 'NONE', #11151 ) ;
#11769=AXIS2_PLACEMENT_3D ( 'NONE', #12986, #10715, #8616 ) ;
#11771=AXIS2_PLACEMENT_3D ( 'NONE', #3833, #7126, #2789 ) ;
#11776=DIRECTION ( 'NONE',  ( 5.551115123125776539E-17, -1.000000000000000000, -3.944304526105059027E-31 ) ) ;
#11777=CARTESIAN_POINT ( 'NONE',  ( 40.00000000000000711, 100.0000000000000000, 0.5000000000000000000 ) ) ;
#11778=AXIS2_PLACEMENT_3D ( 'NONE', #2491, #7672, #13104 ) ;
#11779=PLANE ( 'NONE',  #6855 ) ;
#11781=CARTESIAN_POINT ( 'NONE',  ( -4.525117841679046293, -85.05660262901220392, 8.349665357795196030 ) ) ;
#11783=ORIENTED_EDGE ( 'NONE', *, *, #4444, .F. ) ;
#11785=VECTOR ( 'NONE', #11406, 1000.000000000000000 ) ;
#11786=CARTESIAN_POINT ( 'NONE',  ( -4.330127018922197202, 91.82970358694005597, 2.500000000000001332 ) ) ;
#11789=CARTESIAN_POINT ( 'NONE',  ( -10.69381717166375800, -2.714886977913000710, 21.38763434332750890 ) ) ;
#11790=CARTESIAN_POINT ( 'NONE',  ( -8.385254915620292238, 40.97916847270985841, -16.77050983124058803 ) ) ;
#11791=FACE_OUTER_BOUND ( 'NONE', #9439, .T. ) ;
#11792=CARTESIAN_POINT ( 'NONE',  ( -10.69381717166375623, 6.709890972096426154, -2.632585121279762084E-15 ) ) ;
#11793=CARTESIAN_POINT ( 'NONE',  ( 1.134746186788315070, -154.2164502155151524, 0.2399094883713628612 ) ) ;
#11795=DIRECTION ( 'NONE',  ( -1.000000000000000000, 0.000000000000000000, 0.000000000000000000 ) ) ;
#11797=CARTESIAN_POINT ( 'NONE',  ( -9.940250983052290934, -69.87878787878452158, -1.425521750854495506 ) ) ;
#11798=CARTESIAN_POINT ( 'NONE',  ( 12.99553232110413958, -17.19957910547634228, 25.99106464220828983 ) ) ;
#11799=DIRECTION ( 'NONE',  ( -0.000000000000000000, -0.000000000000000000, -1.000000000000000000 ) ) ;
#11802=EDGE_LOOP ( 'NONE', ( #13069, #3640, #9055, #3897 ) ) ;
#11810=CARTESIAN_POINT ( 'NONE',  ( -8.385254915620297567, 24.75422479069652937, 16.77050983124058803 ) ) ;
#11813=CARTESIAN_POINT ( 'NONE',  ( -15.29705854078138749, 10.24803554138234496, -3.766461023514128305E-15 ) ) ;
#11818=AXIS2_PLACEMENT_3D ( 'NONE', #9397, #1887, #7341 ) ;
#11819=AXIS2_PLACEMENT_3D ( 'NONE', #8481, #2100, #2442 ) ;
#11820=EDGE_CURVE ( 'NONE', #11393, #8022, #3940, .T. ) ;
#11822=ORIENTED_EDGE ( 'NONE', *, *, #11006, .F. ) ;
#11826=FACE_OUTER_BOUND ( 'NONE', #1542, .T. ) ;
#11827=EDGE_CURVE ( 'NONE', #6325, #10679, #9318, .T. ) ;
#11831=AXIS2_PLACEMENT_3D ( 'NONE', #12580, #11708, #6316 ) ;
#11833=ORIENTED_EDGE ( 'NONE', *, *, #1741, .T. ) ;
#11834=ORIENTED_EDGE ( 'NONE', *, *, #5390, .F. ) ;
#11836=AXIS2_PLACEMENT_3D ( 'NONE', #5566, #2079, #8459 ) ;
#11837=VERTEX_POINT ( 'NONE', #6425 ) ;
#11841=( BOUNDED_SURFACE ( )  B_SPLINE_SURFACE ( 3, 3, ( 
 ( #4829, #3765, #6856, #1797 ),
 ( #5804, #11274, #5883, #9103 ),
 ( #10156, #9165, #11134, #13490 ),
 ( #13556, #3975, #761, #8251 ) ),
 .UNSPECIFIED., .F., .F., .T. ) 
 B_SPLINE_SURFACE_WITH_KNOTS ( ( 4, 4 ),
 ( 4, 4 ),
 ( 0.000000000000000000, 1.000000000000000000 ),
 ( 0.000000000000000000, 1.000000000000000000 ),
 .UNSPECIFIED. ) 
 GEOMETRIC_REPRESENTATION_ITEM ( )  RATIONAL_B_SPLINE_SURFACE ( (
 ( 1.000000000000000000, 0.3333333333333334259, 0.3333333333333334259, 1.000000000000000000),
 ( 1.000000000000000000, 0.3333333333333334259, 0.3333333333333334259, 1.000000000000000000),
 ( 1.000000000000000000, 0.3333333333333334259, 0.3333333333333334259, 1.000000000000000000),
 ( 1.000000000000000000, 0.3333333333333334259, 0.3333333333333334259, 1.000000000000000000) ) ) 
 REPRESENTATION_ITEM ( '' )  SURFACE ( )  );
#11846=CARTESIAN_POINT ( 'NONE',  ( -1.409802153637102151, -82.49939887521887272, 9.633183655277679946 ) ) ;
#11853=CARTESIAN_POINT ( 'NONE',  ( -2.766098618134340104, 90.01525736159538837, 4.178197917109232051 ) ) ;
#11854=CARTESIAN_POINT ( 'NONE',  ( -0.2462491701482444895, -80.00109949033800660, 10.02538131881691008 ) ) ;
#11855=ORIENTED_EDGE ( 'NONE', *, *, #11273, .T. ) ;
#11856=CARTESIAN_POINT ( 'NONE',  ( -15.29705854078138749, 10.24803554138234496, -1.809656371776380929E-17 ) ) ;
#11857=CARTESIAN_POINT ( 'NONE',  ( 1.214223716166046518, -80.16973037252847689, -10.05352466437349612 ) ) ;
#11858=CARTESIAN_POINT ( 'NONE',  ( 8.385254915620294014, 5.904668890677672088, -16.77050983124058092 ) ) ;
#11861=CARTESIAN_POINT ( 'NONE',  ( 0.03865624730933259895, -158.0606060602139564, 1.868422726205244189 ) ) ;
#11862=EDGE_CURVE ( 'NONE', #6545, #2529, #12237, .T. ) ;
#11864=CARTESIAN_POINT ( 'NONE',  ( -9.997547090296809102, -68.99999999999981526, -0.6397344882394256915 ) ) ;
#11868=EDGE_LOOP ( 'NONE', ( #1514, #13439, #4079, #6774 ) ) ;
#11870=CARTESIAN_POINT ( 'NONE',  ( -12.99579180576516535, 73.50828762700210461, -25.99158361153033425 ) ) ;
#11872=ORIENTED_EDGE ( 'NONE', *, *, #4051, .T. ) ;
#11875=CARTESIAN_POINT ( 'NONE',  ( 6.991987007918878033E-16, -24.99427717735608212, 4.413631546192547049E-17 ) ) ;
#11877=CARTESIAN_POINT ( 'NONE',  ( -39.99999999999999289, 120.0000000000000284, 2.500000000000000000 ) ) ;
#11880=CARTESIAN_POINT ( 'NONE',  ( -12.99553232110414491, 1.649976794542511893, -1.597320951662050367E-15 ) ) ;
#11890=EDGE_CURVE ( 'NONE', #3535, #1419, #6192, .T. ) ;
#11891=CARTESIAN_POINT ( 'NONE',  ( 9.628507540654561270E-16, -34.41905512736551032, 6.077912412602530076E-17 ) ) ;
#11893=B_SPLINE_CURVE_WITH_KNOTS ( 'NONE', 3,
 ( #5876, #4591, #2637, #10147 ),
 .UNSPECIFIED., .F., .F.,
 ( 4, 4 ),
 ( 0.000000000000000000, 1.000000000000000000 ),
 .UNSPECIFIED. ) ;
#11894=VERTEX_POINT ( 'NONE', #3122 ) ;
#11896=DIRECTION ( 'NONE',  ( -1.000000000000000000, 0.000000000000000000, 0.000000000000000000 ) ) ;
#11897=DIRECTION ( 'NONE',  ( 1.000000000000000000, 1.632680918566407779E-15, 0.000000000000000000 ) ) ;
#11904=ORIENTED_EDGE ( 'NONE', *, *, #6112, .F. ) ;
#11905=DIRECTION ( 'NONE',  ( -2.797435172181481150E-17, 1.000000000000000000, -1.765856845898762549E-18 ) ) ;
#11909=DIRECTION ( 'NONE',  ( 0.000000000000000000, 0.000000000000000000, -1.000000000000000000 ) ) ;
#11912=CARTESIAN_POINT ( 'NONE',  ( -12.99579180576517246, 64.08350967699263379, -1.817850092276246042E-15 ) ) ;
#11913=FACE_OUTER_BOUND ( 'NONE', #1373, .T. ) ;
#11917=VERTEX_POINT ( 'NONE', #11356 ) ;
#11919=EDGE_CURVE ( 'NONE', #5181, #11519, #1927, .T. ) ;
#11921=CARTESIAN_POINT ( 'NONE',  ( -3.159504973698680885, 90.09612598291141694, 3.878748273749980768 ) ) ;
#11922=CARTESIAN_POINT ( 'NONE',  ( 0.1244050240884003455, -80.00111861713446615, 10.00661217103304068 ) ) ;
#11925=PRESENTATION_STYLE_ASSIGNMENT (( #7648 ) ) ;
#11926=CARTESIAN_POINT ( 'NONE',  ( 15.29705854078139105, 36.63580182200523438, 3.746698755667522411E-15 ) ) ;
#11931=CARTESIAN_POINT ( 'NONE',  ( 12.99579180576516535, 45.23395377697384134, 0.000000000000000000 ) ) ;
#11932=CARTESIAN_POINT ( 'NONE',  ( -10.69346802281034847, -16.37459952631584059, 21.38693604562068984 ) ) ;
#11936=EDGE_LOOP ( 'NONE', ( #4144, #11766, #13520, #532 ) ) ;
#11939=EDGE_LOOP ( 'NONE', ( #4984, #5449, #2941, #8264 ) ) ;
#11940=EDGE_CURVE ( 'NONE', #7842, #5381, #12923, .T. ) ;
#11942=DIRECTION ( 'NONE',  ( -0.1234677578012386562, -1.701584941912606716E-18, 0.9923485843107423543 ) ) ;
#11943=ORIENTED_EDGE ( 'NONE', *, *, #2849, .F. ) ;
#11944=LINE ( 'NONE', #5633, #3921 ) ;
#11945=ORIENTED_EDGE ( 'NONE', *, *, #6644, .F. ) ;
#11947=CARTESIAN_POINT ( 'NONE',  ( -10.69346802281035202, 2.474956373702985157, 21.38693604562069339 ) ) ;
#11950=FACE_OUTER_BOUND ( 'NONE', #5157, .T. ) ;
#11952=CARTESIAN_POINT ( 'NONE',  ( -15.29705854078140170, -29.33764382806072746, -1.769737219441121578E-15 ) ) ;
#11953=CARTESIAN_POINT ( 'NONE',  ( -3.554095123023855901E-16, 12.70483462268159869, -2.243491919447391838E-17 ) ) ;
#11954=CARTESIAN_POINT ( 'NONE',  ( -15.29705854078139282, 17.78624592198638155, 30.59411708156276788 ) ) ;
#11955=B_SPLINE_CURVE_WITH_KNOTS ( 'NONE', 3,
 ( #6489, #185, #4661, #10886 ),
 .UNSPECIFIED., .F., .F.,
 ( 4, 4 ),
 ( 0.000000000000000000, 1.000000000000000000 ),
 .UNSPECIFIED. ) ;
#11956=ORIENTED_EDGE ( 'NONE', *, *, #4051, .F. ) ;
#11958=VERTEX_POINT ( 'NONE', #11750 ) ;
#11959=DIRECTION ( 'NONE',  ( -2.797435172181481150E-17, 1.000000000000000000, -1.765856845898762549E-18 ) ) ;
#11962=CARTESIAN_POINT ( 'NONE',  ( -10.69381717166375800, 25.55944687211528077, -1.399883545467522885E-15 ) ) ;
#11963=CIRCLE ( 'NONE', #8602, 15.29705854078138927 ) ;
#11964=CARTESIAN_POINT ( 'NONE',  ( -8.385254915620295790, 40.97916847270985130, -7.236334518677345233E-17 ) ) ;
#11970=EDGE_LOOP ( 'NONE', ( #6927, #8473, #5901, #6373, #4101, #3948, #7556 ) ) ;
#11972=AXIS2_PLACEMENT_3D ( 'NONE', #13299, #2536, #7861 ) ;
#11974=DIRECTION ( 'NONE',  ( 2.797435172181480534E-17, -1.000000000000000000, 1.765856845898762164E-18 ) ) ;
#11976=DIRECTION ( 'NONE',  ( -2.797435172181481150E-17, 1.000000000000000000, -1.765856845898762549E-18 ) ) ;
#11977=AXIS2_PLACEMENT_3D ( 'NONE', #9001, #11245, #1631 ) ;
#11978=EDGE_CURVE ( 'NONE', #1745, #7988, #8644, .T. ) ;
#11982=DIRECTION ( 'NONE',  ( -1.000000000000000000, 0.000000000000000000, 0.000000000000000000 ) ) ;
#11985=AXIS2_PLACEMENT_3D ( 'NONE', #7951, #3883, #12306 ) ;
#11993=CARTESIAN_POINT ( 'NONE',  ( -10.00000000000000711, 92.00000000000000000, -2.500000000000000000 ) ) ;
#11995=EDGE_CURVE ( 'NONE', #11418, #5860, #3270, .T. ) ;
#11997=CARTESIAN_POINT ( 'NONE',  ( -49.99999999999999289, 120.0000000000000284, 2.500000000000000000 ) ) ;
#12000=DIRECTION ( 'NONE',  ( 2.797435172181480534E-17, -1.000000000000000000, 1.765856845898762164E-18 ) ) ;
#12005=SURFACE_STYLE_FILL_AREA ( #241 ) ;
#12012=( BOUNDED_SURFACE ( )  B_SPLINE_SURFACE ( 3, 3, ( 
 ( #13349, #2648, #6918, #11207 ),
 ( #565, #12333, #9106, #2724 ),
 ( #1671, #7130, #6020, #10563 ),
 ( #13698, #12682, #9513, #3062 ) ),
 .UNSPECIFIED., .F., .F., .T. ) 
 B_SPLINE_SURFACE_WITH_KNOTS ( ( 4, 4 ),
 ( 4, 4 ),
 ( 0.000000000000000000, 1.000000000000000000 ),
 ( 0.000000000000000000, 1.000000000000000000 ),
 .UNSPECIFIED. ) 
 GEOMETRIC_REPRESENTATION_ITEM ( )  RATIONAL_B_SPLINE_SURFACE ( (
 ( 1.000000000000000000, 0.3333333333333334259, 0.3333333333333334259, 1.000000000000000000),
 ( 1.000000000000000000, 0.3333333333333334259, 0.3333333333333334259, 1.000000000000000000),
 ( 1.000000000000000000, 0.3333333333333334259, 0.3333333333333334259, 1.000000000000000000),
 ( 1.000000000000000000, 0.3333333333333334259, 0.3333333333333334259, 1.000000000000000000) ) ) 
 REPRESENTATION_ITEM ( '' )  SURFACE ( )  );
#12016=LINE ( 'NONE', #2403, #1233 ) ;
#12019=CARTESIAN_POINT ( 'NONE',  ( -10.69381717166375800, 25.55944687211528077, -1.399883545467522885E-15 ) ) ;
#12027=CARTESIAN_POINT ( 'NONE',  ( -10.69346802281035202, 77.87317997377837742, -1.584597914529132607E-15 ) ) ;
#12028=CARTESIAN_POINT ( 'NONE',  ( 8.385254915620297567, -6.144721277337255927, 1.036136684519089207E-15 ) ) ;
#12030=ORIENTED_EDGE ( 'NONE', *, *, #571, .F. ) ;
#12031=CARTESIAN_POINT ( 'NONE',  ( -35.45454545454546036, 140.4866414850956744, 2.500000000000000000 ) ) ;
#12036=DIRECTION ( 'NONE',  ( -0.000000000000000000, -0.000000000000000000, -1.000000000000000000 ) ) ;
#12037=CARTESIAN_POINT ( 'NONE',  ( -12.99579180576517601, 54.65873172698324112, 25.99158361153033070 ) ) ;
#12038=EDGE_CURVE ( 'NONE', #6322, #2621, #9735, .T. ) ;
#12040=CARTESIAN_POINT ( 'NONE',  ( 9.636121582682617870, -72.23759216827741625, 2.995460419705799904 ) ) ;
#12041=ORIENTED_EDGE ( 'NONE', *, *, #7534, .T. ) ;
#12042=VERTEX_POINT ( 'NONE', #12896 ) ;
#12043=VECTOR ( 'NONE', #2661, 1000.000000000000000 ) ;
#12046=CARTESIAN_POINT ( 'NONE',  ( 12.99579180576516713, 54.65873172698324112, 0.000000000000000000 ) ) ;
#12050=LINE ( 'NONE', #1129, #1086 ) ;
#12051=LINE ( 'NONE', #4772, #12567 ) ;
#12052=CIRCLE ( 'NONE', #8260, 48.00000000000001421 ) ;
#12053=DIRECTION ( 'NONE',  ( 1.000000000000000000, 0.000000000000000000, 0.000000000000000000 ) ) ;
#12055=CARTESIAN_POINT ( 'NONE',  ( -1.698372594682201253, -102.6769990425255799, -7.133712067588741768 ) ) ;
#12060=ADVANCED_FACE ( 'NONE', ( #10961 ), #1237, .T. ) ;
#12061=AXIS2_PLACEMENT_3D ( 'NONE', #10892, #11752, #5363 ) ;
#12062=FACE_OUTER_BOUND ( 'NONE', #3407, .T. ) ;
#12063=B_SPLINE_CURVE_WITH_KNOTS ( 'NONE', 3,
 ( #1197, #11912, #8553, #5460 ),
 .UNSPECIFIED., .F., .F.,
 ( 4, 4 ),
 ( 0.000000000000000000, 1.000000000000000000 ),
 .UNSPECIFIED. ) ;
#12067=ORIENTED_EDGE ( 'NONE', *, *, #2924, .F. ) ;
#12068=CARTESIAN_POINT ( 'NONE',  ( -10.69381717166375623, -2.714886977913000710, -1.300026693482923793E-15 ) ) ;
#12070=DIRECTION ( 'NONE',  ( -2.797435172181481150E-17, 1.000000000000000000, -1.765856845898762549E-18 ) ) ;
#12073=FACE_OUTER_BOUND ( 'NONE', #5826, .T. ) ;
#12074=CARTESIAN_POINT ( 'NONE',  ( -1.410017725396658984E-15, 50.40394642271930792, -8.900615385087330109E-17 ) ) ;
#12075=CIRCLE ( 'NONE', #3789, 15.29705854078138927 ) ;
#12076=DIRECTION ( 'NONE',  ( 0.8907235428302444635, 0.4545454545454587492, 0.000000000000000000 ) ) ;
#12079=ORIENTED_EDGE ( 'NONE', *, *, #11820, .F. ) ;
#12081=CARTESIAN_POINT ( 'NONE',  ( -2.517691654963332357E-15, 90.00000000000000000, -1.589271161308885878E-16 ) ) ;
#12084=AXIS2_PLACEMENT_3D ( 'NONE', #8369, #6268, #10540 ) ;
#12085=ADVANCED_FACE ( 'NONE', ( #188 ), #2263, .T. ) ;
#12086=ORIENTED_EDGE ( 'NONE', *, *, #10858, .F. ) ;
#12092=AXIS2_PLACEMENT_3D ( 'NONE', #12081, #2551, #13092 ) ;
#12093=CIRCLE ( 'NONE', #7, 15.29705854078139460 ) ;
#12094=CARTESIAN_POINT ( 'NONE',  ( 4.961407659643947810, 90.00000000000001421, -0.6346170828971222644 ) ) ;
#12095=CARTESIAN_POINT ( 'NONE',  ( 2.406219558548489190E-16, -8.601520358636511432, 1.518905361043589440E-17 ) ) ;
#12096=DIRECTION ( 'NONE',  ( 0.000000000000000000, 0.000000000000000000, 1.000000000000000000 ) ) ;
#12098=CARTESIAN_POINT ( 'NONE',  ( -10.11144051725924520, -69.99977036137985920, 0.2534939247371171822 ) ) ;
#12099=CARTESIAN_POINT ( 'NONE',  ( -12.99579180576517778, -30.16426982310158422, 25.99158361153034136 ) ) ;
#12100=LINE ( 'NONE', #1509, #4526 ) ;
#12101=CARTESIAN_POINT ( 'NONE',  ( -8.385254915620294014, -6.144721277337256815, -16.77050983124059513 ) ) ;
#12102=CIRCLE ( 'NONE', #9427, 15.29705854078140170 ) ;
#12103=ADVANCED_FACE ( 'NONE', ( #10209 ), #9517, .T. ) ;
#12104=ORIENTED_EDGE ( 'NONE', *, *, #7396, .F. ) ;
#12106=ORIENTED_EDGE ( 'NONE', *, *, #7873, .F. ) ;
#12107=EDGE_CURVE ( 'NONE', #1315, #1460, #10146, .T. ) ;
#12108=ORIENTED_EDGE ( 'NONE', *, *, #13252, .T. ) ;
#12119=CARTESIAN_POINT ( 'NONE',  ( 9.876538003337365978, -71.62961015055314817, 2.126563534463134619 ) ) ;
#12120=ORIENTED_EDGE ( 'NONE', *, *, #8833, .T. ) ;
#12123=EDGE_CURVE ( 'NONE', #3017, #1421, #3729, .T. ) ;
#12125=ORIENTED_EDGE ( 'NONE', *, *, #12304, .T. ) ;
#12132=CARTESIAN_POINT ( 'NONE',  ( 15.29705854078138749, 76.22148119144830503, 3.746698755667522411E-15 ) ) ;
#12135=DIRECTION ( 'NONE',  ( -0.000000000000000000, -0.000000000000000000, -1.000000000000000000 ) ) ;
#12136=LINE ( 'NONE', #4476, #1872 ) ;
#12137=FACE_OUTER_BOUND ( 'NONE', #1679, .T. ) ;
#12138=ORIENTED_EDGE ( 'NONE', *, *, #6375, .F. ) ;
#12139=ORIENTED_EDGE ( 'NONE', *, *, #9381, .F. ) ;
#12140=CARTESIAN_POINT ( 'NONE',  ( -8.567019981000800755, -91.60288616555511965, -1.484956459547787544 ) ) ;
#12143=CARTESIAN_POINT ( 'NONE',  ( -1.024078386997803625, -80.66666666666729668, 9.976024522091169189 ) ) ;
#12145=CARTESIAN_POINT ( 'NONE',  ( 4.330127018922196314, 91.72908881866754882, 2.499999999999993783 ) ) ;
#12149=CARTESIAN_POINT ( 'NONE',  ( 0.2890385494233890795, -128.7272727272696500, -4.499839249777167538 ) ) ;
#12150=CARTESIAN_POINT ( 'NONE',  ( 1.958204620527036497E-15, -70.00000000000000000, 1.236099792129133461E-16 ) ) ;
#12154=EDGE_LOOP ( 'NONE', ( #13020, #7137, #10596, #2677 ) ) ;
#12156=CARTESIAN_POINT ( 'NONE',  ( 0.5086153989323403124, -157.9221515666981190, 1.416975838558779177 ) ) ;
#12161=CARTESIAN_POINT ( 'NONE',  ( -8.385254915620292238, 79.99058638175036151, -1.412519245696701158E-16 ) ) ;
#12167=DIRECTION ( 'NONE',  ( -0.4545454545454531425, -0.8907235428302472391, 0.000000000000000000 ) ) ;
#12168=CARTESIAN_POINT ( 'NONE',  ( -10.69381717166375090, 44.40900277213413716, -21.38763434332750890 ) ) ;
#12171=LINE ( 'NONE', #6903, #5980 ) ;
#12172=CARTESIAN_POINT ( 'NONE',  ( -10.10544246792081857, -70.44230941534301849, -0.3214603539705591650 ) ) ;
#12174=CARTESIAN_POINT ( 'NONE',  ( -8.385254915620294014, 90.00000000000000000, -1.589271161308885878E-16 ) ) ;
#12176=VECTOR ( 'NONE', #2238, 1000.000000000000000 ) ;
#12179=CARTESIAN_POINT ( 'NONE',  ( -6.733243228433030581, -82.89610389607871355, 12.92256141468849506 ) ) ;
#12180=VECTOR ( 'NONE', #1550, 1000.000000000000000 ) ;
#12182=( GEOMETRIC_REPRESENTATION_CONTEXT ( 3 ) GLOBAL_UNCERTAINTY_ASSIGNED_CONTEXT ( ( #7133 ) ) GLOBAL_UNIT_ASSIGNED_CONTEXT ( ( #2760, #11304, #9209 ) ) REPRESENTATION_CONTEXT ( 'NONE', 'WORKASPACE' ) );
#12183=CARTESIAN_POINT ( 'NONE',  ( 8.385254915620292238, 50.40394642271930792, 9.355740606675297531E-16 ) ) ;
#12185=ORIENTED_EDGE ( 'NONE', *, *, #275, .T. ) ;
#12190=EDGE_CURVE ( 'NONE', #9797, #1472, #3060, .T. ) ;
#12191=DIRECTION ( 'NONE',  ( -2.797435172181481150E-17, 1.000000000000000000, -1.765856845898762549E-18 ) ) ;
#12192=CARTESIAN_POINT ( 'NONE',  ( 7.128864087426364016, -75.84752376712806665, 7.199434346136632357 ) ) ;
#12199=CARTESIAN_POINT ( 'NONE',  ( 12.99553232110415024, -26.62435705548576692, -25.99106464220828627 ) ) ;
#12201=ORIENTED_EDGE ( 'NONE', *, *, #7551, .F. ) ;
#12206=ADVANCED_FACE ( 'NONE', ( #8373 ), #7022, .T. ) ;
#12208=CARTESIAN_POINT ( 'NONE',  ( -10.69381717166375623, 34.98422482212468054, -1.433169162795722386E-15 ) ) ;
#12210=CARTESIAN_POINT ( 'NONE',  ( -1.520893302047029660, -106.0215521432844952, 6.750146769911295586 ) ) ;
#12211=CARTESIAN_POINT ( 'NONE',  ( -8.385254915620292238, 15.32944684068712782, -2.089804632053991565E-15 ) ) ;
#12213=EDGE_CURVE ( 'NONE', #1501, #2348, #6145, .T. ) ;
#12219=CARTESIAN_POINT ( 'NONE',  ( 9.807291687912153222, -69.33333333333652604, 2.012068907120017514 ) ) ;
#12220=ORIENTED_EDGE ( 'NONE', *, *, #1045, .T. ) ;
#12223=CARTESIAN_POINT ( 'NONE',  ( 10.69346802281034847, -35.22415542633469698, 0.000000000000000000 ) ) ;
#12226=CARTESIAN_POINT ( 'NONE',  ( 2.739930038170992344, -137.4545454545608720, 2.373837707219488280 ) ) ;
#12234=EDGE_LOOP ( 'NONE', ( #12963, #2674, #2030, #11021 ) ) ;
#12235=CARTESIAN_POINT ( 'NONE',  ( 0.7709178830051971465, -102.1536708361958716, -7.353836487445167158 ) ) ;
#12236=ADVANCED_FACE ( 'NONE', ( #10609 ), #13854, .T. ) ;
#12237=CIRCLE ( 'NONE', #5063, 15.29705854078139105 ) ;
#12238=LINE ( 'NONE', #13535, #5273 ) ;
#12240=VERTEX_POINT ( 'NONE', #11668 ) ;
#12242=ORIENTED_EDGE ( 'NONE', *, *, #6870, .T. ) ;
#12248=DIRECTION ( 'NONE',  ( -1.000000000000000000, 0.000000000000000000, 0.000000000000000000 ) ) ;
#12249=CARTESIAN_POINT ( 'NONE',  ( 12.99553232110414669, -26.62435705548577047, 0.000000000000000000 ) ) ;
#12254=CARTESIAN_POINT ( 'NONE',  ( 2.940534136604410875, -72.18181818207969513, 3.082537950474903088 ) ) ;
#12255=EDGE_CURVE ( 'NONE', #7855, #3210, #3907, .T. ) ;
#12256=AXIS2_PLACEMENT_3D ( 'NONE', #1601, #8122, #5729 ) ;
#12259=CARTESIAN_POINT ( 'NONE',  ( 6.733243228435068950, -82.89610389607662455, -12.92256141468959640 ) ) ;
#12260=CARTESIAN_POINT ( 'NONE',  ( 12.99579180576516535, 7.534841976936129448, 3.183050967463141802E-15 ) ) ;
#12262=CARTESIAN_POINT ( 'NONE',  ( 10.69346802281033781, 21.32451227372186864, 21.38693604562068629 ) ) ;
#12263=CARTESIAN_POINT ( 'NONE',  ( 14.13596196814456718, -39.17949320881311337, 28.27192393628914502 ) ) ;
#12268=EDGE_LOOP ( 'NONE', ( #6246, #7691, #3212, #1185 ) ) ;
#12270=ORIENTED_EDGE ( 'NONE', *, *, #2697, .T. ) ;
#12272=CARTESIAN_POINT ( 'NONE',  ( -15.29705854078138394, -36.87585420866476937, -30.59411708156277854 ) ) ;
#12274=CARTESIAN_POINT ( 'NONE',  ( -9.357262989153291244, -70.83714849354491605, -3.840749687708657767 ) ) ;
#12275=CARTESIAN_POINT ( 'NONE',  ( 10.00000000000000711, 139.9999999999999716, 0.5000000000000000000 ) ) ;
#12276=CARTESIAN_POINT ( 'NONE',  ( 8.182234252389633866, -94.33801111161687913, 1.656266771341373900 ) ) ;
#12281=DIRECTION ( 'NONE',  ( -2.797435172181481150E-17, 1.000000000000000000, -1.765856845898762549E-18 ) ) ;
#12283=DIRECTION ( 'NONE',  ( 0.000000000000000000, 0.000000000000000000, 1.000000000000000000 ) ) ;
#12285=CARTESIAN_POINT ( 'NONE',  ( -1.463793564954975146, -80.12121212121181202, 10.07802918118912139 ) ) ;
#12286=ORIENTED_EDGE ( 'NONE', *, *, #13832, .T. ) ;
#12287=CARTESIAN_POINT ( 'NONE',  ( 15.29705854078140170, -19.91286587805129926, 1.906846944237140710E-15 ) ) ;
#12290=DIRECTION ( 'NONE',  ( 0.9923485843107423543, 2.797833471351478217E-17, 0.1234677578012386562 ) ) ;
#12291=CARTESIAN_POINT ( 'NONE',  ( 4.855892414095402287, -117.0909090909090793, 4.610765637404218076 ) ) ;
#12292=CARTESIAN_POINT ( 'NONE',  ( -12.99579180576517068, 45.23395377697383424, 25.99158361153032004 ) ) ;
#12293=CARTESIAN_POINT ( 'NONE',  ( -4.418010223188907126, -106.9090909090898549, 5.547116815809651769 ) ) ;
#12294=DIRECTION ( 'NONE',  ( 1.000000000000000000, 0.000000000000000000, 0.000000000000000000 ) ) ;
#12295=CARTESIAN_POINT ( 'NONE',  ( -32.72727272727271952, 135.1423002281142089, -0.5000000000000000000 ) ) ;
#12297=ORIENTED_EDGE ( 'NONE', *, *, #9112, .T. ) ;
#12298=EDGE_LOOP ( 'NONE', ( #3467, #9416, #12771 ) ) ;
#12300=CARTESIAN_POINT ( 'NONE',  ( 1.146825886634105895, -155.8473912411174354, 1.122800904668010302 ) ) ;
#12302=CARTESIAN_POINT ( 'NONE',  ( -5.052187264070409967, -96.66555973379486488, -6.278296762411313736 ) ) ;
#12304=EDGE_CURVE ( 'NONE', #11415, #4734, #10091, .T. ) ;
#12306=DIRECTION ( 'NONE',  ( 1.000000000000000000, 0.000000000000000000, 0.000000000000000000 ) ) ;
#12308=DIRECTION ( 'NONE',  ( -1.000000000000000000, 0.000000000000000000, 0.000000000000000000 ) ) ;
#12311=ADVANCED_FACE ( 'NONE', ( #10475 ), #12669, .T. ) ;
#12316=CARTESIAN_POINT ( 'NONE',  ( -15.29705854078140170, -29.33764382806072746, 5.180607919632063331E-17 ) ) ;
#12317=CARTESIAN_POINT ( 'NONE',  ( 1.958204620527036497E-15, -70.00000000000000000, 1.236099792129133461E-16 ) ) ;
#12319=CARTESIAN_POINT ( 'NONE',  ( -10.69381717166375800, 63.25855867215300066, 21.38763434332750535 ) ) ;
#12320=CARTESIAN_POINT ( 'NONE',  ( 8.385254915620292238, 40.97916847270985130, 9.522168693316296019E-16 ) ) ;
#12321=AXIS2_PLACEMENT_3D ( 'NONE', #12597, #5081, #2056 ) ;
#12323=CARTESIAN_POINT ( 'NONE',  ( 2.886819890957835977, -105.1818181818214128, -3.599275682873738003 ) ) ;
#12324=VERTEX_POINT ( 'NONE', #1993 ) ;
#12326=ORIENTED_EDGE ( 'NONE', *, *, #12255, .F. ) ;
#12330=CARTESIAN_POINT ( 'NONE',  ( -1.275238607045734884, -147.1038961039145647, 4.986937111402549583 ) ) ;
#12332=CARTESIAN_POINT ( 'NONE',  ( -8.385254915620294014, 5.904668890677672088, 16.77050983124058092 ) ) ;
#12333=CARTESIAN_POINT ( 'NONE',  ( -12.99579180576517601, -20.73949187309215247, 25.99158361153034136 ) ) ;
#12334=AXIS2_PLACEMENT_3D ( 'NONE', #9769, #2473, #8937 ) ;
#12335=CARTESIAN_POINT ( 'NONE',  ( -12.99553232110414491, -36.04913500549519512, 25.99106464220827917 ) ) ;
#12339=CARTESIAN_POINT ( 'NONE',  ( 5.799822717052470544, -77.11029875732677397, 8.314269019852831732 ) ) ;
#12343=CARTESIAN_POINT ( 'NONE',  ( -10.69346802281034670, -25.79937747632526879, -2.581358761202454000E-15 ) ) ;
#12344=AXIS2_PLACEMENT_3D ( 'NONE', #762, #5028, #9382 ) ;
#12346=ORIENTED_EDGE ( 'NONE', *, *, #6112, .T. ) ;
#12349=CARTESIAN_POINT ( 'NONE',  ( -15.29705854078139282, -8.601520358636511432, 1.518905361043589440E-17 ) ) ;
#12350=CARTESIAN_POINT ( 'NONE',  ( -9.704377265674031250, -70.11112484213649054, -2.862656033565787794 ) ) ;
#12352=CARTESIAN_POINT ( 'NONE',  ( 1.395779086812880765, -82.48867648896566607, -9.636429481739551051 ) ) ;
#12355=CARTESIAN_POINT ( 'NONE',  ( -12.99553232110414491, 58.19864449459908684, 25.99106464220826851 ) ) ;
#12361=CARTESIAN_POINT ( 'NONE',  ( 10.69346802281034847, -25.79937747632526879, 2.619144277183853555E-15 ) ) ;
#12362=CARTESIAN_POINT ( 'NONE',  ( 7.668969345093573864, -75.54545454545474570, 6.730503492161126644 ) ) ;
#12363=EDGE_LOOP ( 'NONE', ( #1245, #9487, #9238, #12658 ) ) ;
#12364=CARTESIAN_POINT ( 'NONE',  ( 8.862685984072301792, -71.63821981287377128, 4.927609687620887691 ) ) ;
#12366=CARTESIAN_POINT ( 'NONE',  ( 6.764234067549970142, -111.2727272727265699, -0.6609924544552198133 ) ) ;
#12368=CARTESIAN_POINT ( 'NONE',  ( 2.557893175568158206, -128.7272727272670352, -3.337007314118542567 ) ) ;
#12379=ADVANCED_FACE ( 'NONE', ( #7584 ), #13010, .T. ) ;
#12380=VECTOR ( 'NONE', #11466, 1000.000000000000000 ) ;
#12381=CARTESIAN_POINT ( 'NONE',  ( 6.201497802824914807, -111.6673017749467078, -0.6065233957951752242 ) ) ;
#12386=FACE_OUTER_BOUND ( 'NONE', #8117, .T. ) ;
#12387=CARTESIAN_POINT ( 'NONE',  ( -0.9917158832135428703, -156.3625650723581941, -1.200616968270185048 ) ) ;
#12388=CYLINDRICAL_SURFACE ( 'NONE', #10336, 15.29705854078139460 ) ;
#12389=FACE_OUTER_BOUND ( 'NONE', #11936, .T. ) ;
#12391=EDGE_CURVE ( 'NONE', #2835, #3968, #10870, .T. ) ;
#12393=CARTESIAN_POINT ( 'NONE',  ( -10.69381717166375623, 63.25855867215299355, -1.533026014780321478E-15 ) ) ;
#12395=ORIENTED_EDGE ( 'NONE', *, *, #660, .T. ) ;
#12396=TOROIDAL_SURFACE ( 'NONE', #8566, 71.99999999999998579, 2.000000000000000000 ) ;
#12397=CARTESIAN_POINT ( 'NONE',  ( -1.800977217388287643, -65.63636364672284174, -1.354836293040065032 ) ) ;
#12401=CARTESIAN_POINT ( 'NONE',  ( -4.330127018922195425, 92.00000000000000000, -2.500000000000000000 ) ) ;
#12403=( BOUNDED_SURFACE ( )  B_SPLINE_SURFACE ( 3, 3, ( 
 ( #12934, #4412, #7508, #10728 ),
 ( #304, #13146, #3434, #5472 ),
 ( #12068, #11789, #12866, #2179 ),
 ( #9901, #6737, #4557, #7778 ) ),
 .UNSPECIFIED., .F., .F., .F. ) 
 B_SPLINE_SURFACE_WITH_KNOTS ( ( 4, 4 ),
 ( 4, 4 ),
 ( 0.000000000000000000, 1.000000000000000000 ),
 ( 0.000000000000000000, 1.000000000000000000 ),
 .UNSPECIFIED. ) 
 GEOMETRIC_REPRESENTATION_ITEM ( )  RATIONAL_B_SPLINE_SURFACE ( (
 ( 1.000000000000000000, 0.3333333333333334259, 0.3333333333333334259, 1.000000000000000000),
 ( 1.000000000000000000, 0.3333333333333334259, 0.3333333333333334259, 1.000000000000000000),
 ( 1.000000000000000000, 0.3333333333333334259, 0.3333333333333334259, 1.000000000000000000),
 ( 1.000000000000000000, 0.3333333333333334259, 0.3333333333333334259, 1.000000000000000000) ) ) 
 REPRESENTATION_ITEM ( '' )  SURFACE ( )  );
#12404=CARTESIAN_POINT ( 'NONE',  ( -18.84535726877603423, -167.3636363590141229, -7.741214182183449921 ) ) ;
#12406=DIRECTION ( 'NONE',  ( -1.000000000000000000, 0.000000000000000000, 0.000000000000000000 ) ) ;
#12410=VECTOR ( 'NONE', #11799, 1000.000000000000000 ) ;
#12411=CARTESIAN_POINT ( 'NONE',  ( -8.634227980725805551, -88.04976197785512682, 2.978358350864825255 ) ) ;
#12416=CYLINDRICAL_SURFACE ( 'NONE', #6500, 24.99999999999998934 ) ;
#12417=DIRECTION ( 'NONE',  ( 0.8907235428302473501, 0.4545454545454531425, -6.308085367188369928E-15 ) ) ;
#12418=CARTESIAN_POINT ( 'NONE',  ( -5.784531816357078249, -115.5952484847508117, 0.2985095753478224090 ) ) ;
#12423=CARTESIAN_POINT ( 'NONE',  ( 15.29705854078138927, -27.45107625865536960, 30.59411708156278564 ) ) ;
#12424=CARTESIAN_POINT ( 'NONE',  ( 6.374260517225430966, -76.81818181818142932, 7.989319691426051584 ) ) ;
#12425=EDGE_LOOP ( 'NONE', ( #2500, #7349, #880, #5890 ) ) ;
#12426=CARTESIAN_POINT ( 'NONE',  ( 3.656918997208050470, -76.68408298408331802, 9.436988895887294504 ) ) ;
#12428=DIRECTION ( 'NONE',  ( 1.000000000000000000, 0.000000000000000000, 0.000000000000000000 ) ) ;
#12429=CARTESIAN_POINT ( 'NONE',  ( 2.905947830705836399, -133.0909090908846224, -2.158723819797785826 ) ) ;
#12432=DIRECTION ( 'NONE',  ( -2.797435172181481150E-17, 1.000000000000000000, -1.765856845898762549E-18 ) ) ;
#12433=AXIS2_PLACEMENT_3D ( 'NONE', #6066, #7173, #8230 ) ;
#12439=ORIENTED_EDGE ( 'NONE', *, *, #2616, .T. ) ;
#12440=CARTESIAN_POINT ( 'NONE',  ( 5.713079006591276432, -108.6653251258257029, -3.322691064749034862 ) ) ;
#12441=EDGE_CURVE ( 'NONE', #4148, #11146, #5347, .T. ) ;
#12448=CYLINDRICAL_SURFACE ( 'NONE', #12433, 15.29705854078138927 ) ;
#12450=CARTESIAN_POINT ( 'NONE',  ( -0.6173387890061908800, -69.99999999999998579, 4.961742921553712549 ) ) ;
#12451=CARTESIAN_POINT ( 'NONE',  ( 0.5292784318607320904, -80.00108554120387794, -10.03971594810948709 ) ) ;
#12456=CARTESIAN_POINT ( 'NONE',  ( -15.29705854078139993, -19.91286587805129926, 3.516327053222078456E-17 ) ) ;
#12457=CARTESIAN_POINT ( 'NONE',  ( -10.69346802281034670, -16.37459952631584059, -1.251741741247135829E-15 ) ) ;
#12459=DIRECTION ( 'NONE',  ( -2.797435172181481150E-17, 1.000000000000000000, -1.765856845898762549E-18 ) ) ;
#12460=CIRCLE ( 'NONE', #2139, 15.29705854078139105 ) ;
#12461=ORIENTED_EDGE ( 'NONE', *, *, #13444, .F. ) ;
#12462=CARTESIAN_POINT ( 'NONE',  ( 10.69381717166375445, 53.83378072214353693, 1.239955467309983489E-15 ) ) ;
#12463=CARTESIAN_POINT ( 'NONE',  ( 10.82118823930636964, -118.2727272727259731, 9.720764081409937418 ) ) ;
#12468=CYLINDRICAL_SURFACE ( 'NONE', #4341, 2.000000000000000000 ) ;
#12469=AXIS2_PLACEMENT_3D ( 'NONE', #11076, #12135, #12053 ) ;
#12470=CARTESIAN_POINT ( 'NONE',  ( -8.139862572394246717E-16, 29.09759144140119957, -5.138218104596347907E-17 ) ) ;
#12473=CARTESIAN_POINT ( 'NONE',  ( 10.69346802281034137, 49.59884612375012836, 21.38693604562069694 ) ) ;
#12474=PLANE ( 'NONE',  #12620 ) ;
#12475=DIRECTION ( 'NONE',  ( -1.000000000000000000, 0.000000000000000000, 0.000000000000000000 ) ) ;
#12476=MANIFOLD_SOLID_BREP ( 'Cut-Revolve-Thin2', #8271 ) ;
#12478=AXIS2_PLACEMENT_3D ( 'NONE', #2992, #10428, #763 ) ;
#12479=DIRECTION ( 'NONE',  ( -1.000000000000000000, 0.000000000000000000, 0.000000000000000000 ) ) ;
#12480=( BOUNDED_SURFACE ( )  B_SPLINE_SURFACE ( 3, 3, ( 
 ( #1963, #12773, #10452, #853 ),
 ( #987, #12644, #5253, #6248 ),
 ( #10514, #921, #5186, #9541 ),
 ( #3143, #7555, #284, #5452 ) ),
 .UNSPECIFIED., .F., .F., .F. ) 
 B_SPLINE_SURFACE_WITH_KNOTS ( ( 4, 4 ),
 ( 4, 4 ),
 ( 0.000000000000000000, 1.000000000000000000 ),
 ( 0.000000000000000000, 1.000000000000000000 ),
 .UNSPECIFIED. ) 
 GEOMETRIC_REPRESENTATION_ITEM ( )  RATIONAL_B_SPLINE_SURFACE ( (
 ( 1.000000000000000000, 0.3333333333333334259, 0.3333333333333334259, 1.000000000000000000),
 ( 1.000000000000000000, 0.3333333333333334259, 0.3333333333333334259, 1.000000000000000000),
 ( 1.000000000000000000, 0.3333333333333334259, 0.3333333333333334259, 1.000000000000000000),
 ( 1.000000000000000000, 0.3333333333333334259, 0.3333333333333334259, 1.000000000000000000) ) ) 
 REPRESENTATION_ITEM ( '' )  SURFACE ( )  );
#12482=DIRECTION ( 'NONE',  ( 0.000000000000000000, -0.000000000000000000, 1.000000000000000000 ) ) ;
#12488=CARTESIAN_POINT ( 'NONE',  ( 7.901556246067206857, -95.03441247031096850, 2.400298799947536477 ) ) ;
#12490=ORIENTED_EDGE ( 'NONE', *, *, #1987, .F. ) ;
#12492=ORIENTED_EDGE ( 'NONE', *, *, #5940, .F. ) ;
#12493=CARTESIAN_POINT ( 'NONE',  ( 12.99553232110414491, -7.774801155466914970, 3.182987412051232562E-15 ) ) ;
#12495=B_SPLINE_CURVE_WITH_KNOTS ( 'NONE', 3,
 ( #3402, #7681, #11962, #2354 ),
 .UNSPECIFIED., .F., .F.,
 ( 4, 4 ),
 ( 0.000000000000000000, 1.000000000000000000 ),
 .UNSPECIFIED. ) ;
#12498=ORIENTED_EDGE ( 'NONE', *, *, #3817, .T. ) ;
#12501=CARTESIAN_POINT ( 'NONE',  ( -15.29705854078139460, 46.06057977201469100, 30.59411708156277498 ) ) ;
#12506=CARTESIAN_POINT ( 'NONE',  ( -0.5318696992121811906, -153.1606381718178227, -1.636362426323313413 ) ) ;
#12512=ORIENTED_EDGE ( 'NONE', *, *, #10136, .F. ) ;
#12513=CARTESIAN_POINT ( 'NONE',  ( 3.062175308430663989, -118.9477956384829582, 4.375409443047287184 ) ) ;
#12515=CARTESIAN_POINT ( 'NONE',  ( -8.139862572394246717E-16, 29.09759144140119957, -5.138218104596347907E-17 ) ) ;
#12516=CARTESIAN_POINT ( 'NONE',  ( 25.00000000000000355, 120.0000000000000284, -0.5000000000000000000 ) ) ;
#12518=CARTESIAN_POINT ( 'NONE',  ( -1.853002570266264915, -151.7308256017814188, 0.1000873228714606461 ) ) ;
#12520=CARTESIAN_POINT ( 'NONE',  ( 0.09220535803714466350, -163.8787878952597907, -3.538661136606733315 ) ) ;
#12521=DIRECTION ( 'NONE',  ( 1.000000000000000000, 0.000000000000000000, 0.000000000000000000 ) ) ;
#12522=DIRECTION ( 'NONE',  ( 0.8907235428302473501, -0.4545454545454531425, 0.000000000000000000 ) ) ;
#12525=CYLINDRICAL_SURFACE ( 'NONE', #9647, 15.29705854078139105 ) ;
#12526=DIRECTION ( 'NONE',  ( 0.000000000000000000, 0.000000000000000000, 1.000000000000000000 ) ) ;
#12528=EDGE_CURVE ( 'NONE', #9083, #9012, #4842, .T. ) ;
#12530=CARTESIAN_POINT ( 'NONE',  ( -8.827136188495221389E-16, 31.55439052270045508, -5.572053652267360357E-17 ) ) ;
#12531=EDGE_LOOP ( 'NONE', ( #10463, #10451, #6705, #5219 ) ) ;
#12534=CARTESIAN_POINT ( 'NONE',  ( -12.09338464843077077, -61.00000000000002842, 0.006909782851250131745 ) ) ;
#12536=EDGE_CURVE ( 'NONE', #4522, #2108, #5495, .T. ) ;
#12538=AXIS2_PLACEMENT_3D ( 'NONE', #11042, #554, #1440 ) ;
#12539=ORIENTED_EDGE ( 'NONE', *, *, #11312, .T. ) ;
#12540=CARTESIAN_POINT ( 'NONE',  ( 1.958204620527036497E-15, -70.00000000000000000, 1.236099792129133461E-16 ) ) ;
#12542=TOROIDAL_SURFACE ( 'NONE', #13220, 22.99999999999999289, 2.000000000000000000 ) ;
#12544=CARTESIAN_POINT ( 'NONE',  ( 8.723672207956152391, -129.7272727272730890, -9.720751085824081983 ) ) ;
#12545=CARTESIAN_POINT ( 'NONE',  ( 12.99553232110413248, 48.77386654458962312, 25.99106464220827917 ) ) ;
#12546=FACE_OUTER_BOUND ( 'NONE', #8294, .T. ) ;
#12547=EDGE_CURVE ( 'NONE', #4849, #4529, #9097, .T. ) ;
#12548=FACE_OUTER_BOUND ( 'NONE', #5284, .T. ) ;
#12550=CIRCLE ( 'NONE', #461, 15.29705854078139105 ) ;
#12552=EDGE_CURVE ( 'NONE', #1069, #13048, #4157, .T. ) ;
#12554=CARTESIAN_POINT ( 'NONE',  ( -4.302448071771068250, -82.51104542591967572, 8.727548302715668171 ) ) ;
#12556=ORIENTED_EDGE ( 'NONE', *, *, #4267, .T. ) ;
#12557=VERTEX_POINT ( 'NONE', #1489 ) ;
#12558=CARTESIAN_POINT ( 'NONE',  ( 8.385254915620294014, -22.36966495935058319, -16.77050983124058092 ) ) ;
#12561=AXIS2_PLACEMENT_3D ( 'NONE', #402, #13096, #11942 ) ;
#12562=CARTESIAN_POINT ( 'NONE',  ( -8.385254915620294014, 31.55439052270045508, -16.77050983124059158 ) ) ;
#12564=CARTESIAN_POINT ( 'NONE',  ( 2.249530157828166566, -133.0425321159758880, -2.931855161479524075 ) ) ;
#12567=VECTOR ( 'NONE', #8061, 1000.000000000000000 ) ;
#12568=EDGE_LOOP ( 'NONE', ( #7014, #8351, #338, #7975 ) ) ;
#12569=ADVANCED_FACE ( 'NONE', ( #531 ), #6960, .T. ) ;
#12571=AXIS2_PLACEMENT_3D ( 'NONE', #3594, #8712, #7591 ) ;
#12572=ORIENTED_EDGE ( 'NONE', *, *, #2669, .T. ) ;
#12573=CARTESIAN_POINT ( 'NONE',  ( -4.330127018922195425, 91.83037361138187293, -2.499999999999999556 ) ) ;
#12577=CARTESIAN_POINT ( 'NONE',  ( 9.736331930512850619, -69.99978782402618549, 2.722951059031191612 ) ) ;
#12579=CARTESIAN_POINT ( 'NONE',  ( -9.849578953073196530, -91.60173160172604412, 1.758148290372610223 ) ) ;
#12580=CARTESIAN_POINT ( 'NONE',  ( 5.042740091284176371E-16, -18.02629830864596627, 3.183186227453577089E-17 ) ) ;
#12585=CARTESIAN_POINT ( 'NONE',  ( -2.914768773580740380, -136.4521213004123865, 1.564187473038843423 ) ) ;
#12589=VERTEX_POINT ( 'NONE', #10188 ) ;
#12591=CARTESIAN_POINT ( 'NONE',  ( -15.29705854078138749, 38.52236939141059935, -2.009399357253887220E-15 ) ) ;
#12594=CARTESIAN_POINT ( 'NONE',  ( 6.068924878052031069, -84.14159528350513995, -7.406228478373899193 ) ) ;
#12595=FACE_OUTER_BOUND ( 'NONE', #10153, .T. ) ;
#12597=CARTESIAN_POINT ( 'NONE',  ( 0.000000000000000000, 71.01020514433645303, -0.5000000000000000000 ) ) ;
#12600=DIRECTION ( 'NONE',  ( 1.000000000000000000, 1.665334536937735599E-15, 0.000000000000000000 ) ) ;
#12603=ORIENTED_EDGE ( 'NONE', *, *, #4759, .T. ) ;
#12605=CARTESIAN_POINT ( 'NONE',  ( -4.588105241658432476, -161.0909090906812082, 0.3432044964271254162 ) ) ;
#12610=CARTESIAN_POINT ( 'NONE',  ( -8.385254915620292238, -3.520109059331727686, 6.216008680731233110E-18 ) ) ;
#12615=CARTESIAN_POINT ( 'NONE',  ( 3.867425345466886100, -111.7272727272767554, -3.383301718857324225 ) ) ;
#12616=CARTESIAN_POINT ( 'NONE',  ( 15.29705854078139282, 74.33491362204294717, 1.740418857596141236E-15 ) ) ;
#12620=AXIS2_PLACEMENT_3D ( 'NONE', #6292, #10430, #4173 ) ;
#12621=ORIENTED_EDGE ( 'NONE', *, *, #3984, .F. ) ;
#12622=CARTESIAN_POINT ( 'NONE',  ( -2.081238242702796892, -80.78225910474277782, 9.793491045833961905 ) ) ;
#12626=CIRCLE ( 'NONE', #3404, 8.385254915620292238 ) ;
#12627=CARTESIAN_POINT ( 'NONE',  ( -10.69381717166375623, -21.56444287793185666, -2.596402595788921324E-15 ) ) ;
#12630=DIRECTION ( 'NONE',  ( 0.000000000000000000, 0.000000000000000000, 1.000000000000000000 ) ) ;
#12632=CARTESIAN_POINT ( 'NONE',  ( -12.99553232110414136, 58.19864449459907974, -1.797034655631248355E-15 ) ) ;
#12633=ADVANCED_FACE ( 'NONE', ( #1841 ), #4006, .F. ) ;
#12634=CARTESIAN_POINT ( 'NONE',  ( -0.07087239851500722054, -158.6804527307045873, 1.494076624346223792 ) ) ;
#12635=CARTESIAN_POINT ( 'NONE',  ( 15.29705854078139282, 47.94714734142005597, -30.59411708156277498 ) ) ;
#12638=CARTESIAN_POINT ( 'NONE',  ( -12.99553232110414847, -7.774801155466916747, 25.99106464220827917 ) ) ;
#12642=ORIENTED_EDGE ( 'NONE', *, *, #1064, .T. ) ;
#12644=CARTESIAN_POINT ( 'NONE',  ( 10.69346802281035025, 77.87317997377837742, -21.38693604562069339 ) ) ;
#12645=VERTEX_POINT ( 'NONE', #10462 ) ;
#12648=CARTESIAN_POINT ( 'NONE',  ( -0.6173387890061912131, -70.00000000000000000, 4.961742921553712549 ) ) ;
#12651=ADVANCED_FACE ( 'NONE', ( #7361 ), #13590, .T. ) ;
#12653=CARTESIAN_POINT ( 'NONE',  ( -1.181099040078819939, -130.2509440800175469, 3.835336864914359101 ) ) ;
#12656=EDGE_LOOP ( 'NONE', ( #3813, #8578, #3684, #2106 ) ) ;
#12658=ORIENTED_EDGE ( 'NONE', *, *, #6436, .F. ) ;
#12659=CARTESIAN_POINT ( 'NONE',  ( -25.00000000000000355, 120.0000000000000284, 0.5000000000000000000 ) ) ;
#12660=CARTESIAN_POINT ( 'NONE',  ( 2.715127098185230459, -81.24690994262827815, -9.545145086786032351 ) ) ;
#12663=CARTESIAN_POINT ( 'NONE',  ( 12.99579180576517246, 64.08350967699263379, -25.99158361153033425 ) ) ;
#12667=DIRECTION ( 'NONE',  ( -1.000000000000000000, 0.000000000000000000, 0.000000000000000000 ) ) ;
#12669=CYLINDRICAL_SURFACE ( 'NONE', #5920, 8.385254915620292238 ) ;
#12674=ORIENTED_EDGE ( 'NONE', *, *, #9583, .F. ) ;
#12675=CARTESIAN_POINT ( 'NONE',  ( 10.69381717166375267, -12.13966492792242846, 21.38763434332751601 ) ) ;
#12676=ORIENTED_EDGE ( 'NONE', *, *, #4296, .T. ) ;
#12680=CARTESIAN_POINT ( 'NONE',  ( 11.42522452384381459, -72.18181818184932297, 3.860454353695761842 ) ) ;
#12681=DIRECTION ( 'NONE',  ( 1.000000000000000000, 6.530723674265631117E-15, 0.000000000000000000 ) ) ;
#12682=CARTESIAN_POINT ( 'NONE',  ( -8.385254915620292238, -22.36966495935058319, 16.77050983124057737 ) ) ;
#12683=VECTOR ( 'NONE', #6818, 1000.000000000000000 ) ;
#12684=DIRECTION ( 'NONE',  ( -1.000000000000000000, 0.000000000000000000, 0.000000000000000000 ) ) ;
#12685=CARTESIAN_POINT ( 'NONE',  ( -4.696430422119474812, 90.40949893945196436, 1.719416569030751907 ) ) ;
#12686=ADVANCED_FACE ( 'NONE', ( #1975 ), #11646, .F. ) ;
#12688=CARTESIAN_POINT ( 'NONE',  ( -2.712777076799875786, -81.24515448198224021, 9.546134740491345028 ) ) ;
#12691=CARTESIAN_POINT ( 'NONE',  ( 12.99579180576517246, -11.31471392308272428, -25.99158361153033070 ) ) ;
#12692=CARTESIAN_POINT ( 'NONE',  ( 10.00000000000000711, 139.9999999999999716, -0.5000000000000000000 ) ) ;
#12693=DIRECTION ( 'NONE',  ( 1.000000000000000000, 0.000000000000000000, 0.000000000000000000 ) ) ;
#12695=DIRECTION ( 'NONE',  ( 1.000000000000000000, 0.000000000000000000, 0.000000000000000000 ) ) ;
#12699=EDGE_CURVE ( 'NONE', #12324, #6913, #8358, .T. ) ;
#12700=VERTEX_POINT ( 'NONE', #2823 ) ;
#12706=CARTESIAN_POINT ( 'NONE',  ( -3.163850051431345456, 90.09728930184206774, -3.875191615614280494 ) ) ;
#12709=ORIENTED_EDGE ( 'NONE', *, *, #11312, .F. ) ;
#12710=CARTESIAN_POINT ( 'NONE',  ( 0.9875500501441598633, -80.00464164738322381, -10.06307372056550342 ) ) ;
#12711=PLANE ( 'NONE',  #5791 ) ;
#12712=CARTESIAN_POINT ( 'NONE',  ( -9.883290025451492156, -71.99999999999975842, -4.866269441041104926 ) ) ;
#12715=CARTESIAN_POINT ( 'NONE',  ( -0.5859240664712906943, -103.8004541631269291, -7.169336856130571256 ) ) ;
#12716=DIRECTION ( 'NONE',  ( -0.000000000000000000, -0.000000000000000000, -1.000000000000000000 ) ) ;
#12720=ORIENTED_EDGE ( 'NONE', *, *, #6436, .T. ) ;
#12721=DIRECTION ( 'NONE',  ( -1.000000000000000000, 0.000000000000000000, 0.000000000000000000 ) ) ;
#12723=CARTESIAN_POINT ( 'NONE',  ( 12.99553232110413781, 39.34908859458022334, 3.182987412051230984E-15 ) ) ;
#12725=CARTESIAN_POINT ( 'NONE',  ( -6.124978294105043908, -112.7307712075077006, -0.3410559919339725132 ) ) ;
#12727=DIRECTION ( 'NONE',  ( -1.000000000000000000, 0.000000000000000000, 0.000000000000000000 ) ) ;
#12728=FACE_OUTER_BOUND ( 'NONE', #9606, .T. ) ;
#12729=CARTESIAN_POINT ( 'NONE',  ( -15.29705854078138927, 0.8232575913729157646, -30.59411708156278564 ) ) ;
#12730=CARTESIAN_POINT ( 'NONE',  ( 35.20000000000002416, 106.4000000000000199, 0.5000000000000000000 ) ) ;
#12732=DIRECTION ( 'NONE',  ( -2.797435172181481150E-17, 1.000000000000000000, -1.765856845898762549E-18 ) ) ;
#12733=DIRECTION ( 'NONE',  ( 1.000000000000000000, 0.000000000000000000, 0.000000000000000000 ) ) ;
#12734=CARTESIAN_POINT ( 'NONE',  ( -11.42522452383575526, -72.18181818187404986, -3.860454353694361629 ) ) ;
#12737=FACE_OUTER_BOUND ( 'NONE', #10909, .T. ) ;
#12739=CARTESIAN_POINT ( 'NONE',  ( 15.29705854078139105, -10.48808792804187284, 1.890204135573039875E-15 ) ) ;
#12740=CARTESIAN_POINT ( 'NONE',  ( -25.00000000000000355, 120.0000000000000284, -2.500000000000000000 ) ) ;
#12742=CARTESIAN_POINT ( 'NONE',  ( -5.138450363093652662, -111.7272727272696642, 0.006098328147121623993 ) ) ;
#12743=CIRCLE ( 'NONE', #1529, 15.29705854078139105 ) ;
#12745=DIRECTION ( 'NONE',  ( 1.000000000000000000, 0.000000000000000000, 0.000000000000000000 ) ) ;
#12746=CARTESIAN_POINT ( 'NONE',  ( 2.933974605883639275E-16, -10.48808792804187284, 1.852046186812095429E-17 ) ) ;
#12747=DIRECTION ( 'NONE',  ( -1.000000000000000000, 0.000000000000000000, 0.000000000000000000 ) ) ;
#12749=CIRCLE ( 'NONE', #6687, 8.385254915620292238 ) ;
#12753=CARTESIAN_POINT ( 'NONE',  ( 8.385254915620290461, 43.60378069071538221, 9.813990265092201964E-16 ) ) ;
#12754=CARTESIAN_POINT ( 'NONE',  ( -8.385254915620297567, 69.25350232273815720, 16.77050983124058448 ) ) ;
#12755=EDGE_CURVE ( 'NONE', #4358, #11837, #7289, .T. ) ;
#12759=CARTESIAN_POINT ( 'NONE',  ( -8.827136188495221389E-16, 31.55439052270045508, -5.572053652267360357E-17 ) ) ;
#12762=DIRECTION ( 'NONE',  ( 1.000000000000000000, 0.000000000000000000, 0.000000000000000000 ) ) ;
#12767=AXIS2_PLACEMENT_3D ( 'NONE', #2906, #1988, #10471 ) ;
#12768=AXIS2_PLACEMENT_3D ( 'NONE', #5647, #9930, #7897 ) ;
#12769=CARTESIAN_POINT ( 'NONE',  ( -3.828914887500469266, 90.45818551217382719, -3.218881588266133686 ) ) ;
#12771=ORIENTED_EDGE ( 'NONE', *, *, #11919, .F. ) ;
#12773=CARTESIAN_POINT ( 'NONE',  ( 8.385254915620295790, 78.67828027274755698, -16.77050983124058803 ) ) ;
#12778=EDGE_CURVE ( 'NONE', #8282, #10214, #3466, .T. ) ;
#12781=CARTESIAN_POINT ( 'NONE',  ( -10.69346802281034847, 68.44840202376897764, -2.779593060601867454E-15 ) ) ;
#12783=CARTESIAN_POINT ( 'NONE',  ( -2.891665148108589545, -140.3705018960054929, 0.05415431998640414524 ) ) ;
#12786=AXIS2_PLACEMENT_3D ( 'NONE', #8388, #4171, #12681 ) ;
#12792=AXIS2_PLACEMENT_3D ( 'NONE', #11599, #3106, #3174 ) ;
#12793=CARTESIAN_POINT ( 'NONE',  ( -12.99553232110412893, 39.34908859458022334, -25.99106464220826851 ) ) ;
#12794=CARTESIAN_POINT ( 'NONE',  ( 8.641831928493635573, -88.07519045024412208, -2.946015976100306855 ) ) ;
#12797=CARTESIAN_POINT ( 'NONE',  ( -10.69381717166375090, 6.709890972096425266, -21.38763434332751245 ) ) ;
#12798=B_SPLINE_CURVE_WITH_KNOTS ( 'NONE', 3,
 ( #5525, #78, #3420, #10847, #4271, #1260, #6450, #6521, #10714, #13064, #9812, #4332, #8615, #7560, #10779, #1194, #4474, #5676, #5897, #9119, #641, #3783, #12274, #8978, #11288, #3634, #12350, #13209 ),
 .UNSPECIFIED., .F., .F.,
 ( 4, 2, 2, 2, 2, 2, 2, 2, 2, 2, 2, 2, 2, 4 ),
 ( 1.917168677021176670E-17, 0.002162634761238544073, 0.003243952141857817627, 0.004325269522477092482, 0.006487904283715641325, 0.008650539044954190168, 0.009731856425573476299, 0.01081317380619276416, 0.01189449118681205030, 0.01297580856743134163, 0.01513844332866991910, 0.01621976070928919655, 0.01676041939959882487, 0.01730107808990844973 ),
 .UNSPECIFIED. ) ;
#12800=DIRECTION ( 'NONE',  ( -1.000000000000000000, -2.835060530349835421E-17, 0.000000000000000000 ) ) ;
#12802=CARTESIAN_POINT ( 'NONE',  ( -1.623329383841033646, -80.00119987276727329, -9.930725418093544477 ) ) ;
#12803=CARTESIAN_POINT ( 'NONE',  ( -1.673669778670227307E-15, 59.82872437272870769, -1.056489625149731375E-16 ) ) ;
#12804=DIRECTION ( 'NONE',  ( -2.797435172181481150E-17, 1.000000000000000000, -1.765856845898762549E-18 ) ) ;
#12806=ADVANCED_FACE ( 'NONE', ( #5461 ), #9747, .T. ) ;
#12811=VECTOR ( 'NONE', #6871, 1000.000000000000000 ) ;
#12812=CIRCLE ( 'NONE', #715, 5.000000000000000000 ) ;
#12813=CARTESIAN_POINT ( 'NONE',  ( -10.69381717166375623, 72.68333662216238622, -2.782997899970468246E-15 ) ) ;
#12815=CARTESIAN_POINT ( 'NONE',  ( 6.296481028488151388, -65.63636363857402500, 1.027962039518596882 ) ) ;
#12818=ORIENTED_EDGE ( 'NONE', *, *, #3795, .F. ) ;
#12821=CARTESIAN_POINT ( 'NONE',  ( -1.553027081867818682, -81.93939393924890169, 9.741774319753540468 ) ) ;
#12822=EDGE_CURVE ( 'NONE', #11499, #10921, #11441, .T. ) ;
#12825=DIRECTION ( 'NONE',  ( -2.797435172181481150E-17, 1.000000000000000000, -1.765856845898762549E-18 ) ) ;
#12826=CARTESIAN_POINT ( 'NONE',  ( 12.99553232110413958, 11.07475474455194053, 1.577534959232427603E-15 ) ) ;
#12831=ORIENTED_EDGE ( 'NONE', *, *, #114, .F. ) ;
#12832=( BOUNDED_SURFACE ( )  B_SPLINE_SURFACE ( 3, 3, ( 
 ( #6104, #2869, #12562, #4182 ),
 ( #11693, #6235, #8268, #1047 ),
 ( #10441, #1815, #2086, #8203 ),
 ( #2020, #5241, #10637, #6367 ) ),
 .UNSPECIFIED., .F., .F., .F. ) 
 B_SPLINE_SURFACE_WITH_KNOTS ( ( 4, 4 ),
 ( 4, 4 ),
 ( 0.000000000000000000, 1.000000000000000000 ),
 ( 0.000000000000000000, 1.000000000000000000 ),
 .UNSPECIFIED. ) 
 GEOMETRIC_REPRESENTATION_ITEM ( )  RATIONAL_B_SPLINE_SURFACE ( (
 ( 1.000000000000000000, 0.3333333333333334259, 0.3333333333333334259, 1.000000000000000000),
 ( 1.000000000000000000, 0.3333333333333334259, 0.3333333333333334259, 1.000000000000000000),
 ( 1.000000000000000000, 0.3333333333333334259, 0.3333333333333334259, 1.000000000000000000),
 ( 1.000000000000000000, 0.3333333333333334259, 0.3333333333333334259, 1.000000000000000000) ) ) 
 REPRESENTATION_ITEM ( '' )  SURFACE ( )  );
#12833=CIRCLE ( 'NONE', #7203, 40.00000000000001421 ) ;
#12839=CARTESIAN_POINT ( 'NONE',  ( -3.989522564198866306, -78.56682798443820559, -9.305603802367686583 ) ) ;
#12840=CARTESIAN_POINT ( 'NONE',  ( 0.5328336654596128596, -153.1537951631405576, 1.636456857774888807 ) ) ;
#12845=VERTEX_POINT ( 'NONE', #8619 ) ;
#12847=LINE ( 'NONE', #5320, #2705 ) ;
#12848=EDGE_LOOP ( 'NONE', ( #6200, #3315, #7507 ) ) ;
#12849=CARTESIAN_POINT ( 'NONE',  ( 8.385254915620288685, 71.87811454074363837, 2.053795118489799215E-15 ) ) ;
#12854=CARTESIAN_POINT ( 'NONE',  ( -12.99553232110413958, 67.62342244460847951, -3.323022390375262386E-15 ) ) ;
#12856=CARTESIAN_POINT ( 'NONE',  ( -3.876523907412873449, -100.4503140241744461, -6.538907747273460913 ) ) ;
#12859=ORIENTED_EDGE ( 'NONE', *, *, #3984, .T. ) ;
#12860=EDGE_LOOP ( 'NONE', ( #5349, #11299, #3935, #11715, #3844, #4369 ) ) ;
#12865=ORIENTED_EDGE ( 'NONE', *, *, #10557, .F. ) ;
#12866=CARTESIAN_POINT ( 'NONE',  ( 10.69381717166375090, -2.714886977913000266, 21.38763434332751245 ) ) ;
#12868=CARTESIAN_POINT ( 'NONE',  ( -6.244934989200983111, -111.0871311010834006, 1.123163629316296541 ) ) ;
#12870=CARTESIAN_POINT ( 'NONE',  ( -2.739930038171048743, -137.4545454545128678, -2.373837707219439874 ) ) ;
#12873=CARTESIAN_POINT ( 'NONE',  ( -9.082088619475678470, -71.90909090908878909, -4.345719731624131832 ) ) ;
#12874=CARTESIAN_POINT ( 'NONE',  ( -35.20000000000000995, 106.4000000000000199, -2.500000000000000000 ) ) ;
#12877=CARTESIAN_POINT ( 'NONE',  ( -38.79999999999999716, 101.5999999999999943, -2.500000000000000000 ) ) ;
#12880=ADVANCED_FACE ( 'NONE', ( #11913 ), #8194, .T. ) ;
#12883=LINE ( 'NONE', #11541, #7062 ) ;
#12888=ORIENTED_EDGE ( 'NONE', *, *, #5341, .T. ) ;
#12890=FACE_OUTER_BOUND ( 'NONE', #8069, .T. ) ;
#12891=DIRECTION ( 'NONE',  ( -1.000000000000000000, 0.000000000000000000, 0.000000000000000000 ) ) ;
#12894=CARTESIAN_POINT ( 'NONE',  ( 8.385254915620288685, 34.17900274070598243, 9.688596779957292534E-16 ) ) ;
#12895=DIRECTION ( 'NONE',  ( 1.000000000000000000, 0.000000000000000000, 0.000000000000000000 ) ) ;
#12896=CARTESIAN_POINT ( 'NONE',  ( 0.6173387890061909911, 79.99058638175036151, -4.961742921553712549 ) ) ;
#12897=DIRECTION ( 'NONE',  ( -2.797435172181481150E-17, 1.000000000000000000, -1.765856845898762549E-18 ) ) ;
#12903=CARTESIAN_POINT ( 'NONE',  ( 12.99579180576517068, 45.23395377697383424, -25.99158361153033070 ) ) ;
#12908=CARTESIAN_POINT ( 'NONE',  ( -25.00000000000000355, 120.0000000000000284, 0.5000000000000000000 ) ) ;
#12909=AXIS2_PLACEMENT_3D ( 'NONE', #13792, #12716, #10524 ) ;
#12911=DIRECTION ( 'NONE',  ( -2.797435172181481150E-17, 1.000000000000000000, -1.765856845898762549E-18 ) ) ;
#12916=CIRCLE ( 'NONE', #3915, 15.29705854078140170 ) ;
#12917=EDGE_CURVE ( 'NONE', #5877, #7271, #9322, .T. ) ;
#12919=ORIENTED_EDGE ( 'NONE', *, *, #6512, .F. ) ;
#12920=ORIENTED_EDGE ( 'NONE', *, *, #4444, .T. ) ;
#12923=CIRCLE ( 'NONE', #13627, 2.000000000000000000 ) ;
#12924=FACE_OUTER_BOUND ( 'NONE', #8165, .T. ) ;
#12925=CARTESIAN_POINT ( 'NONE',  ( 4.066030946031333748, 90.77438413795609051, -2.912544222229247914 ) ) ;
#12926=CARTESIAN_POINT ( 'NONE',  ( -8.551509863446513648, -93.00797441535850396, -0.1595843423901910085 ) ) ;
#12927=DIRECTION ( 'NONE',  ( 1.000000000000000000, 0.000000000000000000, 0.000000000000000000 ) ) ;
#12931=CARTESIAN_POINT ( 'NONE',  ( -2.517691654963332357E-15, 90.00000000000000000, -1.589271161308885878E-16 ) ) ;
#12932=CARTESIAN_POINT ( 'NONE',  ( -15.29705854078139105, 90.00000000000000000, -1.589271161308885878E-16 ) ) ;
#12933=EDGE_LOOP ( 'NONE', ( #13649, #4207, #8128, #8514 ) ) ;
#12934=CARTESIAN_POINT ( 'NONE',  ( -15.29705854078139282, -1.063309978032445979, -1.869594071425719488E-15 ) ) ;
#12935=CARTESIAN_POINT ( 'NONE',  ( 34.00000000000001421, 108.0000000000000142, -0.5000000000000000000 ) ) ;
#12936=CARTESIAN_POINT ( 'NONE',  ( -8.385254915620294014, 3.280056672672198914, -5.792110530374064999E-18 ) ) ;
#12939=CARTESIAN_POINT ( 'NONE',  ( -0.9052951019203371308, -81.00000000000012790, -10.12030223674820562 ) ) ;
#12940=EDGE_CURVE ( 'NONE', #2529, #6545, #2824, .T. ) ;
#12943=B_SPLINE_CURVE_WITH_KNOTS ( 'NONE', 3,
 ( #2864, #1678, #10498, #4898, #12622, #12688, #5961, #7204, #12554, #2939, #10299, #9248, #9174, #1880, #1743, #6167, #703, #10435, #837, #12411, #5103, #2998, #11555, #7068, #6297, #13290, #5609, #9056, #12140, #8072, #299, #371, #5827, #738, #1495, #1710, #12302, #7950, #3881, #9077, #2694, #9282, #3665, #10261, #12235, #10057, #6893, #2625, #11378, #5996, #6968, #5001, #11252, #6062, #11179, #12440, #13597, #1565, #666, #8095, #5855, #4934, #12381, #10128, #538, #3949, #13393, #13313, #3807, #1637, #10335, #8224, #12513, #13533, #13464, #5922, #4723, #3742, #5775, #6828, #603, #464, #4866, #9214, #8162, #7034, #11105, #8024, #11313, #10196, #2767, #2831, #9007, #9142, #7103, #11522, #803, #7168, #10598, #2050, #3037, #4011, #11652, #11591, #6258, #5269, #9556, #13864, #1493, #2828, #3662, #664, #3877, #11176, #3740, #5994, #12300, #11250, #12156, #10193, #4798, #5773, #2548, #5853 ),
 .UNSPECIFIED., .F., .F.,
 ( 4, 2, 2, 2, 2, 2, 2, 2, 2, 2, 2, 2, 2, 2, 2, 2, 2, 2, 2, 2, 2, 2, 2, 2, 2, 2, 2, 2, 2, 2, 2, 2, 2, 2, 2, 2, 2, 2, 2, 2, 2, 2, 2, 2, 2, 2, 2, 2, 2, 2, 2, 2, 2, 2, 2, 2, 2, 2, 2, 2, 2, 4 ),
 ( 2.912531104258623014E-17, 0.0008227720497348227488, 0.001645544099469616224, 0.003291088198939203392, 0.004936632298408791426, 0.006582176397878378160, 0.008227720497347964027, 0.009050492547082742215, 0.009873264596817522137, 0.01316435279575666265, 0.01480989689522623463, 0.01645544099469580662, 0.01810098509416537688, 0.01892375714390017935, 0.01974652919363497836, 0.02303761739257425070, 0.02468316149204390075, 0.02632870559151355080, 0.02797424969098320433, 0.02961979379045285438, 0.03291088198939215448, 0.03455642608886181494, 0.03620197018833147540, 0.03784751428780114280, 0.03949305838727080326, 0.04278414658621013111, 0.04360691863594496481, 0.04442969068567979851, 0.04607523478514943122, 0.04772077888461906392, 0.04854355093435388374, 0.04936632298408870356, 0.05101186708355830157, 0.05265741118302790652, 0.05594849938196708172, 0.05759404348143667279, 0.05923958758090627774, 0.06088513168037586881, 0.06253067577984547376, 0.06582176397878466978, 0.06746730807825425391, 0.06911285217772385192, 0.07075839627719342217, 0.07240394037666302018, 0.07569502857560218845, 0.07734057267507175870, 0.07898611677454135671, 0.08063166087401094084, 0.08227720497348053885, 0.08556829317241962385, 0.08721383727188916635, 0.08885938137135870885, 0.09050492547082823747, 0.09215046957029777996, 0.09379601366976733634, 0.09544155776923687884, 0.09708710186870640746, 0.09873264596817596384, 0.1020237341671150488, 0.1036692782665845497, 0.1044920503163192654, 0.1053148223660539812 ),
 .UNSPECIFIED. ) ;
#12948=DIRECTION ( 'NONE',  ( -1.000000000000000000, 0.000000000000000000, 0.000000000000000000 ) ) ;
#12952=CARTESIAN_POINT ( 'NONE',  ( -12.99579180576517068, 73.50828762700209040, -1.851135709604445740E-15 ) ) ;
#12953=CARTESIAN_POINT ( 'NONE',  ( 12.99579180576516713, 54.65873172698324112, 1.506871011810438326E-15 ) ) ;
#12955=EDGE_CURVE ( 'NONE', #6325, #1805, #3487, .T. ) ;
#12959=CYLINDRICAL_SURFACE ( 'NONE', #10151, 15.29705854078139105 ) ;
#12960=DIRECTION ( 'NONE',  ( -1.000000000000000000, 0.000000000000000000, 0.000000000000000000 ) ) ;
#12962=CIRCLE ( 'NONE', #5787, 42.00000000000001421 ) ;
#12963=ORIENTED_EDGE ( 'NONE', *, *, #5817, .F. ) ;
#12965=B_SPLINE_CURVE_WITH_KNOTS ( 'NONE', 3,
 ( #13163, #10872, #4360, #398 ),
 .UNSPECIFIED., .F., .F.,
 ( 4, 4 ),
 ( 0.000000000000000000, 1.000000000000000000 ),
 .UNSPECIFIED. ) ;
#12968=CARTESIAN_POINT ( 'NONE',  ( 0.000000000000000000, 71.01020514433645303, 2.500000000000000000 ) ) ;
#12975=EDGE_CURVE ( 'NONE', #13355, #11738, #6826, .T. ) ;
#12978=EDGE_CURVE ( 'NONE', #5587, #11767, #7948, .T. ) ;
#12982=CARTESIAN_POINT ( 'NONE',  ( 10.69381717166375445, 53.83378072214353693, 0.000000000000000000 ) ) ;
#12983=ORIENTED_EDGE ( 'NONE', *, *, #3189, .F. ) ;
#12985=DIRECTION ( 'NONE',  ( 1.000000000000000000, 0.000000000000000000, 0.000000000000000000 ) ) ;
#12986=CARTESIAN_POINT ( 'NONE',  ( -2.132246523607266586E-15, 76.22148119144830503, -1.345962243664627229E-16 ) ) ;
#12990=ORIENTED_EDGE ( 'NONE', *, *, #10621, .T. ) ;
#12992=CIRCLE ( 'NONE', #3561, 8.385254915620292238 ) ;
#12993=EDGE_LOOP ( 'NONE', ( #13747, #5272, #4569, #8472 ) ) ;
#12994=ORIENTED_EDGE ( 'NONE', *, *, #9112, .F. ) ;
#12999=CARTESIAN_POINT ( 'NONE',  ( -1.146365672123090463E-15, 40.97916847270985130, -7.236334518677345233E-17 ) ) ;
#13000=SURFACE_SIDE_STYLE ('',( #8697 ) ) ;
#13001=CARTESIAN_POINT ( 'NONE',  ( -15.29705854078139282, 36.63580182200523438, -2.002736540738517883E-15 ) ) ;
#13002=CARTESIAN_POINT ( 'NONE',  ( -15.29705854078139460, -8.601520358636511432, -3.733175406185929791E-15 ) ) ;
#13005=CARTESIAN_POINT ( 'NONE',  ( -1.483439550716517611E-15, 53.02855864072483882, -9.364084330386787485E-17 ) ) ;
#13006=AXIS2_PLACEMENT_3D ( 'NONE', #9860, #1371, #8956 ) ;
#13007=CARTESIAN_POINT ( 'NONE',  ( -6.150798755069114776, -74.45454545454569484, -8.129532795066724660 ) ) ;
#13008=AXIS2_PLACEMENT_3D ( 'NONE', #3647, #8143, #6945 ) ;
#13010=CYLINDRICAL_SURFACE ( 'NONE', #1202, 8.385254915620292238 ) ;
#13011=VERTEX_POINT ( 'NONE', #12456 ) ;
#13017=CIRCLE ( 'NONE', #6067, 15.29705854078138749 ) ;
#13019=CARTESIAN_POINT ( 'NONE',  ( -2.517691654963332357E-15, 90.00000000000000000, -1.589271161308885878E-16 ) ) ;
#13020=ORIENTED_EDGE ( 'NONE', *, *, #1284, .T. ) ;
#13021=CARTESIAN_POINT ( 'NONE',  ( -4.288313376222440694E-16, 15.32944684068712782, -2.706960864746847057E-17 ) ) ;
#13024=CARTESIAN_POINT ( 'NONE',  ( -12.99553232110414847, 1.649976794542511671, 25.99106464220827917 ) ) ;
#13027=CARTESIAN_POINT ( 'NONE',  ( -15.29705854078139993, -19.91286587805129926, 3.516327053222078456E-17 ) ) ;
#13028=CARTESIAN_POINT ( 'NONE',  ( -8.385254915620290461, 12.70483462268160046, -16.77050983124058803 ) ) ;
#13032=VECTOR ( 'NONE', #4301, 1000.000000000000000 ) ;
#13033=CARTESIAN_POINT ( 'NONE',  ( 31.81818181818183433, 133.3608531424536920, -0.5000000000000000000 ) ) ;
#13037=ADVANCED_FACE ( 'NONE', ( #9496 ), #2730, .T. ) ;
#13039=DIRECTION ( 'NONE',  ( -2.797435172181481150E-17, 1.000000000000000000, -1.765856845898762549E-18 ) ) ;
#13042=VERTEX_POINT ( 'NONE', #6070 ) ;
#13043=DIRECTION ( 'NONE',  ( -2.797435172181481150E-17, 1.000000000000000000, -1.765856845898762549E-18 ) ) ;
#13045=CARTESIAN_POINT ( 'NONE',  ( -1.815818965600183303E-15, 64.91013567203349055, -1.146220074446778111E-16 ) ) ;
#13048=VERTEX_POINT ( 'NONE', #6211 ) ;
#13053=CARTESIAN_POINT ( 'NONE',  ( -10.00000000000000000, 90.00000000000000000, 0.5000000000000000000 ) ) ;
#13054=ADVANCED_FACE ( 'NONE', ( #11531 ), #1923, .T. ) ;
#13057=ORIENTED_EDGE ( 'NONE', *, *, #12536, .T. ) ;
#13059=ORIENTED_EDGE ( 'NONE', *, *, #1706, .T. ) ;
#13061=CARTESIAN_POINT ( 'NONE',  ( -12.99579180576517601, 73.50828762700210461, 25.99158361153033070 ) ) ;
#13064=CARTESIAN_POINT ( 'NONE',  ( -4.711442097700778042, -75.83792215129622605, -8.965827225112430909 ) ) ;
#13066=CARTESIAN_POINT ( 'NONE',  ( 2.179449471770333435, 90.00000000000000000, -4.500000000000000888 ) ) ;
#13067=CARTESIAN_POINT ( 'NONE',  ( -7.108720426521072611, -96.49446529545537032, -3.837650603676977301 ) ) ;
#13069=ORIENTED_EDGE ( 'NONE', *, *, #7625, .F. ) ;
#13072=AXIS2_PLACEMENT_3D ( 'NONE', #11953, #2344, #4590 ) ;
#13075=DIRECTION ( 'NONE',  ( -0.000000000000000000, -0.000000000000000000, -1.000000000000000000 ) ) ;
#13076=ORIENTED_EDGE ( 'NONE', *, *, #7270, .F. ) ;
#13081=CARTESIAN_POINT ( 'NONE',  ( -8.385254915620288685, 5.904668890677672088, -16.77050983124058448 ) ) ;
#13083=CARTESIAN_POINT ( 'NONE',  ( 2.491129965231927645, -148.3982683980968034, -1.520867222960365472 ) ) ;
#13085=CARTESIAN_POINT ( 'NONE',  ( -1.238635481694431384, -80.00117812811808449, -9.950197937997891984 ) ) ;
#13087=CARTESIAN_POINT ( 'NONE',  ( -2.197875741315214793, -79.21212121212059287, -9.798460318839479655 ) ) ;
#13090=EDGE_LOOP ( 'NONE', ( #4655, #12108, #4646, #13458 ) ) ;
#13092=DIRECTION ( 'NONE',  ( -1.000000000000000000, 0.000000000000000000, 0.000000000000000000 ) ) ;
#13093=CARTESIAN_POINT ( 'NONE',  ( -8.385254915620286909, 71.87811454074363837, -16.77050983124057737 ) ) ;
#13096=DIRECTION ( 'NONE',  ( -2.797435172181479917E-17, 1.000000000000000000, -1.765856845898779112E-18 ) ) ;
#13098=DIRECTION ( 'NONE',  ( -1.000000000000000000, 0.000000000000000000, 0.000000000000000000 ) ) ;
#13100=CARTESIAN_POINT ( 'NONE',  ( 8.385254915620290461, 24.75422479069652937, 16.77050983124058803 ) ) ;
#13101=DIRECTION ( 'NONE',  ( 0.000000000000000000, 0.000000000000000000, 1.000000000000000000 ) ) ;
#13102=CARTESIAN_POINT ( 'NONE',  ( -2.517691654963332357E-15, 90.00000000000000000, -1.589271161308885878E-16 ) ) ;
#13103=DIRECTION ( 'NONE',  ( 0.000000000000000000, 0.000000000000000000, 1.000000000000000000 ) ) ;
#13104=DIRECTION ( 'NONE',  ( -1.000000000000000000, 0.000000000000000000, 0.000000000000000000 ) ) ;
#13107=ORIENTED_EDGE ( 'NONE', *, *, #10054, .F. ) ;
#13110=CARTESIAN_POINT ( 'NONE',  ( 10.00000000000000711, 139.9999999999999716, 0.5000000000000000000 ) ) ;
#13115=EDGE_CURVE ( 'NONE', #12645, #2744, #1274, .T. ) ;
#13116=CARTESIAN_POINT ( 'NONE',  ( -2.517691654963332357E-15, 90.00000000000000000, -1.589271161308885878E-16 ) ) ;
#13119=CARTESIAN_POINT ( 'NONE',  ( -12.99553232110413781, -26.62435705548576692, -25.99106464220828627 ) ) ;
#13120=VECTOR ( 'NONE', #2128, 1000.000000000000000 ) ;
#13127=CYLINDRICAL_SURFACE ( 'NONE', #4897, 14.99999999999999112 ) ;
#13128=CARTESIAN_POINT ( 'NONE',  ( -38.79999999999999716, 101.5999999999999943, 2.500000000000000000 ) ) ;
#13130=CARTESIAN_POINT ( 'NONE',  ( 4.330127018922190985, 92.00000000000000000, -2.500000000000000000 ) ) ;
#13131=EDGE_CURVE ( 'NONE', #12240, #4671, #8432, .T. ) ;
#13132=CARTESIAN_POINT ( 'NONE',  ( -12.99579180576516713, -30.16426982310158422, -25.99158361153034491 ) ) ;
#13133=ADVANCED_FACE ( 'NONE', ( #8504 ), #3388, .F. ) ;
#13143=CARTESIAN_POINT ( 'NONE',  ( -8.385254915620292238, 5.904668890677672088, -1.042679998336861873E-17 ) ) ;
#13145=ORIENTED_EDGE ( 'NONE', *, *, #10458, .F. ) ;
#13146=CARTESIAN_POINT ( 'NONE',  ( -12.99579180576517068, -1.889935973073298747, 25.99158361153033070 ) ) ;
#13149=CARTESIAN_POINT ( 'NONE',  ( -8.385254915620292238, 34.17900274070598243, 16.77050983124057382 ) ) ;
#13151=CARTESIAN_POINT ( 'NONE',  ( -0.5797347049570008570, -122.9090909090927113, 5.796875383663884662 ) ) ;
#13153=CARTESIAN_POINT ( 'NONE',  ( -0.09220535797252617238, -163.8787878627269095, 3.538661136716170219 ) ) ;
#13154=CARTESIAN_POINT ( 'NONE',  ( -11.81226048336476708, -40.00941361824963849, -1.520867253700650540E-15 ) ) ;
#13156=ADVANCED_FACE ( 'NONE', ( #689, #3761 ), #1733, .T. ) ;
#13162=EDGE_CURVE ( 'NONE', #5237, #13265, #9434, .T. ) ;
#13163=CARTESIAN_POINT ( 'NONE',  ( 8.385254915620294014, 3.280056672672199358, 1.018788103988028997E-15 ) ) ;
#13171=CARTESIAN_POINT ( 'NONE',  ( 15.29705854078138749, 10.24803554138234496, 1.856918518244839783E-15 ) ) ;
#13172=ORIENTED_EDGE ( 'NONE', *, *, #9008, .T. ) ;
#13174=CARTESIAN_POINT ( 'NONE',  ( -2.517691654963332357E-15, 90.00000000000000000, -1.589271161308885878E-16 ) ) ;
#13177=DIRECTION ( 'NONE',  ( -2.797435172181481150E-17, 1.000000000000000000, -1.765856845898762549E-18 ) ) ;
#13180=CARTESIAN_POINT ( 'NONE',  ( -15.29705854078138927, 66.79670324143890525, -1.179534157023628988E-16 ) ) ;
#13182=CARTESIAN_POINT ( 'NONE',  ( -10.04421448780857062, -71.03329039521169364, -1.233851563443314925 ) ) ;
#13183=CARTESIAN_POINT ( 'NONE',  ( -8.385254915620295790, -31.79444290936001494, 16.77050983124058803 ) ) ;
#13188=EDGE_LOOP ( 'NONE', ( #5448, #6869, #8196, #8335 ) ) ;
#13201=ORIENTED_EDGE ( 'NONE', *, *, #13614, .T. ) ;
#13202=VECTOR ( 'NONE', #3418, 1000.000000000000000 ) ;
#13203=CARTESIAN_POINT ( 'NONE',  ( -15.29705854078139460, -27.45107625865536605, -3.726038954167064142E-15 ) ) ;
#13208=CARTESIAN_POINT ( 'NONE',  ( -12.99553232110414136, 77.04820039461787928, -1.863605890287647356E-15 ) ) ;
#13209=CARTESIAN_POINT ( 'NONE',  ( -9.736331930512843513, -69.99978782402621391, -2.722951059031194276 ) ) ;
#13217=AXIS2_PLACEMENT_3D ( 'NONE', #3912, #8192, #12475 ) ;
#13218=EDGE_CURVE ( 'NONE', #11359, #1146, #13416, .T. ) ;
#13219=CARTESIAN_POINT ( 'NONE',  ( -10.69346802281034847, -25.79937747632526879, 21.38693604562068984 ) ) ;
#13220=AXIS2_PLACEMENT_3D ( 'NONE', #4737, #1577, #9016 ) ;
#13222=CARTESIAN_POINT ( 'NONE',  ( 9.997547090296855288, -68.99999999999997158, 0.6397344882394334631 ) ) ;
#13224=CYLINDRICAL_SURFACE ( 'NONE', #2778, 15.29705854078139993 ) ;
#13225=CARTESIAN_POINT ( 'NONE',  ( 15.29705854078139105, -36.87585420866476227, 1.940132561565339224E-15 ) ) ;
#13226=CARTESIAN_POINT ( 'NONE',  ( -8.385254915620292238, 43.60378069071538221, -7.699803463976802609E-17 ) ) ;
#13227=DIRECTION ( 'NONE',  ( -1.000000000000000000, 0.000000000000000000, 0.000000000000000000 ) ) ;
#13228=CARTESIAN_POINT ( 'NONE',  ( 8.597717047226394627, -85.78354978353216609, -6.129448613119037326 ) ) ;
#13231=CARTESIAN_POINT ( 'NONE',  ( 4.974937185533097050, 90.00000000000000000, -0.5000000000000000000 ) ) ;
#13236=ORIENTED_EDGE ( 'NONE', *, *, #12441, .T. ) ;
#13243=EDGE_CURVE ( 'NONE', #3719, #12240, #8637, .T. ) ;
#13244=LINE ( 'NONE', #250, #11216 ) ;
#13245=DIRECTION ( 'NONE',  ( 0.8907235428302473501, -0.4545454545454531425, 0.000000000000000000 ) ) ;
#13247=EDGE_CURVE ( 'NONE', #4278, #2799, #147, .T. ) ;
#13250=CARTESIAN_POINT ( 'NONE',  ( 4.330127018922190985, 92.00000000000000000, -2.500000000000000000 ) ) ;
#13251=CARTESIAN_POINT ( 'NONE',  ( -15.29705854078139282, 46.06057977201469100, -3.826369441655158758E-15 ) ) ;
#13252=EDGE_CURVE ( 'NONE', #430, #10377, #12916, .T. ) ;
#13256=CARTESIAN_POINT ( 'NONE',  ( -0.6173387890061953209, 90.00000000000000000, 4.961742921553712549 ) ) ;
#13257=CARTESIAN_POINT ( 'NONE',  ( -8.235865139535142987, -74.54711635784300938, -5.866162687843151424 ) ) ;
#13262=VECTOR ( 'NONE', #2411, 1000.000000000000000 ) ;
#13264=CARTESIAN_POINT ( 'NONE',  ( -5.503342039658565452E-16, 19.67281349139174296, -3.473937238186366113E-17 ) ) ;
#13265=VERTEX_POINT ( 'NONE', #12401 ) ;
#13268=EDGE_LOOP ( 'NONE', ( #5958, #4779, #6180, #10355, #8690 ) ) ;
#13272=CARTESIAN_POINT ( 'NONE',  ( 15.29705854078138927, 36.63580182200523438, 1.806990092252540434E-15 ) ) ;
#13277=CARTESIAN_POINT ( 'NONE',  ( 8.385254915620288685, 22.12961257269105531, 16.77050983124058448 ) ) ;
#13279=ORIENTED_EDGE ( 'NONE', *, *, #1064, .F. ) ;
#13280=AXIS2_PLACEMENT_3D ( 'NONE', #6266, #6209, #2184 ) ;
#13283=CARTESIAN_POINT ( 'NONE',  ( 12.99553232110412893, 77.04820039461787928, 25.99106464220827561 ) ) ;
#13285=CIRCLE ( 'NONE', #6096, 8.385254915620295790 ) ;
#13287=CARTESIAN_POINT ( 'NONE',  ( -0.4532106388231725846, -104.8728397088437134, 7.045281447031682909 ) ) ;
#13288=CARTESIAN_POINT ( 'NONE',  ( -12.99579180576516002, 16.95961992694555676, -25.99158361153033070 ) ) ;
#13290=CARTESIAN_POINT ( 'NONE',  ( -8.751592884076366374, -90.91481115778101696, -0.6498984818527145935 ) ) ;
#13291=CARTESIAN_POINT ( 'NONE',  ( 10.69346802281034314, -6.949821576306441706, 21.38693604562069694 ) ) ;
#13293=EDGE_LOOP ( 'NONE', ( #5863, #7223, #937, #10578 ) ) ;
#13296=CARTESIAN_POINT ( 'NONE',  ( 10.14773761995948753, -69.33333333333402493, -0.3621078539016990283 ) ) ;
#13297=ORIENTED_EDGE ( 'NONE', *, *, #3242, .T. ) ;
#13298=DIRECTION ( 'NONE',  ( 1.000000000000000000, 0.000000000000000000, 0.000000000000000000 ) ) ;
#13299=CARTESIAN_POINT ( 'NONE',  ( -10.00000000000000711, 139.9999999999999716, 2.500000000000000000 ) ) ;
#13300=CARTESIAN_POINT ( 'NONE',  ( 12.99553232110414314, -36.04913500549519512, 0.000000000000000000 ) ) ;
#13301=DIRECTION ( 'NONE',  ( 1.000000000000000000, 0.000000000000000000, 0.000000000000000000 ) ) ;
#13303=CARTESIAN_POINT ( 'NONE',  ( 1.553027081813024735, -81.93939393942123672, -9.741774319690060580 ) ) ;
#13312=ORIENTED_EDGE ( 'NONE', *, *, #4364, .F. ) ;
#13313=CARTESIAN_POINT ( 'NONE',  ( 5.365047425320059737, -115.1629361961574318, 2.316356917355964384 ) ) ;
#13314=B_SPLINE_CURVE_WITH_KNOTS ( 'NONE', 3,
 ( #4662, #9786, #2340, #12894 ),
 .UNSPECIFIED., .F., .F.,
 ( 4, 4 ),
 ( 0.000000000000000000, 1.000000000000000000 ),
 .UNSPECIFIED. ) ;
#13315=CARTESIAN_POINT ( 'NONE',  ( -4.330127018922195425, 92.00000000000000000, -2.500000000000000000 ) ) ;
#13317=DIRECTION ( 'NONE',  ( 1.000000000000000000, 0.000000000000000000, 0.000000000000000000 ) ) ;
#13320=CARTESIAN_POINT ( 'NONE',  ( 10.69381717166375800, -12.13966492792242846, 0.000000000000000000 ) ) ;
#13322=CARTESIAN_POINT ( 'NONE',  ( -1.386339613915927416, -154.8029363165078962, -0.8714183873244492062 ) ) ;
#13323=DIRECTION ( 'NONE',  ( -1.000000000000000000, 0.000000000000000000, 0.000000000000000000 ) ) ;
#13330=( BOUNDED_SURFACE ( )  B_SPLINE_SURFACE ( 3, 3, ( 
 ( #2583, #6862, #11138, #5809 ),
 ( #13352, #3699, #12263, #2650 ),
 ( #6921, #1603, #6093, #10431 ),
 ( #6293, #7134, #4110, #8392 ) ),
 .UNSPECIFIED., .F., .F., .T. ) 
 B_SPLINE_SURFACE_WITH_KNOTS ( ( 4, 4 ),
 ( 4, 4 ),
 ( 0.000000000000000000, 1.000000000000000000 ),
 ( 0.000000000000000000, 1.000000000000000000 ),
 .UNSPECIFIED. ) 
 GEOMETRIC_REPRESENTATION_ITEM ( )  RATIONAL_B_SPLINE_SURFACE ( (
 ( 1.000000000000000000, 0.3333333333333334259, 0.3333333333333334259, 1.000000000000000000),
 ( 1.000000000000000000, 0.3333333333333334259, 0.3333333333333334259, 1.000000000000000000),
 ( 1.000000000000000000, 0.3333333333333334259, 0.3333333333333334259, 1.000000000000000000),
 ( 1.000000000000000000, 0.3333333333333334259, 0.3333333333333334259, 1.000000000000000000) ) ) 
 REPRESENTATION_ITEM ( '' )  SURFACE ( )  );
#13331=CARTESIAN_POINT ( 'NONE',  ( 8.385254915620294014, -24.99427717735608212, 1.068716529980328543E-15 ) ) ;
#13336=EDGE_CURVE ( 'NONE', #10177, #5287, #7074, .T. ) ;
#13338=CARTESIAN_POINT ( 'NONE',  ( 11.72298137502706439, -61.00000000000002842, 2.970135970080976850 ) ) ;
#13340=ADVANCED_FACE ( 'NONE', ( #9708 ), #11533, .T. ) ;
#13345=ORIENTED_EDGE ( 'NONE', *, *, #1444, .F. ) ;
#13346=CARTESIAN_POINT ( 'NONE',  ( -14.14432607165394629, -111.7272727272741264, 3.395498375151935200 ) ) ;
#13347=AXIS2_PLACEMENT_3D ( 'NONE', #8738, #13043, #3471 ) ;
#13348=CARTESIAN_POINT ( 'NONE',  ( -12.99579180576516535, 7.534841976936128560, -1.618136388307047266E-15 ) ) ;
#13349=CARTESIAN_POINT ( 'NONE',  ( -15.29705854078139993, -19.91286587805129926, -1.803022836769320882E-15 ) ) ;
#13350=CARTESIAN_POINT ( 'NONE',  ( -10.69346802281034670, -35.22415542633469698, -1.185170506590736236E-15 ) ) ;
#13352=CARTESIAN_POINT ( 'NONE',  ( -14.13596196814457429, -39.17949320881311337, -1.592785305112443692E-15 ) ) ;
#13355=VERTEX_POINT ( 'NONE', #9447 ) ;
#13356=ORIENTED_EDGE ( 'NONE', *, *, #9951, .T. ) ;
#13360=CARTESIAN_POINT ( 'NONE',  ( 15.29705854078139282, -36.87585420866476937, -30.59411708156276788 ) ) ;
#13361=CARTESIAN_POINT ( 'NONE',  ( -15.29705854078139282, 90.00000000000000000, -1.589271161308885878E-16 ) ) ;
#13365=CARTESIAN_POINT ( 'NONE',  ( -1.861383205662802354, -106.4032560435130534, 6.615796263637743202 ) ) ;
#13366=CARTESIAN_POINT ( 'NONE',  ( -8.385254915620295790, -6.144721277337255927, 1.085069813372578838E-17 ) ) ;
#13368=EDGE_LOOP ( 'NONE', ( #6348, #6573, #9, #7002 ) ) ;
#13372=CIRCLE ( 'NONE', #3465, 22.99999999999999289 ) ;
#13375=CARTESIAN_POINT ( 'NONE',  ( 6.967039245478349407, -74.45454545454340689, 7.244513656184971673 ) ) ;
#13376=ORIENTED_EDGE ( 'NONE', *, *, #4903, .F. ) ;
#13379=DIRECTION ( 'NONE',  ( -2.797435172181481150E-17, 1.000000000000000000, -1.765856845898762549E-18 ) ) ;
#13380=CARTESIAN_POINT ( 'NONE',  ( 0.7374174230186665291, -122.9090909090850658, 5.357146445002347157 ) ) ;
#13381=CARTESIAN_POINT ( 'NONE',  ( 15.29705854078138394, 46.06057977201469100, 30.59411708156277854 ) ) ;
#13384=CARTESIAN_POINT ( 'NONE',  ( -2.401759516268851424, -79.03030303026447712, -10.21173794902991361 ) ) ;
#13385=CARTESIAN_POINT ( 'NONE',  ( 15.29705854078139282, -1.063309978032472403, 1.873561326908939435E-15 ) ) ;
#13388=CARTESIAN_POINT ( 'NONE',  ( 0.000000000000000000, 71.01020514433645303, -2.500000000000000000 ) ) ;
#13391=DIRECTION ( 'NONE',  ( -0.5999999999999989786, -0.8000000000000008216, 0.000000000000000000 ) ) ;
#13393=CARTESIAN_POINT ( 'NONE',  ( 5.805747447557420671, -113.9141079195865842, 1.331989755664621633 ) ) ;
#13397=DIRECTION ( 'NONE',  ( 0.000000000000000000, 0.000000000000000000, 1.000000000000000000 ) ) ;
#13402=CARTESIAN_POINT ( 'NONE',  ( 3.426743173711812140, -134.8377289227223628, 0.6876845586499595875 ) ) ;
#13405=DIRECTION ( 'NONE',  ( -1.000000000000000000, 0.000000000000000000, 0.000000000000000000 ) ) ;
#13408=CARTESIAN_POINT ( 'NONE',  ( 35.45454545454547457, 140.4866414850956744, 2.500000000000000000 ) ) ;
#13409=CARTESIAN_POINT ( 'NONE',  ( -8.385254915620292238, 62.45333659073423860, -1.247464863180835154E-15 ) ) ;
#13411=ORIENTED_EDGE ( 'NONE', *, *, #1987, .T. ) ;
#13412=CARTESIAN_POINT ( 'NONE',  ( 5.581994045268376503, -105.1818181818169364, -11.80851735648759160 ) ) ;
#13415=EDGE_LOOP ( 'NONE', ( #8136, #2296, #741, #13778 ) ) ;
#13416=LINE ( 'NONE', #8247, #5035 ) ;
#13417=DIRECTION ( 'NONE',  ( -2.797435172181481150E-17, 1.000000000000000000, -1.765856845898762549E-18 ) ) ;
#13419=EDGE_CURVE ( 'NONE', #2480, #7969, #8384, .T. ) ;
#13420=FACE_OUTER_BOUND ( 'NONE', #9278, .T. ) ;
#13421=CARTESIAN_POINT ( 'NONE',  ( -8.385254915620292238, 5.904668890677671200, -1.047751159211637166E-15 ) ) ;
#13424=CARTESIAN_POINT ( 'NONE',  ( 12.99553232110414136, 20.49953269456136695, 3.182987412051232168E-15 ) ) ;
#13425=LINE ( 'NONE', #5956, #7346 ) ;
#13426=ORIENTED_EDGE ( 'NONE', *, *, #11073, .T. ) ;
#13428=CARTESIAN_POINT ( 'NONE',  ( -10.69346802281034137, -25.79937747632526879, -21.38693604562069339 ) ) ;
#13430=EDGE_CURVE ( 'NONE', #6441, #8344, #2003, .T. ) ;
#13432=CARTESIAN_POINT ( 'NONE',  ( 12.99553232110414491, -36.04913500549519512, -25.99106464220827561 ) ) ;
#13433=CARTESIAN_POINT ( 'NONE',  ( 8.385254915620294014, 78.67828027274755698, 2.053795118489801188E-15 ) ) ;
#13434=EDGE_CURVE ( 'NONE', #6545, #11738, #10914, .T. ) ;
#13435=CARTESIAN_POINT ( 'NONE',  ( -2.008006351130390499, -80.00378950643924725, -9.910921267331605833 ) ) ;
#13437=CARTESIAN_POINT ( 'NONE',  ( -5.411086257474907235, -112.3214038155523298, 2.930518103359322168 ) ) ;
#13438=CARTESIAN_POINT ( 'NONE',  ( -10.69346802281034492, 49.59884612375012836, -21.38693604562069694 ) ) ;
#13439=ORIENTED_EDGE ( 'NONE', *, *, #2967, .F. ) ;
#13441=CARTESIAN_POINT ( 'NONE',  ( 10.69346802281034847, -6.949821576306441706, 2.619144277183853949E-15 ) ) ;
#13442=CARTESIAN_POINT ( 'NONE',  ( 8.385254915620294014, 90.00000000000000000, 8.679704431140118580E-16 ) ) ;
#13443=CIRCLE ( 'NONE', #11818, 2.000000000000003109 ) ;
#13444=EDGE_CURVE ( 'NONE', #7271, #2160, #6835, .T. ) ;
#13445=FACE_OUTER_BOUND ( 'NONE', #7283, .T. ) ;
#13447=CARTESIAN_POINT ( 'NONE',  ( 7.861734798228629195, -72.85454079061371147, 6.394819286084763910 ) ) ;
#13451=CARTESIAN_POINT ( 'NONE',  ( -10.69346802281034137, -16.37459952631584059, -21.38693604562069339 ) ) ;
#13452=CARTESIAN_POINT ( 'NONE',  ( -0.3134609018057502028, -154.2164502158701964, 0.8036717672344616537 ) ) ;
#13453=EDGE_CURVE ( 'NONE', #1727, #1229, #11944, .T. ) ;
#13455=CARTESIAN_POINT ( 'NONE',  ( 25.00000000000000355, 120.0000000000000284, 0.5000000000000000000 ) ) ;
#13458=ORIENTED_EDGE ( 'NONE', *, *, #8833, .F. ) ;
#13462=EDGE_CURVE ( 'NONE', #3489, #10825, #8832, .T. ) ;
#13463=VERTEX_POINT ( 'NONE', #13171 ) ;
#13464=CARTESIAN_POINT ( 'NONE',  ( 2.124423463547386426, -120.2384439167012005, 4.721629364818086927 ) ) ;
#13471=CARTESIAN_POINT ( 'NONE',  ( 3.571252647454290496, -130.5986068350643166, -1.733046011458916791 ) ) ;
#13473=CARTESIAN_POINT ( 'NONE',  ( 10.00000000000000000, 92.00000000000000000, -2.500000000000000000 ) ) ;
#13476=CIRCLE ( 'NONE', #7366, 15.29705854078139105 ) ;
#13481=CARTESIAN_POINT ( 'NONE',  ( -8.385254915620292238, 53.02855864072483882, -2.186455329360211015E-15 ) ) ;
#13482=CIRCLE ( 'NONE', #3124, 8.385254915620290461 ) ;
#13484=CARTESIAN_POINT ( 'NONE',  ( -5.849706340270382832, -65.63636363291594478, -2.546235460503720294 ) ) ;
#13487=EDGE_LOOP ( 'NONE', ( #5815, #3520, #12865, #1826 ) ) ;
#13488=CARTESIAN_POINT ( 'NONE',  ( 8.207015671355002297E-16, -29.33764382806072746, 5.180607919632063331E-17 ) ) ;
#13490=CARTESIAN_POINT ( 'NONE',  ( -10.69381717166375623, 34.98422482212468054, -2.696393829553742293E-15 ) ) ;
#13497=CARTESIAN_POINT ( 'NONE',  ( -35.20000000000000995, 106.4000000000000199, -0.5000000000000000000 ) ) ;
#13500=ORIENTED_EDGE ( 'NONE', *, *, #11820, .T. ) ;
#13501=CIRCLE ( 'NONE', #4258, 5.000000000000000000 ) ;
#13502=( BOUNDED_SURFACE ( )  B_SPLINE_SURFACE ( 3, 3, ( 
 ( #11548, #1943, #6290, #3121 ),
 ( #6228, #3977, #12473, #964 ),
 ( #8254, #10492, #12545, #2928 ),
 ( #7200, #5227, #894, #11480 ) ),
 .UNSPECIFIED., .F., .F., .F. ) 
 B_SPLINE_SURFACE_WITH_KNOTS ( ( 4, 4 ),
 ( 4, 4 ),
 ( 0.000000000000000000, 1.000000000000000000 ),
 ( 0.000000000000000000, 1.000000000000000000 ),
 .UNSPECIFIED. ) 
 GEOMETRIC_REPRESENTATION_ITEM ( )  RATIONAL_B_SPLINE_SURFACE ( (
 ( 1.000000000000000000, 0.3333333333333334259, 0.3333333333333334259, 1.000000000000000000),
 ( 1.000000000000000000, 0.3333333333333334259, 0.3333333333333334259, 1.000000000000000000),
 ( 1.000000000000000000, 0.3333333333333334259, 0.3333333333333334259, 1.000000000000000000),
 ( 1.000000000000000000, 0.3333333333333334259, 0.3333333333333334259, 1.000000000000000000) ) ) 
 REPRESENTATION_ITEM ( '' )  SURFACE ( )  );
#13505=CARTESIAN_POINT ( 'NONE',  ( -12.99553232110414136, -36.04913500549519512, -3.146276702057636506E-15 ) ) ;
#13506=CARTESIAN_POINT ( 'NONE',  ( -12.99553232110414491, 77.04820039461787928, 25.99106464220826851 ) ) ;
#13508=DIRECTION ( 'NONE',  ( -1.000000000000000000, 0.000000000000000000, 0.000000000000000000 ) ) ;
#13509=CARTESIAN_POINT ( 'NONE',  ( 0.6389323985104377046, -103.7399573628443932, 7.199555016268553764 ) ) ;
#13511=CARTESIAN_POINT ( 'NONE',  ( 8.385254915620297567, -31.79444290936001494, -16.77050983124058448 ) ) ;
#13512=ORIENTED_EDGE ( 'NONE', *, *, #10470, .F. ) ;
#13514=EDGE_CURVE ( 'NONE', #5587, #6577, #2727, .T. ) ;
#13516=VERTEX_POINT ( 'NONE', #3598 ) ;
#13520=ORIENTED_EDGE ( 'NONE', *, *, #7551, .T. ) ;
#13524=CARTESIAN_POINT ( 'NONE',  ( 9.661733385268016505, -70.21865067213146006, 3.001891211723641373 ) ) ;
#13526=CARTESIAN_POINT ( 'NONE',  ( -12.99579180576516713, 45.23395377697384134, -1.751278857619846450E-15 ) ) ;
#13527=CARTESIAN_POINT ( 'NONE',  ( 3.039669588831058533, -137.4545454546045846, -0.1626128505627332244 ) ) ;
#13529=CARTESIAN_POINT ( 'NONE',  ( -2.517691654963332357E-15, 90.00000000000000000, -1.589271161308885878E-16 ) ) ;
#13531=ORIENTED_EDGE ( 'NONE', *, *, #5159, .F. ) ;
#13533=CARTESIAN_POINT ( 'NONE',  ( 2.442259928100406263, -119.8068162713657898, 4.626198433201162530 ) ) ;
#13535=CARTESIAN_POINT ( 'NONE',  ( 15.29705854078138927, 90.00000000000000000, 1.714422261702872766E-15 ) ) ;
#13538=CARTESIAN_POINT ( 'NONE',  ( -0.1421958018836135540, -122.9182064327156212, -4.881833328960847318 ) ) ;
#13539=CARTESIAN_POINT ( 'NONE',  ( -0.9182679296299821603, -168.0000000000001421, -0.7188769083877089017 ) ) ;
#13540=CARTESIAN_POINT ( 'NONE',  ( 10.00000000000000000, 97.99999999999994316, 2.500000000000000000 ) ) ;
#13543=DIRECTION ( 'NONE',  ( 0.000000000000000000, 0.000000000000000000, 1.000000000000000000 ) ) ;
#13546=ORIENTED_EDGE ( 'NONE', *, *, #13218, .T. ) ;
#13548=CARTESIAN_POINT ( 'NONE',  ( 15.29705854078138394, 38.52236939141059935, 1.806990092252540040E-15 ) ) ;
#13549=CARTESIAN_POINT ( 'NONE',  ( -3.794964386186622907, -129.7272727272728901, 2.624161884220013619 ) ) ;
#13550=CIRCLE ( 'NONE', #1630, 15.29705854078139460 ) ;
#13553=ORIENTED_EDGE ( 'NONE', *, *, #8327, .T. ) ;
#13554=CARTESIAN_POINT ( 'NONE',  ( -4.895853646792291514, 90.06529264441493865, -1.023585852534433460 ) ) ;
#13555=DIRECTION ( 'NONE',  ( 0.000000000000000000, 0.000000000000000000, 1.000000000000000000 ) ) ;
#13556=CARTESIAN_POINT ( 'NONE',  ( 8.385254915620290461, 34.17900274070598243, 9.905219695108648343E-16 ) ) ;
#13558=FACE_OUTER_BOUND ( 'NONE', #5733, .T. ) ;
#13559=CARTESIAN_POINT ( 'NONE',  ( -15.29705854078139105, 19.67281349139177138, -1.942828122597488220E-15 ) ) ;
#13560=CARTESIAN_POINT ( 'NONE',  ( -2.517691654963332357E-15, 90.00000000000000000, -1.589271161308885878E-16 ) ) ;
#13565=CARTESIAN_POINT ( 'NONE',  ( 10.69381717166375800, -21.56444287793185666, 1.362947136962396926E-15 ) ) ;
#13566=EDGE_CURVE ( 'NONE', #2716, #9777, #407, .T. ) ;
#13569=CARTESIAN_POINT ( 'NONE',  ( -8.385254915620288685, -3.520109059331755663, -16.77050983124058448 ) ) ;
#13570=DIRECTION ( 'NONE',  ( 0.000000000000000000, 0.000000000000000000, -1.000000000000000000 ) ) ;
#13571=CARTESIAN_POINT ( 'NONE',  ( 8.320762423101355054, -90.25487416876752889, -3.125163722747064110 ) ) ;
#13573=ORIENTED_EDGE ( 'NONE', *, *, #6356, .F. ) ;
#13574=EDGE_LOOP ( 'NONE', ( #10132, #1676, #395, #12120 ) ) ;
#13576=CIRCLE ( 'NONE', #2334, 8.385254915620294014 ) ;
#13577=ORIENTED_EDGE ( 'NONE', *, *, #3110, .F. ) ;
#13582=LINE ( 'NONE', #3024, #11497 ) ;
#13583=EDGE_CURVE ( 'NONE', #1929, #7574, #3688, .T. ) ;
#13586=DIRECTION ( 'NONE',  ( -1.000000000000000000, 0.000000000000000000, 0.000000000000000000 ) ) ;
#13587=DIRECTION ( 'NONE',  ( 1.000000000000000000, 0.000000000000000000, 0.000000000000000000 ) ) ;
#13588=CARTESIAN_POINT ( 'NONE',  ( -2.035923840464202161, -145.3956134166558058, -1.226378594624949026 ) ) ;
#13589=EDGE_CURVE ( 'NONE', #12324, #2480, #7054, .T. ) ;
#13590=PLANE ( 'NONE',  #10855 ) ;
#13591=AXIS2_PLACEMENT_3D ( 'NONE', #232, #1270, #5474 ) ;
#13592=EDGE_CURVE ( 'NONE', #3902, #2799, #12016, .T. ) ;
#13595=AXIS2_PLACEMENT_3D ( 'NONE', #9222, #3747, #9084 ) ;
#13597=CARTESIAN_POINT ( 'NONE',  ( 5.850599514082611030, -109.0563038876532573, -2.972233473650054858 ) ) ;
#13598=DIRECTION ( 'NONE',  ( -1.000000000000000000, 0.000000000000000000, 0.000000000000000000 ) ) ;
#13599=DIRECTION ( 'NONE',  ( -1.000000000000000000, 0.000000000000000000, 0.000000000000000000 ) ) ;
#13600=AXIS2_PLACEMENT_3D ( 'NONE', #310, #529, #1487 ) ;
#13602=CARTESIAN_POINT ( 'NONE',  ( -1.135377999189010501, -155.8397449083613822, -1.102628456091256703 ) ) ;
#13604=CARTESIAN_POINT ( 'NONE',  ( -0.5095487865723351550, -163.8787878240969746, -3.239446892380866583 ) ) ;
#13607=ADVANCED_FACE ( 'NONE', ( #12386 ), #9965, .T. ) ;
#13608=CARTESIAN_POINT ( 'NONE',  ( 15.29705854078138927, 19.67281349139177138, 1.840275709580740132E-15 ) ) ;
#13609=AXIS2_PLACEMENT_3D ( 'NONE', #3222, #7500, #4204 ) ;
#13613=DIRECTION ( 'NONE',  ( -0.000000000000000000, -0.000000000000000000, -1.000000000000000000 ) ) ;
#13614=EDGE_CURVE ( 'NONE', #8762, #1146, #4824, .T. ) ;
#13616=CARTESIAN_POINT ( 'NONE',  ( 10.00000000000000711, 139.9999999999999716, 0.5000000000000000000 ) ) ;
#13618=DIRECTION ( 'NONE',  ( 1.000000000000000000, 0.000000000000000000, 0.000000000000000000 ) ) ;
#13620=CARTESIAN_POINT ( 'NONE',  ( 6.295302227001586814, -164.3636363559542701, -1.035156591622384159 ) ) ;
#13623=ORIENTED_EDGE ( 'NONE', *, *, #12917, .T. ) ;
#13624=DIRECTION ( 'NONE',  ( 5.551115123125776539E-17, -1.000000000000000000, -3.204747427460360459E-31 ) ) ;
#13625=DIRECTION ( 'NONE',  ( 0.000000000000000000, 0.000000000000000000, -1.000000000000000000 ) ) ;
#13627=AXIS2_PLACEMENT_3D ( 'NONE', #4975, #9254, #13570 ) ;
#13628=CARTESIAN_POINT ( 'NONE',  ( 15.29705854078139282, -8.601520358636511432, 1.890204135573039875E-15 ) ) ;
#13629=LINE ( 'NONE', #1874, #10007 ) ;
#13631=DIRECTION ( 'NONE',  ( -0.000000000000000000, -0.000000000000000000, -1.000000000000000000 ) ) ;
#13636=EDGE_LOOP ( 'NONE', ( #12831, #2393, #3738, #9910 ) ) ;
#13640=FACE_OUTER_BOUND ( 'NONE', #6962, .T. ) ;
#13642=CARTESIAN_POINT ( 'NONE',  ( 2.981500127671308675, -138.8769926725574635, -0.6020624928271046672 ) ) ;
#13643=FACE_OUTER_BOUND ( 'NONE', #9909, .T. ) ;
#13649=ORIENTED_EDGE ( 'NONE', *, *, #6433, .F. ) ;
#13650=CARTESIAN_POINT ( 'NONE',  ( 9.637068721888157441, -69.33333333333251858, 3.199157287630882252 ) ) ;
#13653=CARTESIAN_POINT ( 'NONE',  ( -4.278103086406176203, -97.41991341992381592, -7.774081346650261182 ) ) ;
#13654=DIRECTION ( 'NONE',  ( -2.797435172181481150E-17, 1.000000000000000000, -1.765856845898762549E-18 ) ) ;
#13656=FACE_OUTER_BOUND ( 'NONE', #10296, .T. ) ;
#13657=CARTESIAN_POINT ( 'NONE',  ( 3.202161775521378484, -122.5503334129114279, 3.775223943724925313 ) ) ;
#13660=DIRECTION ( 'NONE',  ( -2.797435172181481150E-17, 1.000000000000000000, -1.765856845898762549E-18 ) ) ;
#13661=ORIENTED_EDGE ( 'NONE', *, *, #8308, .T. ) ;
#13664=EDGE_CURVE ( 'NONE', #12240, #3719, #9075, .T. ) ;
#13665=CIRCLE ( 'NONE', #7780, 2.000000000000000000 ) ;
#13668=EDGE_LOOP ( 'NONE', ( #10030, #11171, #8244, #5596 ) ) ;
#13669=CARTESIAN_POINT ( 'NONE',  ( -15.29705854078138749, 38.52236939141059935, -3.816389449506426866E-15 ) ) ;
#13670=CARTESIAN_POINT ( 'NONE',  ( 8.869476657224877769, -90.43147964619883794, 0.05619714888382777024 ) ) ;
#13671=CARTESIAN_POINT ( 'NONE',  ( -0.2677229415630820730, -160.9696969673928209, 0.7106593571390205089 ) ) ;
#13679=DIRECTION ( 'NONE',  ( 1.000000000000000000, 0.000000000000000000, 0.000000000000000000 ) ) ;
#13680=ADVANCED_FACE ( 'NONE', ( #1572 ), #3239, .T. ) ;
#13683=CARTESIAN_POINT ( 'NONE',  ( 3.361332843921851943, -147.1038961038433968, 14.17852599539457259 ) ) ;
#13685=VERTEX_POINT ( 'NONE', #8103 ) ;
#13686=B_SPLINE_CURVE_WITH_KNOTS ( 'NONE', 3,
 ( #1716, #9287, #3888, #546, #4871, #2632, #10342, #12387, #13602, #13322, #6978, #6898, #12518, #471, #11187, #7109, #743, #11458, #2902, #3673, #4808, #10060, #10203, #5008, #5864, #9015, #7957, #9086, #10137, #9149, #13402, #2703, #11259, #1649, #5932, #2774, #13471, #3816, #8104, #7041, #6002, #10267, #670, #4940, #9223, #13538, #8167, #7441, #10668, #8498, #3232, #2054, #7511, #1849, #11659, #6331, #1983, #7371, #11723, #5205, #12725, #12868, #4083, #6136, #4017, #10406, #10603, #6264, #9560, #2113, #6400, #9493, #9358, #1006, #4152, #942, #10467, #13740, #807, #10535, #6207, #1076, #870, #7242, #3041, #8564, #13802, #5275, #3166, #5077, #13869, #8436, #13670, #4216, #8367, #5340, #12794, #9624, #32, #5138, #3101, #4285, #9426, #8300, #12594, #2973, #11525, #1918, #12660, #7310, #11594, #1149, #11857, #3298 ),
 .UNSPECIFIED., .F., .F.,
 ( 4, 2, 2, 2, 2, 2, 2, 2, 2, 2, 2, 2, 2, 2, 2, 2, 2, 2, 2, 2, 2, 2, 2, 2, 2, 2, 2, 2, 2, 2, 2, 2, 2, 2, 2, 2, 2, 2, 2, 2, 2, 2, 2, 2, 2, 2, 2, 2, 2, 2, 2, 2, 2, 2, 2, 2, 4 ),
 ( 2.168404344971008868E-19, 0.0008229045663924312816, 0.001645809132784862346, 0.003291618265569724693, 0.004937427398354586605, 0.006583236531139448518, 0.009874854796709173210, 0.01152066392949403426, 0.01316647306227889704, 0.01481228219506375982, 0.01645809132784862086, 0.01974970959341826662, 0.02139551872620305134, 0.02304132785898783606, 0.02633294612455740549, 0.02797875525734215552, 0.02962456439012690901, 0.03127037352291166250, 0.03291618265569640905, 0.03620780092126597849, 0.03785361005405073198, 0.03949941918683547853, 0.04114522831962022509, 0.04279103745240498552, 0.04608265571797444393, 0.04772846485075918355, 0.04937427398354391622, 0.05102008311632864890, 0.05184298768272101871, 0.05266589224911337463, 0.05595751051468290937, 0.05924912878025244412, 0.06089493791303720455, 0.06254074704582197886, 0.06418655617860674623, 0.06583236531139149972, 0.06912398357696107609, 0.07076979270974584346, 0.07241560184253061083, 0.07406141097531537820, 0.07570722010810014557, 0.07899883837366970807, 0.08064464750645450319, 0.08229045663923928444, 0.08393626577202409345, 0.08558207490480887469, 0.08887369317037849270, 0.09051950230316328783, 0.09216531143594809683, 0.09381112056873290583, 0.09545692970151771484, 0.09710273883430250996, 0.09874854796708731897, 0.1020401662326569370, 0.1036859753654417460, 0.1045088799318341505, 0.1053317844982265411 ),
 .UNSPECIFIED. ) ;
#13687=CYLINDRICAL_SURFACE ( 'NONE', #4576, 8.385254915620292238 ) ;
#13691=CARTESIAN_POINT ( 'NONE',  ( -9.637068721888248035, -69.33333333333280279, -3.199157287630891133 ) ) ;
#13693=DIRECTION ( 'NONE',  ( -2.797435172181481150E-17, 1.000000000000000000, -1.765856845898762549E-18 ) ) ;
#13695=CARTESIAN_POINT ( 'NONE',  ( 5.912741558351815918, -73.45454546935906137, 18.82838426099241858 ) ) ;
#13696=CARTESIAN_POINT ( 'NONE',  ( 19.28867028138563811, -167.3636363504097346, -6.559046149895597644 ) ) ;
#13698=CARTESIAN_POINT ( 'NONE',  ( -8.385254915620292238, -22.36966495935058319, -9.478943072270380731E-16 ) ) ;
#13699=DIRECTION ( 'NONE',  ( -2.797435172181481150E-17, 1.000000000000000000, -1.765856845898762549E-18 ) ) ;
#13701=CARTESIAN_POINT ( 'NONE',  ( 0.6173387890061948768, -70.00000000000000000, -4.961742921553712549 ) ) ;
#13706=ORIENTED_EDGE ( 'NONE', *, *, #2999, .F. ) ;
#13711=FACE_OUTER_BOUND ( 'NONE', #11868, .T. ) ;
#13713=CARTESIAN_POINT ( 'NONE',  ( 0.03718945268892032141, -157.3606764272614669, 1.516196336863006477 ) ) ;
#13715=VECTOR ( 'NONE', #6052, 1000.000000000000000 ) ;
#13719=VERTEX_POINT ( 'NONE', #11457 ) ;
#13720=CYLINDRICAL_SURFACE ( 'NONE', #13798, 2.000000000000001776 ) ;
#13722=CARTESIAN_POINT ( 'NONE',  ( 15.29705854078139282, -38.76242177807012723, 1.940132561565339619E-15 ) ) ;
#13730=CARTESIAN_POINT ( 'NONE',  ( -0.3891315833696432636, -154.2086256632273944, -1.618697729122736018 ) ) ;
#13737=CARTESIAN_POINT ( 'NONE',  ( -12.99553232110413781, 39.34908859458022334, -1.730463420974848368E-15 ) ) ;
#13738=CARTESIAN_POINT ( 'NONE',  ( 1.236368069360658017, -80.00117829049393947, 9.950313871619497874 ) ) ;
#13740=CARTESIAN_POINT ( 'NONE',  ( 1.581460637658297141, -99.95560608173282446, 7.500979497773645477 ) ) ;
#13741=CARTESIAN_POINT ( 'NONE',  ( -15.29705854078139637, 64.91013567203349055, -3.859655058983359639E-15 ) ) ;
#13742=FACE_OUTER_BOUND ( 'NONE', #1964, .T. ) ;
#13743=CARTESIAN_POINT ( 'NONE',  ( 10.69346802281034847, 2.474956373702985601, 1.309720302413869460E-15 ) ) ;
#13747=ORIENTED_EDGE ( 'NONE', *, *, #11002, .F. ) ;
#13749=DIRECTION ( 'NONE',  ( 1.000000000000000000, 0.000000000000000000, 0.000000000000000000 ) ) ;
#13750=CARTESIAN_POINT ( 'NONE',  ( -1.916816365364703234, -124.8181818181863747, -4.196942880910714990 ) ) ;
#13755=FACE_OUTER_BOUND ( 'NONE', #11267, .T. ) ;
#13757=CARTESIAN_POINT ( 'NONE',  ( -6.075667645225103719, -100.2727272727262147, -11.56208117637899058 ) ) ;
#13758=EDGE_CURVE ( 'NONE', #11837, #11393, #6591, .T. ) ;
#13762=CARTESIAN_POINT ( 'NONE',  ( 35.20000000000001705, 106.4000000000000199, -0.5000000000000000000 ) ) ;
#13768=AXIS2_PLACEMENT_3D ( 'NONE', #11550, #7331, #5230 ) ;
#13774=DIRECTION ( 'NONE',  ( -1.000000000000000000, 0.000000000000000000, 0.000000000000000000 ) ) ;
#13775=DIRECTION ( 'NONE',  ( 0.000000000000000000, 0.000000000000000000, 1.000000000000000000 ) ) ;
#13778=ORIENTED_EDGE ( 'NONE', *, *, #7707, .F. ) ;
#13779=VERTEX_POINT ( 'NONE', #2180 ) ;
#13780=CARTESIAN_POINT ( 'NONE',  ( -2.179449471770338320, 90.00000000000000000, -4.500000000000000888 ) ) ;
#13784=ORIENTED_EDGE ( 'NONE', *, *, #6628, .F. ) ;
#13785=CARTESIAN_POINT ( 'NONE',  ( 10.69381717166375623, 6.709890972096427042, 0.000000000000000000 ) ) ;
#13789=CARTESIAN_POINT ( 'NONE',  ( -2.517691654963332357E-15, 90.00000000000000000, -1.589271161308885878E-16 ) ) ;
#13790=CARTESIAN_POINT ( 'NONE',  ( -8.385254915620295790, 69.25350232273815720, -2.234634242108977241E-15 ) ) ;
#13791=CARTESIAN_POINT ( 'NONE',  ( 0.8868958219609875959, -105.3243828844967851, -6.976889881733200127 ) ) ;
#13792=CARTESIAN_POINT ( 'NONE',  ( -25.00000000000000355, 120.0000000000000284, 2.500000000000000000 ) ) ;
#13793=EDGE_LOOP ( 'NONE', ( #1454, #2404, #1825, #10742 ) ) ;
#13796=DIRECTION ( 'NONE',  ( -1.000000000000000000, 0.000000000000000000, 0.000000000000000000 ) ) ;
#13798=AXIS2_PLACEMENT_3D ( 'NONE', #3018, #4065, #11570 ) ;
#13801=DIRECTION ( 'NONE',  ( -1.000000000000000000, 0.000000000000000000, 0.000000000000000000 ) ) ;
#13802=CARTESIAN_POINT ( 'NONE',  ( 7.157689724239170381, -94.21585681134573065, 4.329420255253605632 ) ) ;
#13805=CARTESIAN_POINT ( 'NONE',  ( -10.69381717166375090, 63.25855867215300066, -21.38763434332750890 ) ) ;
#13806=AXIS2_PLACEMENT_3D ( 'NONE', #12740, #5221, #4168 ) ;
#13807=CARTESIAN_POINT ( 'NONE',  ( -12.99553232110414314, 20.49953269456136695, -3.227288338581441853E-15 ) ) ;
#13808=CARTESIAN_POINT ( 'NONE',  ( -8.385254915620294014, 3.280056672672170937, -2.065495521823092020E-15 ) ) ;
#13813=CARTESIAN_POINT ( 'NONE',  ( 12.65441377644658338, -89.44155844155163493, -5.520840484228896727 ) ) ;
#13817=CARTESIAN_POINT ( 'NONE',  ( -12.99579180576516890, -11.31471392308272605, -1.551565153650648068E-15 ) ) ;
#13822=CARTESIAN_POINT ( 'NONE',  ( 10.35394582475457348, -71.99999999999978684, 3.762420212848049506 ) ) ;
#13823=CARTESIAN_POINT ( 'NONE',  ( -0.1916457366473549029, -105.1818181818147764, -4.609965990740172437 ) ) ;
#13824=CARTESIAN_POINT ( 'NONE',  ( 10.00000000000000711, 139.9999999999999716, -0.5000000000000000000 ) ) ;
#13826=AXIS2_PLACEMENT_3D ( 'NONE', #6895, #11181, #5858 ) ;
#13830=ORIENTED_EDGE ( 'NONE', *, *, #12441, .F. ) ;
#13832=EDGE_CURVE ( 'NONE', #1419, #7777, #13372, .T. ) ;
#13835=ORIENTED_EDGE ( 'NONE', *, *, #11890, .T. ) ;
#13836=EDGE_CURVE ( 'NONE', #9187, #6329, #810, .T. ) ;
#13837=CARTESIAN_POINT ( 'NONE',  ( 15.29705854078140170, -19.91286587805129926, 1.949638918210574015E-15 ) ) ;
#13838=CARTESIAN_POINT ( 'NONE',  ( -10.69346802281034847, 68.44840202376897764, -1.551312297200932909E-15 ) ) ;
#13840=CARTESIAN_POINT ( 'NONE',  ( -10.09953664725343003, -70.24026703750095635, -0.01926284172907780090 ) ) ;
#13841=CARTESIAN_POINT ( 'NONE',  ( -0.1430943862779323617, -159.4721208788122340, 1.503668078069826608 ) ) ;
#13843=LINE ( 'NONE', #6307, #8933 ) ;
#13846=ADVANCED_FACE ( 'NONE', ( #6263 ), #1005, .T. ) ;
#13847=CARTESIAN_POINT ( 'NONE',  ( -4.268720428656457067, 91.34229515271626099, -2.603909174561179540 ) ) ;
#13848=CARTESIAN_POINT ( 'NONE',  ( 3.188279143310706054, -76.81818181818272251, 9.710576830322445119 ) ) ;
#13849=ORIENTED_EDGE ( 'NONE', *, *, #4887, .T. ) ;
#13850=ADVANCED_FACE ( 'NONE', ( #5274 ), #1822, .T. ) ;
#13852=EDGE_CURVE ( 'NONE', #1727, #2504, #8848, .T. ) ;
#13853=FACE_OUTER_BOUND ( 'NONE', #6565, .T. ) ;
#13854=( BOUNDED_SURFACE ( )  B_SPLINE_SURFACE ( 3, 3, ( 
 ( #2911, #9499, #7182, #5014 ),
 ( #4222, #9296, #5085, #3107 ),
 ( #8237, #3175, #9366, #11464 ),
 ( #7381, #5145, #1854, #6144 ) ),
 .UNSPECIFIED., .F., .F., .F. ) 
 B_SPLINE_SURFACE_WITH_KNOTS ( ( 4, 4 ),
 ( 4, 4 ),
 ( 0.000000000000000000, 1.000000000000000000 ),
 ( 0.000000000000000000, 1.000000000000000000 ),
 .UNSPECIFIED. ) 
 GEOMETRIC_REPRESENTATION_ITEM ( )  RATIONAL_B_SPLINE_SURFACE ( (
 ( 1.000000000000000000, 0.3333333333333334259, 0.3333333333333334259, 1.000000000000000000),
 ( 1.000000000000000000, 0.3333333333333334259, 0.3333333333333334259, 1.000000000000000000),
 ( 1.000000000000000000, 0.3333333333333334259, 0.3333333333333334259, 1.000000000000000000),
 ( 1.000000000000000000, 0.3333333333333334259, 0.3333333333333334259, 1.000000000000000000) ) ) 
 REPRESENTATION_ITEM ( '' )  SURFACE ( )  );
#13858=CARTESIAN_POINT ( 'NONE',  ( 2.869852970730162767, -107.6167546509799706, -6.080253893975354096 ) ) ;
#13861=ORIENTED_EDGE ( 'NONE', *, *, #13583, .F. ) ;
#13864=CARTESIAN_POINT ( 'NONE',  ( 1.571852504498140624, -148.1710643681929866, -1.425705211460633670 ) ) ;
#13865=EDGE_CURVE ( 'NONE', #13042, #13685, #9314, .T. ) ;
#13866=CARTESIAN_POINT ( 'NONE',  ( -8.385254915620295790, 40.97916847270985130, -1.171624249618447227E-15 ) ) ;
#13867=VERTEX_POINT ( 'NONE', #869 ) ;
#13868=CARTESIAN_POINT ( 'NONE',  ( -10.69346802281034137, 40.17406817374067174, -21.38693604562068984 ) ) ;
#13869=CARTESIAN_POINT ( 'NONE',  ( 8.374988411100524388, -92.13370500812025909, 2.112857200571143235 ) ) ;
#13871=CARTESIAN_POINT ( 'NONE',  ( -0.05313321603431308410, -142.5800865801647319, -3.258060136337923129 ) ) ;
#13874=CARTESIAN_POINT ( 'NONE',  ( -8.599520226296840875, -74.45454545454605011, -5.474475378420836869 ) ) ;
#13880=CARTESIAN_POINT ( 'NONE',  ( -2.224981447605033136, -153.6493506492698771, 4.266231359686146973 ) ) ;
#13882=CARTESIAN_POINT ( 'NONE',  ( 12.99579180576516180, -11.31471392308272428, 25.99158361153033425 ) ) ;
#13884=CARTESIAN_POINT ( 'NONE',  ( 0.000000000000000000, 71.01020514433645303, -0.5000000000000000000 ) ) ;
#13886=AXIS2_PLACEMENT_3D ( 'NONE', #1309, #4457, #6440 ) ;
#13887=CARTESIAN_POINT ( 'NONE',  ( -6.296481028167455030, -65.63636363759458447, -1.027962039461249866 ) ) ;
#13890=CARTESIAN_POINT ( 'NONE',  ( -10.69346802281033959, 11.89973432371241202, -21.38693604562068984 ) ) ;
#13891=CARTESIAN_POINT ( 'NONE',  ( -10.00000000000000000, 92.00000000000000000, 0.5000000000000000000 ) ) ;
#13894=CIRCLE ( 'NONE', #8476, 50.00000000000001421 ) ;
#13895=ORIENTED_EDGE ( 'NONE', *, *, #13252, .F. ) ;
#13897=ORIENTED_EDGE ( 'NONE', *, *, #5886, .T. ) ;
#13898=CARTESIAN_POINT ( 'NONE',  ( -2.517691654963332357E-15, 90.00000000000000000, -1.589271161308885878E-16 ) ) ;
ENDSEC;
END-ISO-10303-21;
